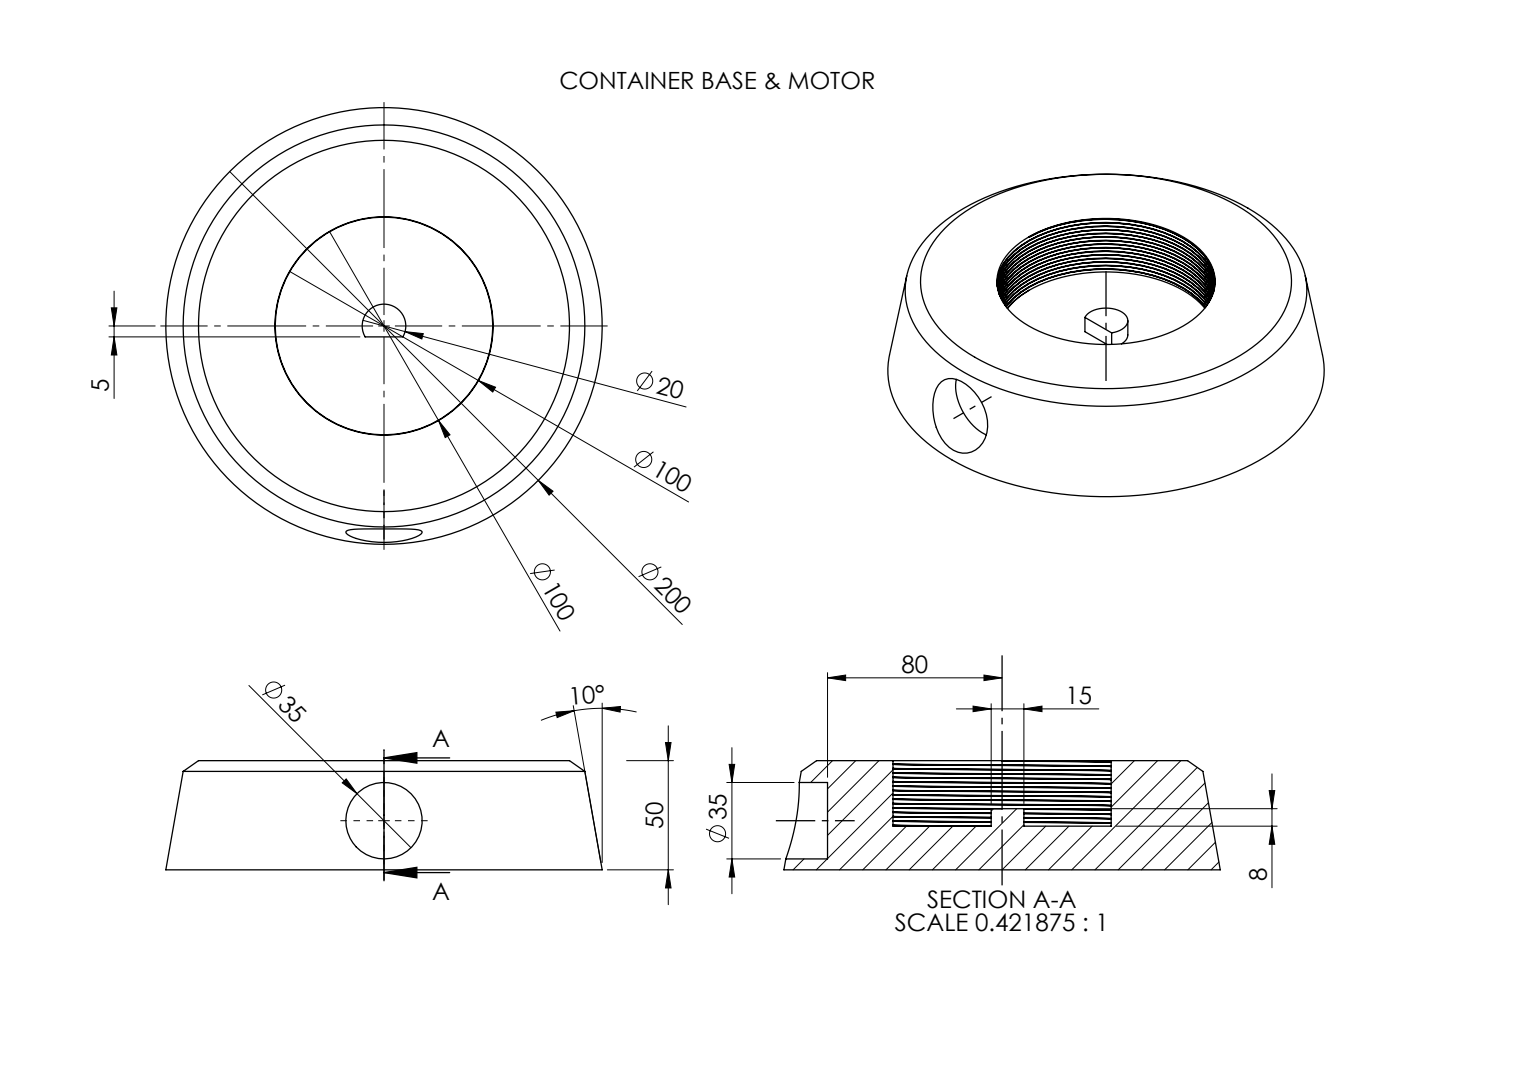
ISO-10303-21;
HEADER;
FILE_DESCRIPTION (('STEP AP214'),
    '1' );
FILE_NAME ('container base & motor.step',
    '2026-10-09T15:02:13',
    ( '' ),
    ( '' ),
    'SwSTEP 2.0',
    'SolidWorks 2026',
    '' );
FILE_SCHEMA (( 'AUTOMOTIVE_DESIGN' ));
ENDSEC;

DATA;
#6=DIRECTION ( 'NONE',  ( 0.000000000000000000, 0.000000000000000000, 1.000000000000000000 ) ) ;
#12=CARTESIAN_POINT ( 'NONE',  ( -15.40903463028480580, 24.25937500034139660, 47.42413220539094709 ) ) ;
#14=CARTESIAN_POINT ( 'NONE',  ( -49.86468353124999453, 37.82187500034139305, -16.20201782572375393 ) ) ;
#16=CARTESIAN_POINT ( 'NONE',  ( -3.219174618344376363E-15, 29.49999999999999645, -52.57311121191334990 ) ) ;
#17=CARTESIAN_POINT ( 'NONE',  ( 30.81806926056962936, 37.15937500034139873, -42.41743335407647209 ) ) ;
#19=CARTESIAN_POINT ( 'NONE',  ( 40.45084971874737079, 45.20000000000000284, -29.38926261462366440 ) ) ;
#27=CARTESIAN_POINT ( 'NONE',  ( -30.90169943749473447, 34.29999999999999005, 42.53254041760200721 ) ) ;
#31=CARTESIAN_POINT ( 'NONE',  ( 15.40903463028482356, 44.52187500034139589, 47.42413220539093999 ) ) ;
#32=CARTESIAN_POINT ( 'NONE',  ( -49.93234176562499727, 49.82031250051209526, 0.000000000000000000 ) ) ;
#34=CARTESIAN_POINT ( 'NONE',  ( -15.45084971874736368, 26.18125000068280173, 47.55282581475768211 ) ) ;
#36=CARTESIAN_POINT ( 'NONE',  ( -3.210462471511496205E-15, 31.42187500034139447, -52.43083105670540789 ) ) ;
#40=VERTEX_POINT ( 'NONE', #9811 ) ;
#45=CARTESIAN_POINT ( 'NONE',  ( -2.547328955960238000E-13, 24.28125000068279604, 49.99999999999999289 ) ) ;
#46=CARTESIAN_POINT ( 'NONE',  ( -3.210462471511496205E-15, 33.35937500034140157, -52.43083105670540789 ) ) ;
#48=CARTESIAN_POINT ( 'NONE',  ( 49.86468353125001585, 46.82187500034139305, 16.20201782572375038 ) ) ;
#63=CARTESIAN_POINT ( 'NONE',  ( 2.600676159226420495E-13, 33.28125000068279604, -49.99999999999999289 ) ) ;
#68=SURFACE_SIDE_STYLE ('',( #9066 ) ) ;
#69=CARTESIAN_POINT ( 'NONE',  ( -7.919222016226809657, 49.55125428154685352, -49.99999999999999289 ) ) ;
#70=CARTESIAN_POINT ( 'NONE',  ( -49.99999999999999289, 39.88125000068279746, 16.24598481164533226 ) ) ;
#73=EDGE_CURVE ( 'NONE', #16417, #15936, #15440, .T. ) ;
#74=CARTESIAN_POINT ( 'NONE',  ( 1.041190247313760726E-14, 50.00000000000000000, 85.01963570546854498 ) ) ;
#78=VECTOR ( 'NONE', #10957, 1000.000000000000000 ) ;
#82=CARTESIAN_POINT ( 'NONE',  ( 0.000000000000000000, 22.50000000000000000, 80.00000000000000000 ) ) ;
#83=CARTESIAN_POINT ( 'NONE',  ( -17.47289750917834539, 23.62647710751876318, 94.22769020256006911 ) ) ;
#89=CARTESIAN_POINT ( 'NONE',  ( 49.86468353125000164, 20.85937500034139802, -6.106662507704105588E-15 ) ) ;
#90=DIRECTION ( 'NONE',  ( -2.126576849575776229E-17, -0.9848077530122080203, -0.1736481776669307198 ) ) ;
#91=CARTESIAN_POINT ( 'NONE',  ( 30.81806926056962936, 27.22187500034139518, -42.41743335407646498 ) ) ;
#94=CARTESIAN_POINT ( 'NONE',  ( 30.90169943749474157, 29.30000000000000071, -42.53254041760200721 ) ) ;
#95=CARTESIAN_POINT ( 'NONE',  ( -49.86468353124999453, 35.95937500034139589, 16.20201782572377525 ) ) ;
#97=CARTESIAN_POINT ( 'NONE',  ( 49.99999999999999289, 41.10000000000000853, -16.24598481164532160 ) ) ;
#100=UNCERTAINTY_MEASURE_WITH_UNIT (LENGTH_MEASURE( 1.000000000000000082E-05 ), #13795, 'distance_accuracy_value', 'NONE');
#102=VERTEX_POINT ( 'NONE', #7719 ) ;
#108=CARTESIAN_POINT ( 'NONE',  ( -40.34137639590981195, 44.12187500034139731, 29.30972558990012189 ) ) ;
#109=CARTESIAN_POINT ( 'NONE',  ( -15.40903463028481646, 39.45937500034139589, -47.42413220539093999 ) ) ;
#113=CARTESIAN_POINT ( 'NONE',  ( -49.99999999999999289, 25.68125000068279462, -16.24598481164531449 ) ) ;
#114=CARTESIAN_POINT ( 'NONE',  ( 15.22000719008740077, 31.21383541804545914, 93.26445288283514401 ) ) ;
#116=CARTESIAN_POINT ( 'NONE',  ( 15.40903463028482356, 32.52187500034139589, 47.42413220539093999 ) ) ;
#122=CARTESIAN_POINT ( 'NONE',  ( -40.45084971874737789, 23.80000000000000071, -29.38926261462365730 ) ) ;
#124=CARTESIAN_POINT ( 'NONE',  ( 9.631387414534489405E-15, 34.35937500034139447, 52.43083105670540789 ) ) ;
#126=FACE_OUTER_BOUND ( 'NONE', #347, .T. ) ;
#128=CARTESIAN_POINT ( 'NONE',  ( 49.86468353125001585, 44.82187500034139305, 16.20201782572375038 ) ) ;
#132=DIRECTION ( 'NONE',  ( 0.000000000000000000, 0.000000000000000000, 1.000000000000000000 ) ) ;
#133=ORIENTED_EDGE ( 'NONE', *, *, #7031, .F. ) ;
#151=CIRCLE ( 'NONE', #2279, 50.00000000000000000 ) ;
#152=CARTESIAN_POINT ( 'NONE',  ( -30.90169943749473447, 32.08125000068280031, 42.53254041760200721 ) ) ;
#156=CARTESIAN_POINT ( 'NONE',  ( -30.90169943749474513, 49.70000000000000284, -42.53254041760200721 ) ) ;
#157=CARTESIAN_POINT ( 'NONE',  ( -40.45084971874737079, 41.98125000068279888, 29.38926261462367151 ) ) ;
#158=DIRECTION ( 'NONE',  ( -0.000000000000000000, 1.000000000000000000, -0.000000000000000000 ) ) ;
#159=EDGE_CURVE ( 'NONE', #15854, #13562, #284, .T. ) ;
#169=CARTESIAN_POINT ( 'NONE',  ( 49.99999999999999289, 42.88125000068279036, -16.24598481164532160 ) ) ;
#170=CARTESIAN_POINT ( 'NONE',  ( -1.240322475938754499E-13, 38.28125000068280315, 50.00000000000000000 ) ) ;
#173=CARTESIAN_POINT ( 'NONE',  ( 2.600676159226421000E-13, 31.49999999999999289, -49.99999999999999289 ) ) ;
#179=CARTESIAN_POINT ( 'NONE',  ( 15.40903463028482356, 24.45937500034139589, 47.42413220539093999 ) ) ;
#181=CARTESIAN_POINT ( 'NONE',  ( 49.86468353125000164, 28.92187500034139802, -6.106662507704105588E-15 ) ) ;
#183=CARTESIAN_POINT ( 'NONE',  ( 15.45084971874737789, 28.60000000000000142, 47.55282581475767500 ) ) ;
#184=CARTESIAN_POINT ( 'NONE',  ( 40.34137639590981905, 32.65937500034139873, 29.30972558990010768 ) ) ;
#192=( BOUNDED_CURVE ( )  B_SPLINE_CURVE ( 2, ( #6981, #12037, #4493, #8380, #732, #13454, #3955, #10196, #11517, #15248, #2623, #11683, #15338 ),
 .UNSPECIFIED., .F., .T. ) 
 B_SPLINE_CURVE_WITH_KNOTS ( ( 3, 2, 2, 2, 2, 2, 3 ),
 ( 0.4500000000000000111, 0.4533333333333333104, 0.4600000000000000200, 0.4666666666666666741, 0.4733333333333333282, 0.4799999999999999822, 0.4833333333333333370 ),
 .UNSPECIFIED. ) 
 CURVE ( )  GEOMETRIC_REPRESENTATION_ITEM ( )  RATIONAL_B_SPLINE_CURVE ( ( 0.9755282581475768211, 0.9755282581475770431, 1.000000000000000000, 0.9510565162951535312, 1.000000000000000000, 0.9510565162951535312, 1.000000000000000000, 0.9510565162951535312, 1.000000000000000000, 0.9510565162951535312, 1.000000000000000000, 0.9755282581475768211, 0.9755282581475768211 ) ) 
 REPRESENTATION_ITEM ( '' )  );
#196=CARTESIAN_POINT ( 'NONE',  ( 15.40903463028481113, 37.32187500034140015, -47.42413220539094709 ) ) ;
#197=CARTESIAN_POINT ( 'NONE',  ( 15.40903463028482356, 44.45937500034139589, 47.42413220539093999 ) ) ;
#198=DIRECTION ( 'NONE',  ( 0.8660254037844513642, 0.4999999999999780731, 0.000000000000000000 ) ) ;
#201=CARTESIAN_POINT ( 'NONE',  ( -15.45084971874736368, 20.18125000068279817, 47.55282581475768211 ) ) ;
#203=CARTESIAN_POINT ( 'NONE',  ( -49.86468353124999453, 28.02187500034139234, 16.20201782572377525 ) ) ;
#211=CARTESIAN_POINT ( 'NONE',  ( 49.99999999999999289, 48.88125000068280457, -16.24598481164532160 ) ) ;
#216=CARTESIAN_POINT ( 'NONE',  ( 49.86468353125000164, 30.85937500034139802, -6.106662507704105588E-15 ) ) ;
#217=CYLINDRICAL_SURFACE ( 'NONE', #11583, 50.00000000000000000 ) ;
#219=CARTESIAN_POINT ( 'NONE',  ( -49.86468353124999453, 47.82187500034140015, -16.20201782572375393 ) ) ;
#222=CARTESIAN_POINT ( 'NONE',  ( -40.34137639590981905, 47.72187500034139873, -29.30972558990011478 ) ) ;
#228=EDGE_LOOP ( 'NONE', ( #7013, #1311, #10553, #6194 ) ) ;
#232=CARTESIAN_POINT ( 'NONE',  ( -40.45084971874737789, 21.80000000000000071, -29.38926261462365730 ) ) ;
#234=CARTESIAN_POINT ( 'NONE',  ( -49.86468353125000164, 49.85937500034139447, 0.000000000000000000 ) ) ;
#237=CARTESIAN_POINT ( 'NONE',  ( -30.81806926056962226, 26.22187500034139518, 42.41743335407647919 ) ) ;
#239=CARTESIAN_POINT ( 'NONE',  ( -50.00000000000000000, 37.78125000068280315, 0.000000000000000000 ) ) ;
#248=DIRECTION ( 'NONE',  ( 0.000000000000000000, 0.000000000000000000, 1.000000000000000000 ) ) ;
#250=ORIENTED_EDGE ( 'NONE', *, *, #6640, .T. ) ;
#253=CARTESIAN_POINT ( 'NONE',  ( -13.94098003074309844, 33.14011566961073640, 93.12075586326798771 ) ) ;
#257=CARTESIAN_POINT ( 'NONE',  ( 40.34137639590981195, 21.05937500034139376, -29.30972558990011834 ) ) ;
#258=CARTESIAN_POINT ( 'NONE',  ( 6.123233995736766085E-15, 20.00000000000000355, -50.00000000000000000 ) ) ;
#259=CARTESIAN_POINT ( 'NONE',  ( 15.40903463028481113, 27.32187500034139660, -47.42413220539094709 ) ) ;
#261=CARTESIAN_POINT ( 'NONE',  ( 50.00000000000000711, 30.89999999999999503, 16.24598481164530739 ) ) ;
#262=CARTESIAN_POINT ( 'NONE',  ( 30.81806926056962936, 29.15937500034139518, -42.41743335407647209 ) ) ;
#275=CARTESIAN_POINT ( 'NONE',  ( -49.86468353124999453, 38.02187500034140299, 16.20201782572377525 ) ) ;
#276=CARTESIAN_POINT ( 'NONE',  ( -49.86468353125000164, 43.85937500034140157, 0.000000000000000000 ) ) ;
#279=CARTESIAN_POINT ( 'NONE',  ( -49.86468353124999453, 49.75937500034138594, -16.20201782572375393 ) ) ;
#280=CARTESIAN_POINT ( 'NONE',  ( 13.91912017332526830, 33.12251588586428852, 93.12580776402357685 ) ) ;
#282=CARTESIAN_POINT ( 'NONE',  ( 15.40903463028481113, 27.32187500034139660, -47.42413220539094709 ) ) ;
#284=( BOUNDED_CURVE ( )  B_SPLINE_CURVE ( 2, ( #4150, #13941, #12709, #1308, #6399, #11460, #5161, #10217, #15270, #3902, #8972, #5486, #15612 ),
 .UNSPECIFIED., .F., .T. ) 
 B_SPLINE_CURVE_WITH_KNOTS ( ( 3, 2, 2, 2, 2, 2, 3 ),
 ( 0.1166666666666666685, 0.1199999999999999956, 0.1266666666666666774, 0.1333333333333333315, 0.1400000000000000133, 0.1466666666666666674, 0.1499999999999999944 ),
 .UNSPECIFIED. ) 
 CURVE ( )  GEOMETRIC_REPRESENTATION_ITEM ( )  RATIONAL_B_SPLINE_CURVE ( ( 0.9755282581475768211, 0.9755282581475768211, 1.000000000000000000, 0.9510565162951535312, 1.000000000000000000, 0.9510565162951535312, 1.000000000000000000, 0.9510565162951535312, 1.000000000000000000, 0.9510565162951535312, 1.000000000000000000, 0.9755282581475768211, 0.9755282581475768211 ) ) 
 REPRESENTATION_ITEM ( '' )  );
#285=CARTESIAN_POINT ( 'NONE',  ( -30.90169943749474513, 27.70000000000000284, -42.53254041760200721 ) ) ;
#288=ORIENTED_EDGE ( 'NONE', *, *, #496, .T. ) ;
#293=CARTESIAN_POINT ( 'NONE',  ( -40.34137639590981195, 28.05937500034139731, 29.30972558990012189 ) ) ;
#294=EDGE_CURVE ( 'NONE', #4877, #10001, #5939, .T. ) ;
#297=CARTESIAN_POINT ( 'NONE',  ( 15.40903463028482356, 40.52187500034139589, 47.42413220539093999 ) ) ;
#300=CARTESIAN_POINT ( 'NONE',  ( 49.86468353125001585, 48.82187500034139305, 16.20201782572375038 ) ) ;
#308=CARTESIAN_POINT ( 'NONE',  ( -40.45084971874737789, 43.58125000068280031, -29.38926261462365730 ) ) ;
#311=CARTESIAN_POINT ( 'NONE',  ( 50.00000000000000711, 24.90000000000000213, 16.24598481164530739 ) ) ;
#312=CARTESIAN_POINT ( 'NONE',  ( 49.86468353125000164, 42.85937500034140157, -6.106662507704105588E-15 ) ) ;
#315=CARTESIAN_POINT ( 'NONE',  ( 49.86468353125000164, 20.92187500034139802, -6.106662507704105588E-15 ) ) ;
#317=DIRECTION ( 'NONE',  ( 0.000000000000000000, 0.000000000000000000, 1.000000000000000000 ) ) ;
#318=CARTESIAN_POINT ( 'NONE',  ( -15.45084971874736368, 42.18125000068279462, 47.55282581475768211 ) ) ;
#334=CARTESIAN_POINT ( 'NONE',  ( 50.00000000000000711, 22.89999999999999858, 16.24598481164530739 ) ) ;
#339=CARTESIAN_POINT ( 'NONE',  ( -48.15826639445383961, 20.00000000000001066, 12.93428853971354009 ) ) ;
#341=CARTESIAN_POINT ( 'NONE',  ( -30.81806926056962226, 26.22187500034139518, 42.41743335407647209 ) ) ;
#344=CARTESIAN_POINT ( 'NONE',  ( 30.81806926056962936, 35.15937500034139873, -42.41743335407647209 ) ) ;
#346=CARTESIAN_POINT ( 'NONE',  ( 40.45084971874737789, 38.80000000000000426, 29.38926261462365375 ) ) ;
#347=EDGE_LOOP ( 'NONE', ( #13905, #11587, #8273, #12260 ) ) ;
#352=DIRECTION ( 'NONE',  ( 0.000000000000000000, 1.000000000000000000, 0.000000000000000000 ) ) ;
#355=CARTESIAN_POINT ( 'NONE',  ( 30.81806926056962936, 33.22187500034139163, -42.41743335407647209 ) ) ;
#356=CARTESIAN_POINT ( 'NONE',  ( 9.631387414534489405E-15, 36.35937500034140157, 52.43083105670540789 ) ) ;
#359=CARTESIAN_POINT ( 'NONE',  ( 49.86468353125000164, 48.85937500034139447, -6.106662507704105588E-15 ) ) ;
#361=CARTESIAN_POINT ( 'NONE',  ( 49.86468353125001585, 30.82187500034139660, 16.20201782572375038 ) ) ;
#362=AXIS2_PLACEMENT_3D ( 'NONE', #15623, #11718, #317 ) ;
#366=ORIENTED_EDGE ( 'NONE', *, *, #16114, .F. ) ;
#369=CARTESIAN_POINT ( 'NONE',  ( -2.547328955960238000E-13, 30.28125000068279604, 49.99999999999999289 ) ) ;
#371=CARTESIAN_POINT ( 'NONE',  ( -40.34137639590981905, 27.65937500034139873, -29.30972558990011478 ) ) ;
#373=VECTOR ( 'NONE', #8711, 1000.000000000000000 ) ;
#374=CARTESIAN_POINT ( 'NONE',  ( 9.631387414534489405E-15, 40.42187500034138736, 52.43083105670540789 ) ) ;
#377=CARTESIAN_POINT ( 'NONE',  ( 15.40903463028481113, 47.32187500034140015, -47.42413220539094709 ) ) ;
#383=VERTEX_POINT ( 'NONE', #15129 ) ;
#384=VERTEX_POINT ( 'NONE', #2495 ) ;
#388=CARTESIAN_POINT ( 'NONE',  ( -8.660254037844387298, 28.00000000000000355, 5.000000000000000000 ) ) ;
#390=CARTESIAN_POINT ( 'NONE',  ( -49.99999999999999289, 26.10000000000000142, 16.24598481164533226 ) ) ;
#391=CARTESIAN_POINT ( 'NONE',  ( 49.86468353125001585, 42.75937500034138594, 16.20201782572375038 ) ) ;
#396=CARTESIAN_POINT ( 'NONE',  ( -40.45084971874737079, 39.98125000068279888, 29.38926261462367151 ) ) ;
#400=CARTESIAN_POINT ( 'NONE',  ( 7.919222016226807881, 46.33250428222964246, 50.00000000000000000 ) ) ;
#405=ORIENTED_EDGE ( 'NONE', *, *, #8129, .F. ) ;
#406=ADVANCED_FACE ( 'NONE', ( #16070 ), #6031, .F. ) ;
#408=CARTESIAN_POINT ( 'NONE',  ( 40.45084971874737079, 43.20000000000000284, -29.38926261462366440 ) ) ;
#410=VECTOR ( 'NONE', #1881, 1000.000000000000000 ) ;
#422=CARTESIAN_POINT ( 'NONE',  ( 1.235979693235591175E-19, 4.999999999999997335, 99.11836509645767990 ) ) ;
#423=CARTESIAN_POINT ( 'NONE',  ( -48.02615145421049903, 20.00000000000000355, 13.41652781627881375 ) ) ;
#424=CARTESIAN_POINT ( 'NONE',  ( -30.81806926056962226, 32.22187500034139163, 42.41743335407647209 ) ) ;
#425=CARTESIAN_POINT ( 'NONE',  ( -2.547328955960238000E-13, 22.49999999999999645, 49.99999999999999289 ) ) ;
#428=CARTESIAN_POINT ( 'NONE',  ( 9.631387414534489405E-15, 32.35937500034139447, 52.43083105670540789 ) ) ;
#430=VECTOR ( 'NONE', #7991, 1000.000000000000000 ) ;
#432=CARTESIAN_POINT ( 'NONE',  ( 49.99999999999999289, 39.10000000000000142, -16.24598481164532160 ) ) ;
#434=( BOUNDED_CURVE ( )  B_SPLINE_CURVE ( 2, ( #3419, #3668, #8482, #2153, #8725, #747, #10898 ),
 .UNSPECIFIED., .F., .F. ) 
 B_SPLINE_CURVE_WITH_KNOTS ( ( 3, 2, 2, 3 ),
 ( 0.9833333333333333925, 0.9866666666666666918, 0.9933333333333332904, 1.000000000000000000 ),
 .UNSPECIFIED. ) 
 CURVE ( )  GEOMETRIC_REPRESENTATION_ITEM ( )  RATIONAL_B_SPLINE_CURVE ( ( 0.9755282581475768211, 0.9755282581475771542, 1.000000000000000000, 0.9510565162951535312, 1.000000000000000000, 0.9510565162951535312, 1.000000000000000000 ) ) 
 REPRESENTATION_ITEM ( '' )  );
#444=CARTESIAN_POINT ( 'NONE',  ( -40.34137639590981905, 37.72187500034139873, -29.30972558990011478 ) ) ;
#445=CARTESIAN_POINT ( 'NONE',  ( -15.40903463028481646, 35.45937500034139589, -47.42413220539093999 ) ) ;
#448=CARTESIAN_POINT ( 'NONE',  ( -15.40903463028481646, 49.45937500034140299, -47.42413220539093999 ) ) ;
#450=CARTESIAN_POINT ( 'NONE',  ( -3.210462471511496205E-15, 25.42187500034139092, -52.43083105670540789 ) ) ;
#452=CARTESIAN_POINT ( 'NONE',  ( -40.45084971874737789, 27.58125000068280031, -29.38926261462365730 ) ) ;
#458=CARTESIAN_POINT ( 'NONE',  ( -40.45084971874737079, 33.98125000068279888, 29.38926261462367151 ) ) ;
#461=CARTESIAN_POINT ( 'NONE',  ( -49.86468353124999453, 27.95937500034139944, 16.20201782572377525 ) ) ;
#463=CARTESIAN_POINT ( 'NONE',  ( -49.86468353124999453, 41.82187500034140015, -16.20201782572375393 ) ) ;
#465=CARTESIAN_POINT ( 'NONE',  ( 30.81806926056964002, 46.62187500034140442, 42.41743335407647209 ) ) ;
#470=ORIENTED_EDGE ( 'NONE', *, *, #10226, .T. ) ;
#472=CARTESIAN_POINT ( 'NONE',  ( 0.000000000000000000, 22.50000000000000000, 80.00000000000000000 ) ) ;
#475=CARTESIAN_POINT ( 'NONE',  ( 9.657523855033129090E-15, 24.50000000000000355, 52.57311121191334990 ) ) ;
#476=CARTESIAN_POINT ( 'NONE',  ( -3.210462471511496205E-15, 47.35937500034138736, -52.43083105670540789 ) ) ;
#482=LINE ( 'NONE', #8144, #13108 ) ;
#483=CARTESIAN_POINT ( 'NONE',  ( -15.45084971874736368, 32.18125000068279462, 47.55282581475768211 ) ) ;
#496=EDGE_CURVE ( 'NONE', #9157, #8721, #11184, .T. ) ;
#498=CARTESIAN_POINT ( 'NONE',  ( 40.45084971874737079, 23.20000000000000284, -29.38926261462366440 ) ) ;
#501=CARTESIAN_POINT ( 'NONE',  ( -30.90169943749473447, 30.08125000068279675, 42.53254041760200721 ) ) ;
#503=ADVANCED_FACE ( 'NONE', ( #9598 ), #12925, .T. ) ;
#504=CARTESIAN_POINT ( 'NONE',  ( -47.65000835890729292, 20.00000000000000355, 14.69569212619059684 ) ) ;
#505=CARTESIAN_POINT ( 'NONE',  ( 30.81806926056962936, 23.22187500034139163, -42.41743335407646498 ) ) ;
#510=CARTESIAN_POINT ( 'NONE',  ( 40.34137639590981905, 34.65937500034139873, 29.30972558990010768 ) ) ;
#519=VECTOR ( 'NONE', #4561, 1000.000000000000000 ) ;
#522=CARTESIAN_POINT ( 'NONE',  ( -49.86468353125000164, 37.92187500034140157, 0.000000000000000000 ) ) ;
#523=CARTESIAN_POINT ( 'NONE',  ( -30.81806926056963292, 37.55937500034139020, -42.41743335407646498 ) ) ;
#526=CARTESIAN_POINT ( 'NONE',  ( 15.45084971874736723, 23.18125000068279817, -47.55282581475768211 ) ) ;
#528=( BOUNDED_CURVE ( )  B_SPLINE_CURVE ( 2, ( #2578, #6411, #11472, #156, #11398, #69, #5174 ),
 .UNSPECIFIED., .F., .F. ) 
 B_SPLINE_CURVE_WITH_KNOTS ( ( 3, 2, 2, 3 ),
 ( 0.000000000000000000, 0.006666666666666667095, 0.01333333333333333419, 0.01666666666666666990 ),
 .UNSPECIFIED. ) 
 CURVE ( )  GEOMETRIC_REPRESENTATION_ITEM ( )  RATIONAL_B_SPLINE_CURVE ( ( 1.000000000000000000, 0.9510565162951535312, 1.000000000000000000, 0.9510565162951535312, 1.000000000000000000, 0.9755282581475768211, 0.9755282581475768211 ) ) 
 REPRESENTATION_ITEM ( '' )  );
#530=CARTESIAN_POINT ( 'NONE',  ( 49.86468353125000164, 26.92187500034139802, -6.106662507704105588E-15 ) ) ;
#535=ORIENTED_EDGE ( 'NONE', *, *, #3544, .T. ) ;
#539=CARTESIAN_POINT ( 'NONE',  ( -40.34137639590981195, 26.05937500034139731, 29.30972558990012189 ) ) ;
#541=CARTESIAN_POINT ( 'NONE',  ( -30.81806926056963292, 39.62187500034139020, -42.41743335407646498 ) ) ;
#543=CARTESIAN_POINT ( 'NONE',  ( -3.210462471511496205E-15, 49.42187500034138736, -52.43083105670540789 ) ) ;
#547=PRODUCT_DEFINITION_SHAPE ( 'NONE', 'NONE',  #11888 ) ;
#551=LINE ( 'NONE', #10709, #923 ) ;
#552=DIRECTION ( 'NONE',  ( 0.000000000000000000, -1.000000000000000000, 0.000000000000000000 ) ) ;
#553=CARTESIAN_POINT ( 'NONE',  ( -40.45084971874737789, 25.80000000000000071, -29.38926261462365730 ) ) ;
#554=CARTESIAN_POINT ( 'NONE',  ( -40.34137639590981905, 45.65937500034139873, -29.30972558990011478 ) ) ;
#555=CARTESIAN_POINT ( 'NONE',  ( -30.81806926056963292, 47.55937500034139731, -42.41743335407646498 ) ) ;
#556=CARTESIAN_POINT ( 'NONE',  ( -2.547328955960238000E-13, 32.28125000068278894, 49.99999999999999289 ) ) ;
#560=CARTESIAN_POINT ( 'NONE',  ( 40.45084971874737789, 22.58125000068279675, 29.38926261462365375 ) ) ;
#564=EDGE_CURVE ( 'NONE', #10216, #11191, #8756, .T. ) ;
#567=EDGE_LOOP ( 'NONE', ( #8568, #5125, #571, #2717, #7157 ) ) ;
#568=CARTESIAN_POINT ( 'NONE',  ( 0.000000000000000000, 20.00000000000000355, 0.000000000000000000 ) ) ;
#571=ORIENTED_EDGE ( 'NONE', *, *, #12236, .F. ) ;
#572=LINE ( 'NONE', #1986, #430 ) ;
#578=CARTESIAN_POINT ( 'NONE',  ( 13.94233552421758837, 11.90832207049870206, 96.90308138387069903 ) ) ;
#580=CARTESIAN_POINT ( 'NONE',  ( -40.34137639590981195, 22.12187500034139731, 29.30972558990012189 ) ) ;
#583=CARTESIAN_POINT ( 'NONE',  ( 49.86468353125001585, 28.75937500034139305, 16.20201782572375038 ) ) ;
#591=CARTESIAN_POINT ( 'NONE',  ( 0.000000000000000000, 20.00000000000000355, 0.000000000000000000 ) ) ;
#595=CARTESIAN_POINT ( 'NONE',  ( -49.86468353125000164, 29.92187500034139802, 0.000000000000000000 ) ) ;
#596=CARTESIAN_POINT ( 'NONE',  ( -49.86468353125000164, 37.85937500034139447, 0.000000000000000000 ) ) ;
#601=CARTESIAN_POINT ( 'NONE',  ( -3.210462471511496205E-15, 47.35937500034138736, -52.43083105670540789 ) ) ;
#604=CARTESIAN_POINT ( 'NONE',  ( -15.40903463028481646, 23.52187500034139944, -47.42413220539093999 ) ) ;
#607=CARTESIAN_POINT ( 'NONE',  ( -15.45084971874736368, 28.18125000068279817, 47.55282581475768211 ) ) ;
#608=ORIENTED_EDGE ( 'NONE', *, *, #2441, .T. ) ;
#610=CIRCLE ( 'NONE', #11775, 50.00000000000000000 ) ;
#612=CARTESIAN_POINT ( 'NONE',  ( -5.823736356558309156E-14, 44.28125000068280315, 50.00000000000000000 ) ) ;
#615=CARTESIAN_POINT ( 'NONE',  ( 49.86468353125000164, 20.85937500034139802, -6.106662507704105588E-15 ) ) ;
#617=( BOUNDED_CURVE ( )  B_SPLINE_CURVE ( 2, ( #7741, #2667, #10000, #7663, #1411, #169, #5273, #15383, #8818, #9075, #12734, #16306, #7495 ),
 .UNSPECIFIED., .F., .F. ) 
 B_SPLINE_CURVE_WITH_KNOTS ( ( 3, 2, 2, 2, 2, 2, 3 ),
 ( 0.2166666666666666741, 0.2200000000000000011, 0.2266666666666666552, 0.2333333333333333370, 0.2399999999999999911, 0.2466666666666666730, 0.2500000000000000000 ),
 .UNSPECIFIED. ) 
 CURVE ( )  GEOMETRIC_REPRESENTATION_ITEM ( )  RATIONAL_B_SPLINE_CURVE ( ( 0.9755282581475768211, 0.9755282581475768211, 1.000000000000000000, 0.9510565162951535312, 1.000000000000000000, 0.9510565162951535312, 1.000000000000000000, 0.9510565162951535312, 1.000000000000000000, 0.9510565162951535312, 1.000000000000000000, 0.9755282581475768211, 0.9755282581475765991 ) ) 
 REPRESENTATION_ITEM ( '' )  );
#618=CARTESIAN_POINT ( 'NONE',  ( 50.00000000000000000, 39.00000000000000000, -6.123233995736766085E-15 ) ) ;
#620=CARTESIAN_POINT ( 'NONE',  ( 15.40903463028482356, 42.52187500034139589, 47.42413220539093999 ) ) ;
#627=CARTESIAN_POINT ( 'NONE',  ( -3.111920190527341144E-15, 45.50000000000000000, -50.00000000000000000 ) ) ;
#632=CARTESIAN_POINT ( 'NONE',  ( -50.00000000000000000, 20.00000000000000000, 0.000000000000000000 ) ) ;
#633=CARTESIAN_POINT ( 'NONE',  ( 15.40903463028481113, 43.25937500034139305, -47.42413220539094709 ) ) ;
#634=CARTESIAN_POINT ( 'NONE',  ( 40.34137639590981195, 47.05937500034140442, -29.30972558990011834 ) ) ;
#635=CARTESIAN_POINT ( 'NONE',  ( 7.919222016226809657, 25.44874571845315359, -50.00000000000000000 ) ) ;
#638=CARTESIAN_POINT ( 'NONE',  ( -15.45084971874736368, 46.40000000000000568, 47.55282581475768211 ) ) ;
#639=CARTESIAN_POINT ( 'NONE',  ( 15.45084971874737789, 20.38125000068279746, 47.55282581475767500 ) ) ;
#640=CARTESIAN_POINT ( 'NONE',  ( -17.50000000000000000, 22.50000000000000000, 80.00000000000000000 ) ) ;
#654=CYLINDRICAL_SURFACE ( 'NONE', #8851, 50.00000000000000000 ) ;
#658=CARTESIAN_POINT ( 'NONE',  ( -40.45084971874737079, 32.20000000000000284, 29.38926261462367151 ) ) ;
#659=ADVANCED_FACE ( 'NONE', ( #13818 ), #1344, .F. ) ;
#663=CARTESIAN_POINT ( 'NONE',  ( 49.86468353124999453, 23.02187500034139944, -16.20201782572376104 ) ) ;
#666=CARTESIAN_POINT ( 'NONE',  ( 40.34137639590981195, 29.05937500034139376, -29.30972558990011834 ) ) ;
#678=CARTESIAN_POINT ( 'NONE',  ( 49.86468353125001585, 26.82187500034138949, 16.20201782572375038 ) ) ;
#679=CARTESIAN_POINT ( 'NONE',  ( -49.86468353124999453, 33.95937500034139589, 16.20201782572377169 ) ) ;
#687=CARTESIAN_POINT ( 'NONE',  ( -49.86468353124999453, 45.75937500034140015, -16.20201782572375393 ) ) ;
#689=( BOUNDED_CURVE ( )  B_SPLINE_CURVE ( 2, ( #16294, #2487, #7565, #8893, #2576, #11470, #15284, #2732, #3913, #1400, #7810, #4068, #13209 ),
 .UNSPECIFIED., .F., .T. ) 
 B_SPLINE_CURVE_WITH_KNOTS ( ( 3, 2, 2, 2, 2, 2, 3 ),
 ( 0.8166666666666666519, 0.8199999999999999512, 0.8266666666666666607, 0.8333333333333333703, 0.8399999999999999689, 0.8466666666666666785, 0.8500000000000000888 ),
 .UNSPECIFIED. ) 
 CURVE ( )  GEOMETRIC_REPRESENTATION_ITEM ( )  RATIONAL_B_SPLINE_CURVE ( ( 0.9755282581475768211, 0.9755282581475768211, 1.000000000000000000, 0.9510565162951535312, 1.000000000000000000, 0.9510565162951535312, 1.000000000000000000, 0.9510565162951535312, 1.000000000000000000, 0.9510565162951535312, 1.000000000000000000, 0.9755282581475763770, 0.9755282581475768211 ) ) 
 REPRESENTATION_ITEM ( '' )  );
#690=CARTESIAN_POINT ( 'NONE',  ( 40.34137639590981905, 22.72187500034139518, 29.30972558990010768 ) ) ;
#695=EDGE_LOOP ( 'NONE', ( #7195, #10121, #1457 ) ) ;
#704=CARTESIAN_POINT ( 'NONE',  ( 9.631387414534489405E-15, 46.42187500034139447, 52.43083105670540789 ) ) ;
#708=CARTESIAN_POINT ( 'NONE',  ( 15.45084971874737789, 40.60000000000000142, 47.55282581475767500 ) ) ;
#712=CARTESIAN_POINT ( 'NONE',  ( -30.81806926056962226, 42.22187500034139163, 42.41743335407647919 ) ) ;
#720=FACE_OUTER_BOUND ( 'NONE', #12786, .T. ) ;
#725=CARTESIAN_POINT ( 'NONE',  ( 1.293669679204937499E-13, 37.50000000000000711, -50.00000000000000000 ) ) ;
#726=CARTESIAN_POINT ( 'NONE',  ( 49.86468353125000164, 36.85937500034139447, -6.106662507704105588E-15 ) ) ;
#727=CARTESIAN_POINT ( 'NONE',  ( -49.86468353124999453, 45.95937500034138878, 16.20201782572377169 ) ) ;
#732=CARTESIAN_POINT ( 'NONE',  ( -40.45084971874737079, 35.98125000068279888, 29.38926261462367151 ) ) ;
#735=DIRECTION ( 'NONE',  ( 0.000000000000000000, 0.000000000000000000, 1.000000000000000000 ) ) ;
#738=ORIENTED_EDGE ( 'NONE', *, *, #13518, .F. ) ;
#743=CARTESIAN_POINT ( 'NONE',  ( 15.45084971874736723, 29.40000000000000213, -47.55282581475768211 ) ) ;
#745=CARTESIAN_POINT ( 'NONE',  ( 1.293669679204937499E-13, 37.50000000000000711, -50.00000000000000000 ) ) ;
#747=CARTESIAN_POINT ( 'NONE',  ( -49.99999999999999289, 20.09999999999999787, 16.24598481164533226 ) ) ;
#749=DIRECTION ( 'NONE',  ( 0.000000000000000000, -0.000000000000000000, 1.000000000000000000 ) ) ;
#752=CARTESIAN_POINT ( 'NONE',  ( -43.39327851764683430, 20.00000000000000711, 25.00490296284258918 ) ) ;
#753=CARTESIAN_POINT ( 'NONE',  ( -15.40903463028480580, 20.32187500034139660, 47.42413220539094709 ) ) ;
#755=CARTESIAN_POINT ( 'NONE',  ( -15.40903463028481646, 23.45937500034139944, -47.42413220539093999 ) ) ;
#762=CARTESIAN_POINT ( 'NONE',  ( 40.45084971874737789, 48.80000000000000426, 29.38926261462365375 ) ) ;
#764=CARTESIAN_POINT ( 'NONE',  ( 50.00000000000000711, 48.68125000068279462, 16.24598481164530739 ) ) ;
#767=CARTESIAN_POINT ( 'NONE',  ( -49.86468353124999453, 29.82187500034139660, -16.20201782572375393 ) ) ;
#768=CARTESIAN_POINT ( 'NONE',  ( 30.81806926056964002, 32.55937500034139731, 42.41743335407646498 ) ) ;
#772=CARTESIAN_POINT ( 'NONE',  ( 9.631387414534489405E-15, 46.35937500034139447, 52.43083105670540789 ) ) ;
#774=CARTESIAN_POINT ( 'NONE',  ( 9.631387414534489405E-15, 22.42187500034139802, 52.43083105670540789 ) ) ;
#780=ORIENTED_EDGE ( 'NONE', *, *, #7914, .F. ) ;
#781=CARTESIAN_POINT ( 'NONE',  ( -7.919222016226688865, 33.33250428222964956, -50.00000000000003553 ) ) ;
#783=CARTESIAN_POINT ( 'NONE',  ( -49.86468353124999453, 19.95937500034138878, 16.20201782572377525 ) ) ;
#787=EDGE_CURVE ( 'NONE', #4002, #5069, #14947, .T. ) ;
#788=PRODUCT_CONTEXT ( 'NONE', #6541, 'mechanical' ) ;
#789=CARTESIAN_POINT ( 'NONE',  ( -40.45084971874737079, 31.98125000068280244, 29.38926261462367151 ) ) ;
#790=CARTESIAN_POINT ( 'NONE',  ( -50.00000000000000000, 36.00000000000000711, 0.000000000000000000 ) ) ;
#791=CARTESIAN_POINT ( 'NONE',  ( 15.40903463028481113, 43.32187500034139305, -47.42413220539094709 ) ) ;
#796=DIRECTION ( 'NONE',  ( -1.000000000000000000, 0.000000000000000000, -0.000000000000000000 ) ) ;
#803=CARTESIAN_POINT ( 'NONE',  ( -2.547328955960238000E-13, 22.28125000068279604, 49.99999999999999289 ) ) ;
#804=CARTESIAN_POINT ( 'NONE',  ( 49.99999999999999289, 36.88125000068279036, -16.24598481164532160 ) ) ;
#805=CARTESIAN_POINT ( 'NONE',  ( -30.81806926056962226, 38.15937500034138452, 42.41743335407647919 ) ) ;
#806=CARTESIAN_POINT ( 'NONE',  ( -40.34137639590981905, 45.65937500034139873, -29.30972558990011478 ) ) ;
#817=EDGE_LOOP ( 'NONE', ( #2895, #1858, #470, #5587, #7961 ) ) ;
#820=( BOUNDED_CURVE ( )  B_SPLINE_CURVE ( 2, ( #15392, #6687, #13234, #3087, #10333, #5524, #4346, #4266, #15642, #14383, #1832, #13070, #9332 ),
 .UNSPECIFIED., .F., .F. ) 
 B_SPLINE_CURVE_WITH_KNOTS ( ( 3, 2, 2, 2, 2, 2, 3 ),
 ( 0.3833333333333333592, 0.3866666666666666585, 0.3933333333333333126, 0.4000000000000000222, 0.4066666666666666763, 0.4133333333333333304, 0.4166666666666666852 ),
 .UNSPECIFIED. ) 
 CURVE ( )  GEOMETRIC_REPRESENTATION_ITEM ( )  RATIONAL_B_SPLINE_CURVE ( ( 0.9755282581475768211, 0.9755282581475770431, 1.000000000000000000, 0.9510565162951535312, 1.000000000000000000, 0.9510565162951535312, 1.000000000000000000, 0.9510565162951535312, 1.000000000000000000, 0.9510565162951535312, 1.000000000000000000, 0.9755282581475765991, 0.9755282581475768211 ) ) 
 REPRESENTATION_ITEM ( '' )  );
#822=CARTESIAN_POINT ( 'NONE',  ( -15.45084971874737256, 39.60000000000000142, -47.55282581475767500 ) ) ;
#823=CARTESIAN_POINT ( 'NONE',  ( 6.123233995736766085E-15, 20.00000000000000355, -50.00000000000000000 ) ) ;
#825=LINE ( 'NONE', #16289, #14432 ) ;
#829=CARTESIAN_POINT ( 'NONE',  ( -49.93234176562499727, 49.96093750017070079, 0.000000000000000000 ) ) ;
#831=CARTESIAN_POINT ( 'NONE',  ( -30.90169943749474513, 47.70000000000000284, -42.53254041760200721 ) ) ;
#834=CARTESIAN_POINT ( 'NONE',  ( -45.40153297753673201, 20.00000000000001776, 20.62078143446483480 ) ) ;
#835=CARTESIAN_POINT ( 'NONE',  ( 49.86468353125000164, 24.92187500034139802, -6.106662507704105588E-15 ) ) ;
#838=CARTESIAN_POINT ( 'NONE',  ( -49.86468353124999453, 27.95937500034139944, 16.20201782572377525 ) ) ;
#841=CARTESIAN_POINT ( 'NONE',  ( 30.90169943749475223, 44.69999999999999574, 42.53254041760199300 ) ) ;
#842=VERTEX_POINT ( 'NONE', #9257 ) ;
#849=CARTESIAN_POINT ( 'NONE',  ( -15.40903463028480580, 32.32187500034139305, 47.42413220539094709 ) ) ;
#850=CARTESIAN_POINT ( 'NONE',  ( 40.34137639590981905, 30.65937500034139518, 29.30972558990010768 ) ) ;
#854=CARTESIAN_POINT ( 'NONE',  ( 49.86468353125001585, 46.75937500034140015, 16.20201782572375038 ) ) ;
#857=CARTESIAN_POINT ( 'NONE',  ( 15.40903463028482356, 24.52187500034139589, 47.42413220539093999 ) ) ;
#864=CARTESIAN_POINT ( 'NONE',  ( -40.34137639590981905, 21.65937500034139518, -29.30972558990011478 ) ) ;
#868=CARTESIAN_POINT ( 'NONE',  ( -49.99999999999999289, 31.88125000068280102, 16.24598481164533226 ) ) ;
#869=CARTESIAN_POINT ( 'NONE',  ( 40.34137639590981195, 41.12187500034139731, -29.30972558990011834 ) ) ;
#876=ORIENTED_EDGE ( 'NONE', *, *, #11887, .F. ) ;
#880=CARTESIAN_POINT ( 'NONE',  ( -15.45084971874737256, 49.38125000068280457, -47.55282581475767500 ) ) ;
#882=CARTESIAN_POINT ( 'NONE',  ( -49.86468353124999453, 35.75937500034140015, -16.20201782572375393 ) ) ;
#883=CARTESIAN_POINT ( 'NONE',  ( -3.210462471511496205E-15, 49.35937500034138736, -52.43083105670540789 ) ) ;
#884=CARTESIAN_POINT ( 'NONE',  ( 50.00000000000000711, 24.89999999999999858, 16.24598481164530739 ) ) ;
#885=CIRCLE ( 'NONE', #362, 10.00000000000000000 ) ;
#886=CARTESIAN_POINT ( 'NONE',  ( -2.547328955960238000E-13, 30.49999999999999645, 49.99999999999999289 ) ) ;
#898=FACE_OUTER_BOUND ( 'NONE', #2362, .T. ) ;
#901=CARTESIAN_POINT ( 'NONE',  ( 2.978552182361884590E-14, 47.28125000068279604, -50.00000000000000000 ) ) ;
#903=CARTESIAN_POINT ( 'NONE',  ( -16.94192497067215797, 17.96950525308796287, 95.33822655640803134 ) ) ;
#904=CARTESIAN_POINT ( 'NONE',  ( 2.600676159226421000E-13, 21.28125000068279604, -49.99999999999999289 ) ) ;
#905=CARTESIAN_POINT ( 'NONE',  ( -2.445080149700054274E-14, 46.28125000068280315, 50.00000000000000000 ) ) ;
#906=CARTESIAN_POINT ( 'NONE',  ( 8.660254037844387298, 28.00000000000000355, 5.000000000000000000 ) ) ;
#910=CARTESIAN_POINT ( 'NONE',  ( -50.00000000000000000, 47.78125000068279604, 0.000000000000000000 ) ) ;
#913=CARTESIAN_POINT ( 'NONE',  ( -40.34137639590981195, 28.05937500034139731, 29.30972558990012189 ) ) ;
#923=VECTOR ( 'NONE', #11786, 1000.000000000000000 ) ;
#928=CARTESIAN_POINT ( 'NONE',  ( -49.86468353124999453, 27.82187500034139305, -16.20201782572375393 ) ) ;
#929=CARTESIAN_POINT ( 'NONE',  ( -30.81806926056962226, 32.15937500034139873, 42.41743335407647209 ) ) ;
#933=CARTESIAN_POINT ( 'NONE',  ( 49.86468353125000164, 44.85937500034140157, -6.106662507704105588E-15 ) ) ;
#936=CARTESIAN_POINT ( 'NONE',  ( -3.219174618344376363E-15, 49.50000000000000711, -52.57311121191334990 ) ) ;
#939=ORIENTED_EDGE ( 'NONE', *, *, #11943, .F. ) ;
#942=AXIS2_PLACEMENT_3D ( 'NONE', #9406, #9328, #14453 ) ;
#943=AXIS2_PLACEMENT_3D ( 'NONE', #6427, #11487, #8999 ) ;
#946=CARTESIAN_POINT ( 'NONE',  ( -49.86468353125000164, 19.85937500034139447, 0.000000000000000000 ) ) ;
#950=CARTESIAN_POINT ( 'NONE',  ( -30.90169943749474868, 31.48125000068279533, -42.53254041760200721 ) ) ;
#951=CARTESIAN_POINT ( 'NONE',  ( 49.86468353125001585, 40.82187500034140726, 16.20201782572375038 ) ) ;
#955=ORIENTED_EDGE ( 'NONE', *, *, #11085, .F. ) ;
#961=( BOUNDED_SURFACE ( )  B_SPLINE_SURFACE ( 1, 2, ( 
 ( #234, #12794, #13868, #2484, #5340, #1397, #10392, #3910, #11311, #9138, #15448, #12634, #5013, #4066, #6488, #1236, #15368, #11544, #13949, #14197, #3989, #9061, #12550, #3743, #6330, #476, #15528, #2818, #10640, #9468, #13207, #14520, #7891, #6826, #13121, #4243, #2979, #3143, #5647, #8049, #13045, #1571, #554, #9385, #12966, #13283, #5579, #15617, #11791, #10564, #8136, #10713, #1886, #9309, #11878, #9552, #6977, #10803, #8217, #15692, #5496, #12031, #15773, #15865, #4399, #14435, #633, #6663, #5728, #1728, #312, #391, #4487, #14283, #11956, #11713, #5412, #10470, #4158, #4320, #9230, #2906, #7973, #1647, #14362, #6744, #3058, #1811, #6903, #7307, #1963, #9801, #8463, #8373, #10879, #16021, #13605, #13686, #8294, #9879, #14930, #2210, #12366, #3560, #8613, #2303, #5893, #15941, #968, #11042, #6065, #7391, #13529, #16196, #13446, #13362, #14852, #805, #5810, #9714, #3397, #3222, #16111, #12455, #4824, #2131, #7056, #12120, #11134, #1048, #726, #6143, #7220, #12280, #4744, #2056, #4563, #11215, #16270, #9626, #3480, #882, #5976, #14766, #8535, #14678, #4901, #14599, #3306, #7144, #12203, #10956, #4649, #2633, #9041, #124, #7709, #13771, #6389, #12778, #5239, #1379, #15349, #1212, #10295, #46, #8706, #16352, #6469, #2383, #5150, #3806, #3728, #6221, #11377, #8960, #14096, #3650, #3966, #2710, #14014, #11526, #7790, #12859, #1464, #6308, #11291, #6558, #11452, #11618, #216, #8870, #9959, #8787, #7466, #10207, #12614, #1126, #5074, #15177, #15015, #15259, #12533, #4991, #13931, #10047, #15101, #13849, #2463, #7544, #16440, #2550, #7629, #3888, #10127, #12699, #1298, #1867, #293, #461, #8030, #13104, #371, #10544, #14178, #14418, #5563, #8110, #10624, #10697, #11858, #15428, #2962, #1552, #5319, #1709, #11938, #15678, #539, #10370, #9290, #15602, #6722, #5474, #5633, #13190, #4223, #15507, #4048, #3038, #4304, #9118, #15753, #6806, #1628, #14264, #13026, #9368, #1794, #4381, #11771, #14346, #12016, #9446, #13268, #14500, #6887, #7954, #3129, #8201, #6963, #2795, #7870, #12948, #6645, #11694, #5392, #10451, #4134, #9209, #2885, #9785, #864, #3459, #12263, #6045, #7200, #10779, #14742, #13344, #615, #8443, #7289, #11021, #12345, #5711, #4628, #10937, #2035, #783, #946 ),
 ( #13425, #9611, #8356, #5960, #8520, #11117, #7126, #9690, #7374, #4807, #8595, #16178, #3377, #3287, #9859, #14830, #13668, #13585, #16089, #2192, #4469, #14911, #5875, #14580, #14659, #3541, #12097, #2282, #15845, #9536, #3206, #8278, #13506, #1947, #7040, #704, #5792, #12184, #10859, #4724, #15925, #4547, #16002, #2113, #7612, #6290, #6204, #8688, #13832, #11438, #11512, #6128, #7693, #12763, #31, #5136, #1362, #6453, #108, #3712, #13754, #10191, #8854, #3868, #5215, #11359, #14000, #11275, #11197, #12686, #15085, #3629, #7523, #1190, #1030, #13912, #10275, #2618, #16424, #16250, #4885, #15244, #8942, #9941, #15331, #5060, #10111, #2531, #16333, #14995, #3950, #9024, #7450, #1283, #15162, #8770, #4973, #2446, #6372, #14079, #2694, #12596, #3789, #12437, #2367, #12517, #1107, #10032, #10434, #11922, #5545, #15732, #15663, #14328, #4285, #11599, #6871, #13008, #5302, #275, #522, #2777, #444, #5617, #14399, #10607, #196, #4207, #9349, #3022, #8093, #13168, #15490, #1777, #2945, #6533, #14161, #10680, #10351, #8012, #1611, #1535, #4031, #9184, #6789, #4363, #1445, #9428, #14476, #11833, #7770, #12842, #15413, #9101, #4115, #7850, #12930, #9273, #6624, #11677, #6704, #5379, #14248, #2867, #13086, #7935, #11754, #355, #5455, #10520, #1692, #15582, #9765, #13401, #1849, #8183, #849, #7185, #6945, #14812, #12165, #7110, #4609, #1927, #13249, #4699, #16158, #14564, #14722, #5857, #10921, #14641, #8339, #11999, #12246, #3353, #5941, #8427, #8505, #9672, #595, #767, #15818, #3111, #15983, #3443, #13489, #13570, #5690, #2097, #2013, #4531, #3269, #2174, #11004, #16066, #13325, #10758, #7270, #12326, #4452, #928, #6026, #11098, #4789, #9845, #9517, #3188, #8261, #7020, #12074, #678, #5777, #10843, #15907, #9594, #8576, #237, #11716, #9925, #10093, #1172, #6267, #10010, #3695, #7355, #7811, #15141, #1493, #3769, #4070, #5038, #13651, #12574, #11181, #14897, #11338, #5343, #8828, #10395, #3524, #2426, #8751, #16316, #15066, #15451, #6585, #13814, #8668, #2259, #12882, #13891, #12422, #9142, #16405, #11258, #7432, #6184, #2507, #11642, #14200, #4951, #7503, #5415, #2824, #6666, #7894, #12969, #1092, #1574, #315, #1013, #6110, #16235, #4869, #14979, #3608, #13737, #2350, #12499, #3225 ) ),
 .UNSPECIFIED., .F., .F., .F. ) 
 B_SPLINE_SURFACE_WITH_KNOTS ( ( 2, 2 ),
 ( 3, 2, 2, 2, 2, 2, 2, 2, 2, 2, 2, 2, 2, 2, 2, 2, 2, 2, 2, 2, 2, 2, 2, 2, 2, 2, 2, 2, 2, 2, 2, 2, 2, 2, 2, 2, 2, 2, 2, 2, 2, 2, 2, 2, 2, 2, 2, 2, 2, 2, 2, 2, 2, 2, 2, 2, 2, 2, 2, 2, 2, 2, 2, 2, 2, 2, 2, 2, 2, 2, 2, 2, 2, 2, 2, 2, 2, 2, 2, 2, 2, 2, 2, 2, 2, 2, 2, 2, 2, 2, 2, 2, 2, 2, 2, 2, 2, 2, 2, 2, 2, 2, 2, 2, 2, 2, 2, 2, 2, 2, 2, 2, 2, 2, 2, 2, 2, 2, 2, 2, 2, 2, 2, 2, 2, 2, 2, 2, 2, 2, 2, 2, 2, 2, 2, 2, 2, 2, 2, 2, 2, 2, 2, 2, 2, 2, 2, 2, 2, 2, 3 ),
 ( 0.000000000000000000, 1.000000000000000000 ),
 ( 0.000000000000000000, 0.006666666666666667095, 0.01333333333333333419, 0.02000000000000000042, 0.02666666666666666838, 0.03333333333333333287, 0.04000000000000000083, 0.04666666666666666879, 0.05333333333333333676, 0.05999999999999999778, 0.06666666666666666574, 0.07333333333333333370, 0.08000000000000000167, 0.08666666666666666963, 0.09333333333333333759, 0.1000000000000000056, 0.1066666666666666735, 0.1133333333333333276, 0.1199999999999999956, 0.1266666666666666774, 0.1333333333333333315, 0.1400000000000000133, 0.1466666666666666674, 0.1533333333333333215, 0.1600000000000000033, 0.1666666666666666574, 0.1733333333333333393, 0.1799999999999999933, 0.1866666666666666752, 0.1933333333333333293, 0.2000000000000000111, 0.2066666666666666652, 0.2133333333333333470, 0.2200000000000000011, 0.2266666666666666552, 0.2333333333333333370, 0.2399999999999999911, 0.2466666666666666730, 0.2533333333333333548, 0.2600000000000000089, 0.2666666666666666630, 0.2733333333333333171, 0.2800000000000000266, 0.2866666666666666807, 0.2933333333333333348, 0.2999999999999999889, 0.3066666666666666430, 0.3133333333333333526, 0.3200000000000000067, 0.3266666666666666607, 0.3333333333333333148, 0.3400000000000000244, 0.3466666666666666785, 0.3533333333333333326, 0.3599999999999999867, 0.3666666666666666408, 0.3733333333333333504, 0.3800000000000000044, 0.3866666666666666585, 0.3933333333333333126, 0.4000000000000000222, 0.4066666666666666763, 0.4133333333333333304, 0.4199999999999999845, 0.4266666666666666941, 0.4333333333333333481, 0.4400000000000000022, 0.4466666666666666563, 0.4533333333333333104, 0.4600000000000000200, 0.4666666666666666741, 0.4733333333333333282, 0.4799999999999999822, 0.4866666666666666918, 0.4933333333333333459, 0.5000000000000000000, 0.5066666666666667096, 0.5133333333333333082, 0.5200000000000000178, 0.5266666666666666163, 0.5333333333333333259, 0.5400000000000000355, 0.5466666666666666341, 0.5533333333333333437, 0.5600000000000000533, 0.5666666666666666519, 0.5733333333333333615, 0.5799999999999999600, 0.5866666666666666696, 0.5933333333333333792, 0.5999999999999999778, 0.6066666666666666874, 0.6133333333333332860, 0.6199999999999999956, 0.6266666666666667052, 0.6333333333333333037, 0.6400000000000000133, 0.6466666666666666119, 0.6533333333333333215, 0.6600000000000000311, 0.6666666666666666297, 0.6733333333333333393, 0.6800000000000000488, 0.6866666666666666474, 0.6933333333333333570, 0.6999999999999999556, 0.7066666666666666652, 0.7133333333333333748, 0.7199999999999999734, 0.7266666666666666829, 0.7333333333333332815, 0.7399999999999999911, 0.7466666666666667007, 0.7533333333333332993, 0.7600000000000000089, 0.7666666666666667185, 0.7733333333333333171, 0.7800000000000000266, 0.7866666666666666252, 0.7933333333333333348, 0.8000000000000000444, 0.8066666666666666430, 0.8133333333333333526, 0.8199999999999999512, 0.8266666666666666607, 0.8333333333333333703, 0.8399999999999999689, 0.8466666666666666785, 0.8533333333333333881, 0.8599999999999999867, 0.8666666666666666963, 0.8733333333333332948, 0.8800000000000000044, 0.8866666666666667140, 0.8933333333333333126, 0.9000000000000000222, 0.9066666666666666208, 0.9133333333333333304, 0.9200000000000000400, 0.9266666666666666385, 0.9333333333333333481, 0.9399999999999999467, 0.9466666666666666563, 0.9533333333333333659, 0.9599999999999999645, 0.9666666666666666741, 0.9733333333333333837, 0.9799999999999999822, 0.9866666666666666918, 0.9933333333333332904, 1.000000000000000000 ),
 .UNSPECIFIED. ) 
 GEOMETRIC_REPRESENTATION_ITEM ( )  RATIONAL_B_SPLINE_SURFACE ( (
 ( 1.000000000000000000, 0.9510565162951535312, 1.000000000000000000, 0.9510565162951535312, 1.000000000000000000, 0.9510565162951535312, 1.000000000000000000, 0.9510565162951535312, 1.000000000000000000, 0.9510565162951535312, 1.000000000000000000, 0.9510565162951535312, 1.000000000000000000, 0.9510565162951535312, 1.000000000000000000, 0.9510565162951535312, 1.000000000000000000, 0.9510565162951535312, 1.000000000000000000, 0.9510565162951535312, 1.000000000000000000, 0.9510565162951535312, 1.000000000000000000, 0.9510565162951535312, 1.000000000000000000, 0.9510565162951535312, 1.000000000000000000, 0.9510565162951535312, 1.000000000000000000, 0.9510565162951535312, 1.000000000000000000, 0.9510565162951535312, 1.000000000000000000, 0.9510565162951535312, 1.000000000000000000, 0.9510565162951535312, 1.000000000000000000, 0.9510565162951535312, 1.000000000000000000, 0.9510565162951535312, 1.000000000000000000, 0.9510565162951535312, 1.000000000000000000, 0.9510565162951535312, 1.000000000000000000, 0.9510565162951535312, 1.000000000000000000, 0.9510565162951535312, 1.000000000000000000, 0.9510565162951535312, 1.000000000000000000, 0.9510565162951535312, 1.000000000000000000, 0.9510565162951535312, 1.000000000000000000, 0.9510565162951535312, 1.000000000000000000, 0.9510565162951535312, 1.000000000000000000, 0.9510565162951535312, 1.000000000000000000, 0.9510565162951535312, 1.000000000000000000, 0.9510565162951535312, 1.000000000000000000, 0.9510565162951535312, 1.000000000000000000, 0.9510565162951535312, 1.000000000000000000, 0.9510565162951535312, 1.000000000000000000, 0.9510565162951535312, 1.000000000000000000, 0.9510565162951535312, 1.000000000000000000, 0.9510565162951535312, 1.000000000000000000, 0.9510565162951535312, 1.000000000000000000, 0.9510565162951535312, 1.000000000000000000, 0.9510565162951535312, 1.000000000000000000, 0.9510565162951535312, 1.000000000000000000, 0.9510565162951535312, 1.000000000000000000, 0.9510565162951535312, 1.000000000000000000, 0.9510565162951535312, 1.000000000000000000, 0.9510565162951535312, 1.000000000000000000, 0.9510565162951535312, 1.000000000000000000, 0.9510565162951535312, 1.000000000000000000, 0.9510565162951535312, 1.000000000000000000, 0.9510565162951535312, 1.000000000000000000, 0.9510565162951535312, 1.000000000000000000, 0.9510565162951535312, 1.000000000000000000, 0.9510565162951535312, 1.000000000000000000, 0.9510565162951535312, 1.000000000000000000, 0.9510565162951535312, 1.000000000000000000, 0.9510565162951535312, 1.000000000000000000, 0.9510565162951535312, 1.000000000000000000, 0.9510565162951535312, 1.000000000000000000, 0.9510565162951535312, 1.000000000000000000, 0.9510565162951535312, 1.000000000000000000, 0.9510565162951535312, 1.000000000000000000, 0.9510565162951535312, 1.000000000000000000, 0.9510565162951535312, 1.000000000000000000, 0.9510565162951535312, 1.000000000000000000, 0.9510565162951535312, 1.000000000000000000, 0.9510565162951535312, 1.000000000000000000, 0.9510565162951535312, 1.000000000000000000, 0.9510565162951535312, 1.000000000000000000, 0.9510565162951535312, 1.000000000000000000, 0.9510565162951535312, 1.000000000000000000, 0.9510565162951535312, 1.000000000000000000, 0.9510565162951535312, 1.000000000000000000, 0.9510565162951535312, 1.000000000000000000, 0.9510565162951535312, 1.000000000000000000, 0.9510565162951535312, 1.000000000000000000, 0.9510565162951535312, 1.000000000000000000, 0.9510565162951535312, 1.000000000000000000, 0.9510565162951535312, 1.000000000000000000, 0.9510565162951535312, 1.000000000000000000, 0.9510565162951535312, 1.000000000000000000, 0.9510565162951535312, 1.000000000000000000, 0.9510565162951535312, 1.000000000000000000, 0.9510565162951535312, 1.000000000000000000, 0.9510565162951535312, 1.000000000000000000, 0.9510565162951535312, 1.000000000000000000, 0.9510565162951535312, 1.000000000000000000, 0.9510565162951535312, 1.000000000000000000, 0.9510565162951535312, 1.000000000000000000, 0.9510565162951535312, 1.000000000000000000, 0.9510565162951535312, 1.000000000000000000, 0.9510565162951535312, 1.000000000000000000, 0.9510565162951535312, 1.000000000000000000, 0.9510565162951535312, 1.000000000000000000, 0.9510565162951535312, 1.000000000000000000, 0.9510565162951535312, 1.000000000000000000, 0.9510565162951535312, 1.000000000000000000, 0.9510565162951535312, 1.000000000000000000, 0.9510565162951535312, 1.000000000000000000, 0.9510565162951535312, 1.000000000000000000, 0.9510565162951535312, 1.000000000000000000, 0.9510565162951535312, 1.000000000000000000, 0.9510565162951535312, 1.000000000000000000, 0.9510565162951535312, 1.000000000000000000, 0.9510565162951535312, 1.000000000000000000, 0.9510565162951535312, 1.000000000000000000, 0.9510565162951535312, 1.000000000000000000, 0.9510565162951535312, 1.000000000000000000, 0.9510565162951535312, 1.000000000000000000, 0.9510565162951535312, 1.000000000000000000, 0.9510565162951535312, 1.000000000000000000, 0.9510565162951535312, 1.000000000000000000, 0.9510565162951535312, 1.000000000000000000, 0.9510565162951535312, 1.000000000000000000, 0.9510565162951535312, 1.000000000000000000, 0.9510565162951535312, 1.000000000000000000, 0.9510565162951535312, 1.000000000000000000, 0.9510565162951535312, 1.000000000000000000, 0.9510565162951535312, 1.000000000000000000, 0.9510565162951535312, 1.000000000000000000, 0.9510565162951535312, 1.000000000000000000, 0.9510565162951535312, 1.000000000000000000, 0.9510565162951535312, 1.000000000000000000, 0.9510565162951535312, 1.000000000000000000, 0.9510565162951535312, 1.000000000000000000, 0.9510565162951535312, 1.000000000000000000, 0.9510565162951535312, 1.000000000000000000, 0.9510565162951535312, 1.000000000000000000, 0.9510565162951535312, 1.000000000000000000, 0.9510565162951535312, 1.000000000000000000, 0.9510565162951535312, 1.000000000000000000, 0.9510565162951535312, 1.000000000000000000, 0.9510565162951535312, 1.000000000000000000, 0.9510565162951535312, 1.000000000000000000, 0.9510565162951535312, 1.000000000000000000, 0.9510565162951535312, 1.000000000000000000, 0.9510565162951535312, 1.000000000000000000, 0.9510565162951535312, 1.000000000000000000, 0.9510565162951535312, 1.000000000000000000, 0.9510565162951535312, 1.000000000000000000, 0.9510565162951535312, 1.000000000000000000, 0.9510565162951535312, 1.000000000000000000, 0.9510565162951535312, 1.000000000000000000, 0.9510565162951535312, 1.000000000000000000, 0.9510565162951535312, 1.000000000000000000, 0.9510565162951535312, 1.000000000000000000, 0.9510565162951535312, 1.000000000000000000, 0.9510565162951535312, 1.000000000000000000, 0.9510565162951535312, 1.000000000000000000, 0.9510565162951535312, 1.000000000000000000, 0.9510565162951535312, 1.000000000000000000),
 ( 1.000000000000000000, 0.9510565162951535312, 1.000000000000000000, 0.9510565162951535312, 1.000000000000000000, 0.9510565162951535312, 1.000000000000000000, 0.9510565162951535312, 1.000000000000000000, 0.9510565162951535312, 1.000000000000000000, 0.9510565162951535312, 1.000000000000000000, 0.9510565162951535312, 1.000000000000000000, 0.9510565162951535312, 1.000000000000000000, 0.9510565162951535312, 1.000000000000000000, 0.9510565162951535312, 1.000000000000000000, 0.9510565162951535312, 1.000000000000000000, 0.9510565162951535312, 1.000000000000000000, 0.9510565162951535312, 1.000000000000000000, 0.9510565162951535312, 1.000000000000000000, 0.9510565162951535312, 1.000000000000000000, 0.9510565162951535312, 1.000000000000000000, 0.9510565162951535312, 1.000000000000000000, 0.9510565162951535312, 1.000000000000000000, 0.9510565162951535312, 1.000000000000000000, 0.9510565162951535312, 1.000000000000000000, 0.9510565162951535312, 1.000000000000000000, 0.9510565162951535312, 1.000000000000000000, 0.9510565162951535312, 1.000000000000000000, 0.9510565162951535312, 1.000000000000000000, 0.9510565162951535312, 1.000000000000000000, 0.9510565162951535312, 1.000000000000000000, 0.9510565162951535312, 1.000000000000000000, 0.9510565162951535312, 1.000000000000000000, 0.9510565162951535312, 1.000000000000000000, 0.9510565162951535312, 1.000000000000000000, 0.9510565162951535312, 1.000000000000000000, 0.9510565162951535312, 1.000000000000000000, 0.9510565162951535312, 1.000000000000000000, 0.9510565162951535312, 1.000000000000000000, 0.9510565162951535312, 1.000000000000000000, 0.9510565162951535312, 1.000000000000000000, 0.9510565162951535312, 1.000000000000000000, 0.9510565162951535312, 1.000000000000000000, 0.9510565162951535312, 1.000000000000000000, 0.9510565162951535312, 1.000000000000000000, 0.9510565162951535312, 1.000000000000000000, 0.9510565162951535312, 1.000000000000000000, 0.9510565162951535312, 1.000000000000000000, 0.9510565162951535312, 1.000000000000000000, 0.9510565162951535312, 1.000000000000000000, 0.9510565162951535312, 1.000000000000000000, 0.9510565162951535312, 1.000000000000000000, 0.9510565162951535312, 1.000000000000000000, 0.9510565162951535312, 1.000000000000000000, 0.9510565162951535312, 1.000000000000000000, 0.9510565162951535312, 1.000000000000000000, 0.9510565162951535312, 1.000000000000000000, 0.9510565162951535312, 1.000000000000000000, 0.9510565162951535312, 1.000000000000000000, 0.9510565162951535312, 1.000000000000000000, 0.9510565162951535312, 1.000000000000000000, 0.9510565162951535312, 1.000000000000000000, 0.9510565162951535312, 1.000000000000000000, 0.9510565162951535312, 1.000000000000000000, 0.9510565162951535312, 1.000000000000000000, 0.9510565162951535312, 1.000000000000000000, 0.9510565162951535312, 1.000000000000000000, 0.9510565162951535312, 1.000000000000000000, 0.9510565162951535312, 1.000000000000000000, 0.9510565162951535312, 1.000000000000000000, 0.9510565162951535312, 1.000000000000000000, 0.9510565162951535312, 1.000000000000000000, 0.9510565162951535312, 1.000000000000000000, 0.9510565162951535312, 1.000000000000000000, 0.9510565162951535312, 1.000000000000000000, 0.9510565162951535312, 1.000000000000000000, 0.9510565162951535312, 1.000000000000000000, 0.9510565162951535312, 1.000000000000000000, 0.9510565162951535312, 1.000000000000000000, 0.9510565162951535312, 1.000000000000000000, 0.9510565162951535312, 1.000000000000000000, 0.9510565162951535312, 1.000000000000000000, 0.9510565162951535312, 1.000000000000000000, 0.9510565162951535312, 1.000000000000000000, 0.9510565162951535312, 1.000000000000000000, 0.9510565162951535312, 1.000000000000000000, 0.9510565162951535312, 1.000000000000000000, 0.9510565162951535312, 1.000000000000000000, 0.9510565162951535312, 1.000000000000000000, 0.9510565162951535312, 1.000000000000000000, 0.9510565162951535312, 1.000000000000000000, 0.9510565162951535312, 1.000000000000000000, 0.9510565162951535312, 1.000000000000000000, 0.9510565162951535312, 1.000000000000000000, 0.9510565162951535312, 1.000000000000000000, 0.9510565162951535312, 1.000000000000000000, 0.9510565162951535312, 1.000000000000000000, 0.9510565162951535312, 1.000000000000000000, 0.9510565162951535312, 1.000000000000000000, 0.9510565162951535312, 1.000000000000000000, 0.9510565162951535312, 1.000000000000000000, 0.9510565162951535312, 1.000000000000000000, 0.9510565162951535312, 1.000000000000000000, 0.9510565162951535312, 1.000000000000000000, 0.9510565162951535312, 1.000000000000000000, 0.9510565162951535312, 1.000000000000000000, 0.9510565162951535312, 1.000000000000000000, 0.9510565162951535312, 1.000000000000000000, 0.9510565162951535312, 1.000000000000000000, 0.9510565162951535312, 1.000000000000000000, 0.9510565162951535312, 1.000000000000000000, 0.9510565162951535312, 1.000000000000000000, 0.9510565162951535312, 1.000000000000000000, 0.9510565162951535312, 1.000000000000000000, 0.9510565162951535312, 1.000000000000000000, 0.9510565162951535312, 1.000000000000000000, 0.9510565162951535312, 1.000000000000000000, 0.9510565162951535312, 1.000000000000000000, 0.9510565162951535312, 1.000000000000000000, 0.9510565162951535312, 1.000000000000000000, 0.9510565162951535312, 1.000000000000000000, 0.9510565162951535312, 1.000000000000000000, 0.9510565162951535312, 1.000000000000000000, 0.9510565162951535312, 1.000000000000000000, 0.9510565162951535312, 1.000000000000000000, 0.9510565162951535312, 1.000000000000000000, 0.9510565162951535312, 1.000000000000000000, 0.9510565162951535312, 1.000000000000000000, 0.9510565162951535312, 1.000000000000000000, 0.9510565162951535312, 1.000000000000000000, 0.9510565162951535312, 1.000000000000000000, 0.9510565162951535312, 1.000000000000000000, 0.9510565162951535312, 1.000000000000000000, 0.9510565162951535312, 1.000000000000000000, 0.9510565162951535312, 1.000000000000000000, 0.9510565162951535312, 1.000000000000000000, 0.9510565162951535312, 1.000000000000000000, 0.9510565162951535312, 1.000000000000000000, 0.9510565162951535312, 1.000000000000000000, 0.9510565162951535312, 1.000000000000000000, 0.9510565162951535312, 1.000000000000000000, 0.9510565162951535312, 1.000000000000000000, 0.9510565162951535312, 1.000000000000000000, 0.9510565162951535312, 1.000000000000000000, 0.9510565162951535312, 1.000000000000000000, 0.9510565162951535312, 1.000000000000000000, 0.9510565162951535312, 1.000000000000000000, 0.9510565162951535312, 1.000000000000000000, 0.9510565162951535312, 1.000000000000000000, 0.9510565162951535312, 1.000000000000000000, 0.9510565162951535312, 1.000000000000000000, 0.9510565162951535312, 1.000000000000000000, 0.9510565162951535312, 1.000000000000000000, 0.9510565162951535312, 1.000000000000000000, 0.9510565162951535312, 1.000000000000000000) ) ) 
 REPRESENTATION_ITEM ( '' )  SURFACE ( )  );
#964=CARTESIAN_POINT ( 'NONE',  ( -49.99999999999999289, 39.88125000068280457, 16.24598481164533226 ) ) ;
#967=CARTESIAN_POINT ( 'NONE',  ( 7.919222016226875382, 37.22999571913595673, -49.99999999999997158 ) ) ;
#968=CARTESIAN_POINT ( 'NONE',  ( 40.34137639590981195, 39.05937500034140442, -29.30972558990011834 ) ) ;
#970=CARTESIAN_POINT ( 'NONE',  ( 49.86468353125000164, 44.85937500034140157, -6.106662507704105588E-15 ) ) ;
#973=CARTESIAN_POINT ( 'NONE',  ( -49.86468353124999453, 49.82187500034139305, -16.20201782572375393 ) ) ;
#975=CARTESIAN_POINT ( 'NONE',  ( 1.293669679204937499E-13, 41.50000000000000000, -50.00000000000000000 ) ) ;
#984=CARTESIAN_POINT ( 'NONE',  ( -1.240322475938754499E-13, 40.50000000000000000, 50.00000000000000000 ) ) ;
#988=CARTESIAN_POINT ( 'NONE',  ( -14.89909204896622263, 13.30277682295380615, 96.51165749809530325 ) ) ;
#990=CARTESIAN_POINT ( 'NONE',  ( 0.000000000000000000, 20.00000000000000355, 0.000000000000000000 ) ) ;
#995=CARTESIAN_POINT ( 'NONE',  ( 15.45084971874737789, 46.38125000068279746, 47.55282581475767500 ) ) ;
#998=CARTESIAN_POINT ( 'NONE',  ( -30.90169943749473447, 26.29999999999999716, 42.53254041760200721 ) ) ;
#1011=CARTESIAN_POINT ( 'NONE',  ( 50.00000000000000000, 35.00000000000000000, -6.123233995736766085E-15 ) ) ;
#1013=CARTESIAN_POINT ( 'NONE',  ( 49.86468353125001585, 20.82187500034140015, 16.20201782572375038 ) ) ;
#1014=CARTESIAN_POINT ( 'NONE',  ( 9.631387414534489405E-15, 32.35937500034139447, 52.43083105670540789 ) ) ;
#1015=CARTESIAN_POINT ( 'NONE',  ( -7.919222016226816763, 35.55125428154684641, -49.99999999999999289 ) ) ;
#1016=CARTESIAN_POINT ( 'NONE',  ( -49.86468353125000164, 35.92187500034140157, 0.000000000000000000 ) ) ;
#1017=CARTESIAN_POINT ( 'NONE',  ( 0.000000000000000000, 20.00000000000000355, 0.000000000000000000 ) ) ;
#1018=VECTOR ( 'NONE', #4511, 1000.000000000000000 ) ;
#1020=CARTESIAN_POINT ( 'NONE',  ( -40.34137639590981195, 38.05937500034139731, 29.30972558990012189 ) ) ;
#1022=CARTESIAN_POINT ( 'NONE',  ( 50.00000000000000000, 45.00000000000000711, -6.123233995736766085E-15 ) ) ;
#1029=CARTESIAN_POINT ( 'NONE',  ( -1.240322475938754499E-13, 40.28125000068280315, 50.00000000000000000 ) ) ;
#1030=CARTESIAN_POINT ( 'NONE',  ( 15.40903463028482356, 42.52187500034139589, 47.42413220539093999 ) ) ;
#1034=CARTESIAN_POINT ( 'NONE',  ( 15.45084971874736723, 37.18125000068280173, -47.55282581475768211 ) ) ;
#1035=CARTESIAN_POINT ( 'NONE',  ( -49.86468353125000164, 35.92187500034140157, 0.000000000000000000 ) ) ;
#1045=CARTESIAN_POINT ( 'NONE',  ( 30.90169943749473802, 27.29999999999999716, -42.53254041760200721 ) ) ;
#1046=CARTESIAN_POINT ( 'NONE',  ( -40.45084971874737789, 23.58125000068280031, -29.38926261462365730 ) ) ;
#1048=CARTESIAN_POINT ( 'NONE',  ( 49.86468353124999453, 36.95937500034139589, -16.20201782572376459 ) ) ;
#1050=CARTESIAN_POINT ( 'NONE',  ( -3.210462471511496205E-15, 45.35937500034139447, -52.43083105670540789 ) ) ;
#1055=CARTESIAN_POINT ( 'NONE',  ( 40.45084971874737789, 40.80000000000000426, 29.38926261462365375 ) ) ;
#1061=ORIENTED_EDGE ( 'NONE', *, *, #9175, .F. ) ;
#1067=CARTESIAN_POINT ( 'NONE',  ( 8.660254037844387298, 28.00000000000000355, 5.000000000000000000 ) ) ;
#1069=CARTESIAN_POINT ( 'NONE',  ( -14.27211209225524158, 12.35708747557853826, 96.77492152178915319 ) ) ;
#1074=PRESENTATION_STYLE_ASSIGNMENT (( #12482 ) ) ;
#1076=CARTESIAN_POINT ( 'NONE',  ( 30.90169943749474157, 47.08125000068280031, -42.53254041760200721 ) ) ;
#1080=CARTESIAN_POINT ( 'NONE',  ( -15.45084971874737256, 25.60000000000000142, -47.55282581475767500 ) ) ;
#1088=CARTESIAN_POINT ( 'NONE',  ( -7.919222016226934890, 20.22999571913595318, 49.99999999999996447 ) ) ;
#1089=DIRECTION ( 'NONE',  ( -0.000000000000000000, 1.000000000000000000, -0.000000000000000000 ) ) ;
#1092=CARTESIAN_POINT ( 'NONE',  ( 40.34137639590981195, 21.12187500034139376, -29.30972558990011834 ) ) ;
#1093=CARTESIAN_POINT ( 'NONE',  ( -40.34137639590981195, 30.05937500034139731, 29.30972558990012189 ) ) ;
#1095=CARTESIAN_POINT ( 'NONE',  ( 30.81806926056962936, 33.22187500034139163, -42.41743335407646498 ) ) ;
#1096=CARTESIAN_POINT ( 'NONE',  ( -15.45084971874736368, 40.40000000000000568, 47.55282581475768211 ) ) ;
#1097=CARTESIAN_POINT ( 'NONE',  ( 49.86468353125001585, 40.75937500034138594, 16.20201782572375038 ) ) ;
#1099=CARTESIAN_POINT ( 'NONE',  ( 49.99999999999999289, 43.10000000000000142, -16.24598481164532160 ) ) ;
#1107=CARTESIAN_POINT ( 'NONE',  ( 15.40903463028481113, 39.32187500034140015, -47.42413220539094709 ) ) ;
#1111=CARTESIAN_POINT ( 'NONE',  ( 49.99999999999999289, 30.88125000068279391, -16.24598481164532160 ) ) ;
#1113=CARTESIAN_POINT ( 'NONE',  ( -49.86468353125000164, 31.92187500034139447, 0.000000000000000000 ) ) ;
#1117=FACE_OUTER_BOUND ( 'NONE', #4619, .T. ) ;
#1124=CARTESIAN_POINT ( 'NONE',  ( -30.90169943749474513, 49.48125000068279178, -42.53254041760200721 ) ) ;
#1126=CARTESIAN_POINT ( 'NONE',  ( -30.81806926056962226, 30.15937500034139163, 42.41743335407647919 ) ) ;
#1128=CARTESIAN_POINT ( 'NONE',  ( 49.86468353124999453, 47.02187500034139589, -16.20201782572376104 ) ) ;
#1147=LINE ( 'NONE', #16290, #13270 ) ;
#1150=CARTESIAN_POINT ( 'NONE',  ( -2.547328955960238000E-13, 32.28125000068278894, 49.99999999999999289 ) ) ;
#1153=CARTESIAN_POINT ( 'NONE',  ( -30.90169943749473802, 46.08125000068278609, 42.53254041760200721 ) ) ;
#1157=CARTESIAN_POINT ( 'NONE',  ( -30.81806926056962226, 22.15937500034139873, 42.41743335407647919 ) ) ;
#1165=EDGE_CURVE ( 'NONE', #5069, #10216, #1357, .T. ) ;
#1170=AXIS2_PLACEMENT_3D ( 'NONE', #2365, #12760, #7448 ) ;
#1172=CARTESIAN_POINT ( 'NONE',  ( -49.86468353124999453, 25.82187500034139305, -16.20201782572375393 ) ) ;
#1173=CARTESIAN_POINT ( 'NONE',  ( -40.34137639590981905, 21.65937500034139518, -29.30972558990011478 ) ) ;
#1175=CARTESIAN_POINT ( 'NONE',  ( -15.40903463028480580, 34.32187500034139305, 47.42413220539094709 ) ) ;
#1177=CARTESIAN_POINT ( 'NONE',  ( 49.99999999999999289, 35.10000000000000853, -16.24598481164532160 ) ) ;
#1178=CARTESIAN_POINT ( 'NONE',  ( 49.86468353125000164, 38.85937500034139447, -6.106662507704105588E-15 ) ) ;
#1180=CARTESIAN_POINT ( 'NONE',  ( 50.00000000000000000, 43.00000000000000000, -6.123233995736766085E-15 ) ) ;
#1185=ORIENTED_EDGE ( 'NONE', *, *, #11085, .T. ) ;
#1187=CARTESIAN_POINT ( 'NONE',  ( -49.99999999999999289, 33.89999999999999147, -16.24598481164531449 ) ) ;
#1190=CARTESIAN_POINT ( 'NONE',  ( 30.81806926056964002, 42.62187500034139731, 42.41743335407647209 ) ) ;
#1194=CARTESIAN_POINT ( 'NONE',  ( 9.657523855033129090E-15, 30.28125000068279604, 52.57311121191334990 ) ) ;
#1196=CARTESIAN_POINT ( 'NONE',  ( -30.81806926056963292, 35.62187500034140442, -42.41743335407647209 ) ) ;
#1205=EDGE_CURVE ( 'NONE', #13562, #9978, #13349, .T. ) ;
#1211=CARTESIAN_POINT ( 'NONE',  ( -48.35726954556750457, 20.00000000000000355, 12.16803787670978387 ) ) ;
#1212=CARTESIAN_POINT ( 'NONE',  ( -30.81806926056963292, 33.55937500034138310, -42.41743335407647209 ) ) ;
#1215=CARTESIAN_POINT ( 'NONE',  ( 30.81806926056964002, 46.62187500034139731, 42.41743335407646498 ) ) ;
#1230=AXIS2_PLACEMENT_3D ( 'NONE', #3697, #5194, #11341 ) ;
#1236=CARTESIAN_POINT ( 'NONE',  ( 9.631387414534489405E-15, 48.35937500034140157, 52.43083105670540789 ) ) ;
#1241=CARTESIAN_POINT ( 'NONE',  ( 40.45084971874737079, 44.98125000068279888, -29.38926261462366440 ) ) ;
#1257=CARTESIAN_POINT ( 'NONE',  ( -15.72858266790894177, 30.19372578669147344, 93.36074974597489984 ) ) ;
#1263=CARTESIAN_POINT ( 'NONE',  ( 30.81806926056962936, 25.15937500034139518, -42.41743335407646498 ) ) ;
#1265=CARTESIAN_POINT ( 'NONE',  ( 49.86468353125000164, 36.92187500034140157, -6.106662507704105588E-15 ) ) ;
#1267=CARTESIAN_POINT ( 'NONE',  ( -49.99999999999999289, 33.90000000000000568, -16.24598481164531449 ) ) ;
#1268=CARTESIAN_POINT ( 'NONE',  ( -15.40903463028481646, 39.45937500034139589, -47.42413220539093999 ) ) ;
#1270=CARTESIAN_POINT ( 'NONE',  ( -50.00000000000000000, 46.00000000000000000, 0.000000000000000000 ) ) ;
#1272=ORIENTED_EDGE ( 'NONE', *, *, #8288, .T. ) ;
#1273=ORIENTED_EDGE ( 'NONE', *, *, #3682, .T. ) ;
#1283=CARTESIAN_POINT ( 'NONE',  ( 30.81806926056964002, 40.62187500034139731, 42.41743335407647209 ) ) ;
#1286=CARTESIAN_POINT ( 'NONE',  ( -15.45084971874736368, 30.18125000068280173, 47.55282581475768211 ) ) ;
#1287=CARTESIAN_POINT ( 'NONE',  ( 15.75363786119666720, 30.20531192536913423, 93.35498375726734821 ) ) ;
#1288=CARTESIAN_POINT ( 'NONE',  ( -3.210462471511496205E-15, 37.42187500034140157, -52.43083105670540789 ) ) ;
#1289=CARTESIAN_POINT ( 'NONE',  ( 50.00000000000000711, 38.89999999999999858, 16.24598481164530739 ) ) ;
#1290=CARTESIAN_POINT ( 'NONE',  ( -49.99999999999999289, 27.89999999999999858, -16.24598481164531449 ) ) ;
#1292=ORIENTED_EDGE ( 'NONE', *, *, #6562, .F. ) ;
#1295=EDGE_CURVE ( 'NONE', #15320, #4877, #6671, .T. ) ;
#1298=CARTESIAN_POINT ( 'NONE',  ( -15.40903463028480580, 28.25937500034139660, 47.42413220539094709 ) ) ;
#1299=CARTESIAN_POINT ( 'NONE',  ( 0.000000000000000000, 50.00000000000000000, 0.000000000000000000 ) ) ;
#1300=CARTESIAN_POINT ( 'NONE',  ( 30.81806926056962936, 43.22187500034139873, -42.41743335407646498 ) ) ;
#1302=DIRECTION ( 'NONE',  ( -0.000000000000000000, -1.000000000000000000, -0.000000000000000000 ) ) ;
#1308=CARTESIAN_POINT ( 'NONE',  ( -30.90169943749473447, 46.08125000068279320, 42.53254041760200721 ) ) ;
#1311=ORIENTED_EDGE ( 'NONE', *, *, #8778, .T. ) ;
#1313=CARTESIAN_POINT ( 'NONE',  ( -49.86468353125000164, 49.85937500034139447, 0.000000000000000000 ) ) ;
#1314=CARTESIAN_POINT ( 'NONE',  ( -2.547328955960238000E-13, 24.28125000068279604, 49.99999999999999289 ) ) ;
#1316=CARTESIAN_POINT ( 'NONE',  ( 50.00000000000000711, 32.68125000068279462, 16.24598481164530739 ) ) ;
#1320=FACE_OUTER_BOUND ( 'NONE', #15807, .T. ) ;
#1321=CARTESIAN_POINT ( 'NONE',  ( 40.45084971874737789, 42.58125000068280031, 29.38926261462365375 ) ) ;
#1325=CARTESIAN_POINT ( 'NONE',  ( 30.81806926056964002, 20.55937500034139376, 42.41743335407647209 ) ) ;
#1337=CARTESIAN_POINT ( 'NONE',  ( -17.50000000000000000, 23.06298493376378289, 94.32371117417838491 ) ) ;
#1341=CARTESIAN_POINT ( 'NONE',  ( -30.81806926056962226, 24.15937500034140228, 42.41743335407647209 ) ) ;
#1342=LINE ( 'NONE', #2757, #2302 ) ;
#1343=CARTESIAN_POINT ( 'NONE',  ( -49.86468353124999453, 33.82187500034138594, -16.20201782572375393 ) ) ;
#1344=CYLINDRICAL_SURFACE ( 'NONE', #8409, 50.00000000000000000 ) ;
#1345=CARTESIAN_POINT ( 'NONE',  ( -30.90169943749473802, 30.29999999999999716, 42.53254041760200721 ) ) ;
#1346=CARTESIAN_POINT ( 'NONE',  ( -15.40903463028481646, 37.45937500034139589, -47.42413220539093999 ) ) ;
#1348=CARTESIAN_POINT ( 'NONE',  ( 40.45084971874737789, 42.80000000000000426, 29.38926261462365375 ) ) ;
#1357=( BOUNDED_CURVE ( )  B_SPLINE_CURVE ( 2, ( #5176, #13798, #15047, #7569, #5020, #11320, #12645, #10232, #16298, #15291, #16386, #9909, #5097 ),
 .UNSPECIFIED., .F., .T. ) 
 B_SPLINE_CURVE_WITH_KNOTS ( ( 3, 2, 2, 2, 2, 2, 3 ),
 ( 0.9500000000000000666, 0.9533333333333333659, 0.9599999999999999645, 0.9666666666666666741, 0.9733333333333333837, 0.9799999999999999822, 0.9833333333333333925 ),
 .UNSPECIFIED. ) 
 CURVE ( )  GEOMETRIC_REPRESENTATION_ITEM ( )  RATIONAL_B_SPLINE_CURVE ( ( 0.9755282581475768211, 0.9755282581475771542, 1.000000000000000000, 0.9510565162951535312, 1.000000000000000000, 0.9510565162951535312, 1.000000000000000000, 0.9510565162951535312, 1.000000000000000000, 0.9510565162951535312, 1.000000000000000000, 0.9755282581475763770, 0.9755282581475768211 ) ) 
 REPRESENTATION_ITEM ( '' )  );
#1362=CARTESIAN_POINT ( 'NONE',  ( -15.40903463028480580, 44.32187500034140015, 47.42413220539094709 ) ) ;
#1363=CARTESIAN_POINT ( 'NONE',  ( -15.40903463028481646, 45.45937500034139589, -47.42413220539093999 ) ) ;
#1366=CARTESIAN_POINT ( 'NONE',  ( -49.99999999999999289, 29.88125000068279391, 16.24598481164533226 ) ) ;
#1367=CARTESIAN_POINT ( 'NONE',  ( 10.69265510062280100, 36.36533908517922242, 92.97600696701006484 ) ) ;
#1368=CARTESIAN_POINT ( 'NONE',  ( -49.86468353124999453, 32.02187500034139589, 16.20201782572377525 ) ) ;
#1371=EDGE_CURVE ( 'NONE', #15116, #12470, #2527, .T. ) ;
#1373=ORIENTED_EDGE ( 'NONE', *, *, #5410, .T. ) ;
#1377=CARTESIAN_POINT ( 'NONE',  ( -49.99999999999999289, 24.10000000000000142, 16.24598481164533226 ) ) ;
#1378=DIRECTION ( 'NONE',  ( 0.000000000000000000, 0.000000000000000000, 1.000000000000000000 ) ) ;
#1379=CARTESIAN_POINT ( 'NONE',  ( -49.86468353124999453, 33.75937500034140015, -16.20201782572375393 ) ) ;
#1381=CARTESIAN_POINT ( 'NONE',  ( 15.40903463028481113, 49.32187500034139305, -47.42413220539094709 ) ) ;
#1391=ORIENTED_EDGE ( 'NONE', *, *, #564, .T. ) ;
#1397=CARTESIAN_POINT ( 'NONE',  ( -3.210462471511496205E-15, 49.35937500034138736, -52.43083105670540789 ) ) ;
#1400=CARTESIAN_POINT ( 'NONE',  ( 30.90169943749475223, 24.48125000068279888, 42.53254041760199300 ) ) ;
#1403=CARTESIAN_POINT ( 'NONE',  ( -3.219174618344376363E-15, 43.28125000068280315, -52.57311121191334990 ) ) ;
#1411=CARTESIAN_POINT ( 'NONE',  ( 40.45084971874737079, 42.98125000068279888, -29.38926261462366440 ) ) ;
#1414=EDGE_CURVE ( 'NONE', #4999, #9634, #11090, .T. ) ;
#1416=CARTESIAN_POINT ( 'NONE',  ( -2.547328955960238000E-13, 32.50000000000000000, 49.99999999999999289 ) ) ;
#1421=CARTESIAN_POINT ( 'NONE',  ( -15.40903463028480580, 22.25937500034139660, 47.42413220539094709 ) ) ;
#1423=CARTESIAN_POINT ( 'NONE',  ( 30.81806926056962936, 31.22187500034139518, -42.41743335407646498 ) ) ;
#1424=EDGE_CURVE ( 'NONE', #4716, #8721, #4447, .T. ) ;
#1427=EDGE_CURVE ( 'NONE', #5069, #10576, #4749, .T. ) ;
#1428=CARTESIAN_POINT ( 'NONE',  ( 40.45084971874737079, 29.19999999999999929, -29.38926261462366440 ) ) ;
#1429=CARTESIAN_POINT ( 'NONE',  ( -49.86468353124999453, 31.95937500034139944, 16.20201782572377525 ) ) ;
#1431=CARTESIAN_POINT ( 'NONE',  ( -3.219174618344376363E-15, 41.49999999999999289, -52.57311121191334990 ) ) ;
#1437=EDGE_LOOP ( 'NONE', ( #8797, #14710, #1373, #13540 ) ) ;
#1438=ORIENTED_EDGE ( 'NONE', *, *, #16032, .F. ) ;
#1439=CARTESIAN_POINT ( 'NONE',  ( 0.000000000000000000, 0.000000000000000000, 100.0000000000000000 ) ) ;
#1441=AXIS2_PLACEMENT_3D ( 'NONE', #10549, #2890, #6473 ) ;
#1442=DIRECTION ( 'NONE',  ( -0.000000000000000000, 1.000000000000000000, -0.000000000000000000 ) ) ;
#1445=CARTESIAN_POINT ( 'NONE',  ( 15.40903463028481113, 35.32187500034139305, -47.42413220539094709 ) ) ;
#1446=CARTESIAN_POINT ( 'NONE',  ( 49.86468353125000164, 40.85937500034139447, -6.106662507704105588E-15 ) ) ;
#1449=CARTESIAN_POINT ( 'NONE',  ( 30.90169943749474157, 25.08125000068279675, -42.53254041760200721 ) ) ;
#1450=CARTESIAN_POINT ( 'NONE',  ( 3.979171442067388931, 39.55125785365773083, 92.94260441222228053 ) ) ;
#1452=CARTESIAN_POINT ( 'NONE',  ( -40.34137639590981195, 30.12187500034139731, 29.30972558990012189 ) ) ;
#1457=ORIENTED_EDGE ( 'NONE', *, *, #8755, .F. ) ;
#1462=CARTESIAN_POINT ( 'NONE',  ( -2.547328955960238000E-13, 24.49999999999999289, 49.99999999999999289 ) ) ;
#1464=CARTESIAN_POINT ( 'NONE',  ( -15.40903463028481646, 31.45937500034139944, -47.42413220539093999 ) ) ;
#1467=CARTESIAN_POINT ( 'NONE',  ( 30.81806926056962936, 47.22187500034139873, -42.41743335407646498 ) ) ;
#1471=CARTESIAN_POINT ( 'NONE',  ( 8.660254037844387298, 20.00000000000000355, 5.000000000000000000 ) ) ;
#1480=( GEOMETRIC_REPRESENTATION_CONTEXT ( 3 ) GLOBAL_UNCERTAINTY_ASSIGNED_CONTEXT ( ( #6443 ) ) GLOBAL_UNIT_ASSIGNED_CONTEXT ( ( #5094, #4932, #3993 ) ) REPRESENTATION_CONTEXT ( 'NONE', 'WORKASPACE' ) );
#1484=CARTESIAN_POINT ( 'NONE',  ( -49.99999999999999289, 22.09999999999999787, 16.24598481164533226 ) ) ;
#1493=CARTESIAN_POINT ( 'NONE',  ( 40.34137639590981195, 25.12187500034139376, -29.30972558990011834 ) ) ;
#1496=CARTESIAN_POINT ( 'NONE',  ( -40.45084971874737789, 39.58125000068280031, -29.38926261462365730 ) ) ;
#1498=CARTESIAN_POINT ( 'NONE',  ( 7.919222016226827421, 47.22999571913595673, -50.00000000000000000 ) ) ;
#1503=VECTOR ( 'NONE', #5732, 1000.000000000000227 ) ;
#1504=AXIS2_PLACEMENT_3D ( 'NONE', #8311, #13377, #1981 ) ;
#1506=DIRECTION ( 'NONE',  ( -0.000000000000000000, 1.000000000000000000, -0.000000000000000000 ) ) ;
#1508=ORIENTED_EDGE ( 'NONE', *, *, #2739, .T. ) ;
#1509=DIRECTION ( 'NONE',  ( 1.000000000000000000, 0.000000000000000000, -0.000000000000000000 ) ) ;
#1510=CARTESIAN_POINT ( 'NONE',  ( -15.18866191491423479, 31.21127306749596642, 93.26832743753136867 ) ) ;
#1514=CARTESIAN_POINT ( 'NONE',  ( -49.99999999999999289, 29.68125000068279817, -16.24598481164531449 ) ) ;
#1516=CARTESIAN_POINT ( 'NONE',  ( -30.81806926056963292, 21.55937500034140086, -42.41743335407646498 ) ) ;
#1517=CARTESIAN_POINT ( 'NONE',  ( -47.84248829804688086, 20.00000000000000355, 14.05740927763701187 ) ) ;
#1518=CARTESIAN_POINT ( 'NONE',  ( -49.86468353124999453, 27.82187500034139305, -16.20201782572375393 ) ) ;
#1521=CARTESIAN_POINT ( 'NONE',  ( 30.90169943749474157, 33.30000000000000426, -42.53254041760200721 ) ) ;
#1522=CARTESIAN_POINT ( 'NONE',  ( 15.40903463028481113, 29.25937500034139660, -47.42413220539094709 ) ) ;
#1535=CARTESIAN_POINT ( 'NONE',  ( -49.86468353124999453, 35.82187500034139305, -16.20201782572375393 ) ) ;
#1536=CARTESIAN_POINT ( 'NONE',  ( -15.40903463028480580, 44.25937500034140015, 47.42413220539094709 ) ) ;
#1540=CARTESIAN_POINT ( 'NONE',  ( 50.00000000000000711, 22.68125000068279462, 16.24598481164530739 ) ) ;
#1542=EDGE_CURVE ( 'NONE', #9634, #1788, #14255, .T. ) ;
#1543=CARTESIAN_POINT ( 'NONE',  ( -40.34137639590981195, 28.12187500034139731, 29.30972558990012189 ) ) ;
#1549=EDGE_CURVE ( 'NONE', #5607, #12984, #192, .T. ) ;
#1552=CARTESIAN_POINT ( 'NONE',  ( 30.81806926056964002, 26.55937500034139376, 42.41743335407647209 ) ) ;
#1553=CARTESIAN_POINT ( 'NONE',  ( 0.000000000000000000, 20.00000000000000355, 50.00000000000000000 ) ) ;
#1554=CARTESIAN_POINT ( 'NONE',  ( 40.34137639590981195, 39.12187500034139731, -29.30972558990011834 ) ) ;
#1557=CARTESIAN_POINT ( 'NONE',  ( 49.86468353125000164, 44.92187500034140157, -6.106662507704105588E-15 ) ) ;
#1559=ORIENTED_EDGE ( 'NONE', *, *, #4297, .F. ) ;
#1565=EDGE_CURVE ( 'NONE', #3318, #383, #2418, .T. ) ;
#1566=CARTESIAN_POINT ( 'NONE',  ( -49.99999999999999289, 43.68125000068280173, -16.24598481164531449 ) ) ;
#1569=CARTESIAN_POINT ( 'NONE',  ( -30.90169943749474868, 27.70000000000000284, -42.53254041760200721 ) ) ;
#1571=CARTESIAN_POINT ( 'NONE',  ( -49.86468353124999453, 45.75937500034140015, -16.20201782572375393 ) ) ;
#1574=CARTESIAN_POINT ( 'NONE',  ( 49.86468353124999453, 21.02187500034139589, -16.20201782572376459 ) ) ;
#1577=CARTESIAN_POINT ( 'NONE',  ( 40.45084971874737079, 42.98125000068279888, -29.38926261462366440 ) ) ;
#1578=CARTESIAN_POINT ( 'NONE',  ( -7.919222016226822092, 46.44874571845315359, 50.00000000000000000 ) ) ;
#1590=CARTESIAN_POINT ( 'NONE',  ( -13.21908673885165086, 34.02500059410989763, 93.06976900205165748 ) ) ;
#1594=CARTESIAN_POINT ( 'NONE',  ( 17.47157445415547983, 21.34957311187938700, 94.63625203854948609 ) ) ;
#1595=CARTESIAN_POINT ( 'NONE',  ( -46.68017951973648394, 20.00000000000001066, 17.53418100958496595 ) ) ;
#1596=CARTESIAN_POINT ( 'NONE',  ( -3.210462471511496205E-15, 29.42187500034139447, -52.43083105670540789 ) ) ;
#1597=CARTESIAN_POINT ( 'NONE',  ( -49.99999999999999289, 21.90000000000000213, -16.24598481164531449 ) ) ;
#1599=CARTESIAN_POINT ( 'NONE',  ( 49.86468353125000164, 32.85937500034139447, -6.106662507704105588E-15 ) ) ;
#1608=DIRECTION ( 'NONE',  ( 0.000000000000000000, 0.000000000000000000, 1.000000000000000000 ) ) ;
#1611=CARTESIAN_POINT ( 'NONE',  ( -49.86468353125000164, 35.92187500034140157, 0.000000000000000000 ) ) ;
#1612=CARTESIAN_POINT ( 'NONE',  ( -49.86468353124999453, 37.95937500034139589, 16.20201782572377169 ) ) ;
#1616=CARTESIAN_POINT ( 'NONE',  ( -30.81806926056963292, 49.55937500034139731, -42.41743335407647209 ) ) ;
#1618=CARTESIAN_POINT ( 'NONE',  ( 49.86468353124999453, 31.02187500034139234, -16.20201782572376459 ) ) ;
#1623=CARTESIAN_POINT ( 'NONE',  ( 0.000000000000000000, 20.00000000000000355, 0.000000000000000000 ) ) ;
#1628=CARTESIAN_POINT ( 'NONE',  ( 15.40903463028482356, 24.45937500034139589, 47.42413220539093999 ) ) ;
#1630=CARTESIAN_POINT ( 'NONE',  ( -49.86468353125000164, 41.92187500034139447, 0.000000000000000000 ) ) ;
#1634=CARTESIAN_POINT ( 'NONE',  ( 15.40903463028481113, 45.32187500034140015, -47.42413220539094709 ) ) ;
#1637=EDGE_CURVE ( 'NONE', #8883, #15854, #7499, .T. ) ;
#1643=CARTESIAN_POINT ( 'NONE',  ( -5.823736356558307894E-14, 44.28125000068280315, 50.00000000000000000 ) ) ;
#1646=CARTESIAN_POINT ( 'NONE',  ( 50.00000000000000000, 23.00000000000000355, -6.123233995736766085E-15 ) ) ;
#1647=CARTESIAN_POINT ( 'NONE',  ( -30.81806926056963292, 41.55937500034139731, -42.41743335407647209 ) ) ;
#1648=CARTESIAN_POINT ( 'NONE',  ( -50.00000000000000000, 25.78125000068279959, 0.000000000000000000 ) ) ;
#1653=CARTESIAN_POINT ( 'NONE',  ( 15.45084971874736723, 43.18125000068280173, -47.55282581475768211 ) ) ;
#1663=DIRECTION ( 'NONE',  ( 0.000000000000000000, 1.000000000000000000, 0.000000000000000000 ) ) ;
#1673=CARTESIAN_POINT ( 'NONE',  ( 15.45084971874736723, 47.40000000000000568, -47.55282581475768211 ) ) ;
#1675=CARTESIAN_POINT ( 'NONE',  ( -30.81806926056963292, 31.62187500034140086, -42.41743335407646498 ) ) ;
#1678=CARTESIAN_POINT ( 'NONE',  ( -40.34137639590981905, 29.65937500034139518, -29.30972558990011478 ) ) ;
#1680=CARTESIAN_POINT ( 'NONE',  ( 7.919222016226758143, 38.55125428154684641, 50.00000000000000711 ) ) ;
#1682=EDGE_CURVE ( 'NONE', #10619, #5249, #15486, .T. ) ;
#1692=CARTESIAN_POINT ( 'NONE',  ( 49.86468353125000164, 32.92187500034139447, -6.106662507704105588E-15 ) ) ;
#1693=CARTESIAN_POINT ( 'NONE',  ( -15.40903463028480580, 36.25937500034140015, 47.42413220539094709 ) ) ;
#1694=CARTESIAN_POINT ( 'NONE',  ( -3.111920190527341144E-15, 25.50000000000000355, -50.00000000000000000 ) ) ;
#1696=CARTESIAN_POINT ( 'NONE',  ( 49.99999999999999289, 22.88125000068280102, -16.24598481164532160 ) ) ;
#1698=( BOUNDED_CURVE ( )  B_SPLINE_CURVE ( 2, ( #7324, #12395, #4842, #4667, #14870, #8635, #5996, #13547, #12299, #13623, #16135, #10975, #901 ),
 .UNSPECIFIED., .F., .F. ) 
 B_SPLINE_CURVE_WITH_KNOTS ( ( 3, 2, 2, 2, 2, 2, 3 ),
 ( 0.05000000000000000278, 0.05333333333333333676, 0.05999999999999999778, 0.06666666666666666574, 0.07333333333333333370, 0.08000000000000000167, 0.08333333333333334259 ),
 .UNSPECIFIED. ) 
 CURVE ( )  GEOMETRIC_REPRESENTATION_ITEM ( )  RATIONAL_B_SPLINE_CURVE ( ( 0.9755282581475768211, 0.9755282581475768211, 1.000000000000000000, 0.9510565162951535312, 1.000000000000000000, 0.9510565162951535312, 1.000000000000000000, 0.9510565162951535312, 1.000000000000000000, 0.9510565162951535312, 1.000000000000000000, 0.9755282581475767101, 0.9755282581475768211 ) ) 
 REPRESENTATION_ITEM ( '' )  );
#1699=CARTESIAN_POINT ( 'NONE',  ( -49.86468353125000164, 25.92187500034139802, 0.000000000000000000 ) ) ;
#1701=CARTESIAN_POINT ( 'NONE',  ( -7.919222016226816763, 27.33250428222964246, -49.99999999999999289 ) ) ;
#1709=CARTESIAN_POINT ( 'NONE',  ( 9.631387414534489405E-15, 26.35937500034140157, 52.43083105670540789 ) ) ;
#1712=CARTESIAN_POINT ( 'NONE',  ( 49.86468353125000164, 38.92187500034139447, -6.106662507704105588E-15 ) ) ;
#1714=CARTESIAN_POINT ( 'NONE',  ( -40.34137639590981195, 44.12187500034139731, 29.30972558990012189 ) ) ;
#1719=ORIENTED_EDGE ( 'NONE', *, *, #3682, .F. ) ;
#1724=FACE_OUTER_BOUND ( 'NONE', #8544, .T. ) ;
#1727=CARTESIAN_POINT ( 'NONE',  ( -15.45084971874737256, 25.60000000000000142, -47.55282581475767500 ) ) ;
#1728=CARTESIAN_POINT ( 'NONE',  ( 49.86468353124999453, 42.95937500034139589, -16.20201782572376459 ) ) ;
#1729=CARTESIAN_POINT ( 'NONE',  ( -40.45084971874737789, 31.58125000068280031, -29.38926261462365730 ) ) ;
#1730=DIRECTION ( 'NONE',  ( 0.000000000000000000, 0.000000000000000000, 1.000000000000000000 ) ) ;
#1732=EDGE_CURVE ( 'NONE', #10576, #11191, #4881, .T. ) ;
#1734=CARTESIAN_POINT ( 'NONE',  ( 30.90169943749475578, 36.48125000068279888, 42.53254041760200010 ) ) ;
#1740=EDGE_CURVE ( 'NONE', #2027, #9264, #14507, .T. ) ;
#1742=ORIENTED_EDGE ( 'NONE', *, *, #14552, .F. ) ;
#1753=CARTESIAN_POINT ( 'NONE',  ( -3.111920190527341144E-15, 27.50000000000000000, -50.00000000000000000 ) ) ;
#1756=CARTESIAN_POINT ( 'NONE',  ( 0.5792196722693350175, 4.999999999999996447, 99.11836509645773674 ) ) ;
#1761=CARTESIAN_POINT ( 'NONE',  ( 49.86468353124999453, 34.95937500034138878, -16.20201782572376459 ) ) ;
#1777=CARTESIAN_POINT ( 'NONE',  ( 30.81806926056964002, 36.62187500034139731, 42.41743335407647209 ) ) ;
#1778=CARTESIAN_POINT ( 'NONE',  ( -30.81806926056962226, 38.15937500034139163, 42.41743335407647209 ) ) ;
#1781=EDGE_CURVE ( 'NONE', #842, #15320, #11663, .T. ) ;
#1782=CARTESIAN_POINT ( 'NONE',  ( -49.99999999999999289, 23.88125000068279746, 16.24598481164533226 ) ) ;
#1784=CARTESIAN_POINT ( 'NONE',  ( 40.34137639590981905, 24.72187500034139873, 29.30972558990010768 ) ) ;
#1788=VERTEX_POINT ( 'NONE', #12128 ) ;
#1794=CARTESIAN_POINT ( 'NONE',  ( -40.34137639590981195, 24.05937500034139731, 29.30972558990012189 ) ) ;
#1796=( BOUNDED_CURVE ( )  B_SPLINE_CURVE ( 2, ( #14890, #4862, #13730, #11174, #7424, #9759, #2343, #8571, #762, #8418, #16229, #10915, #13642 ),
 .UNSPECIFIED., .F., .F. ) 
 B_SPLINE_CURVE_WITH_KNOTS ( ( 3, 2, 2, 2, 2, 2, 3 ),
 ( 0.01666666666666666990, 0.02000000000000000042, 0.02666666666666666838, 0.03333333333333333287, 0.04000000000000000083, 0.04666666666666667573, 0.05000000000000000278 ),
 .UNSPECIFIED. ) 
 CURVE ( )  GEOMETRIC_REPRESENTATION_ITEM ( )  RATIONAL_B_SPLINE_CURVE ( ( 0.9755282581475768211, 0.9755282581475768211, 1.000000000000000000, 0.9510565162951535312, 1.000000000000000000, 0.9510565162951535312, 1.000000000000000000, 0.9510565162951535312, 1.000000000000000000, 0.9510565162951535312, 1.000000000000000000, 0.9755282581475768211, 0.9755282581475768211 ) ) 
 REPRESENTATION_ITEM ( '' )  );
#1797=CARTESIAN_POINT ( 'NONE',  ( -49.86468353124999453, 39.82187500034140015, -16.20201782572375393 ) ) ;
#1800=CARTESIAN_POINT ( 'NONE',  ( -15.40903463028481646, 45.52187500034139589, -47.42413220539093999 ) ) ;
#1808=CARTESIAN_POINT ( 'NONE',  ( 49.99999999999999289, 38.88125000068279036, -16.24598481164532160 ) ) ;
#1810=CARTESIAN_POINT ( 'NONE',  ( -50.00000000000000000, 28.00000000000000000, 0.000000000000000000 ) ) ;
#1811=CARTESIAN_POINT ( 'NONE',  ( 30.81806926056962936, 41.15937500034139873, -42.41743335407647209 ) ) ;
#1816=CARTESIAN_POINT ( 'NONE',  ( -40.45084971874737079, 33.98125000068279888, 29.38926261462367151 ) ) ;
#1817=CARTESIAN_POINT ( 'NONE',  ( 1.293669679204937499E-13, 37.50000000000000711, -50.00000000000000000 ) ) ;
#1821=ORIENTED_EDGE ( 'NONE', *, *, #7453, .T. ) ;
#1823=CARTESIAN_POINT ( 'NONE',  ( 7.919222016226854954, 42.55125428154684641, 49.99999999999998579 ) ) ;
#1829=FACE_OUTER_BOUND ( 'NONE', #13462, .T. ) ;
#1832=CARTESIAN_POINT ( 'NONE',  ( -15.45084971874737256, 37.38125000068279746, -47.55282581475767500 ) ) ;
#1833=CARTESIAN_POINT ( 'NONE',  ( 50.00000000000000000, 47.00000000000000000, -6.123233995736766085E-15 ) ) ;
#1834=CARTESIAN_POINT ( 'NONE',  ( -46.96694430692108568, 19.99999999999999645, 16.75173377947249165 ) ) ;
#1835=CARTESIAN_POINT ( 'NONE',  ( 15.40903463028481113, 23.32187500034139660, -47.42413220539094709 ) ) ;
#1838=CARTESIAN_POINT ( 'NONE',  ( 30.81806926056964002, 26.55937500034139376, 42.41743335407647209 ) ) ;
#1849=CARTESIAN_POINT ( 'NONE',  ( 15.40903463028482356, 32.52187500034139589, 47.42413220539093999 ) ) ;
#1850=CARTESIAN_POINT ( 'NONE',  ( -3.210462471511496205E-15, 35.35937500034140157, -52.43083105670540789 ) ) ;
#1854=CARTESIAN_POINT ( 'NONE',  ( 30.90169943749475578, 20.48125000068279178, 42.53254041760200010 ) ) ;
#1856=CARTESIAN_POINT ( 'NONE',  ( 40.45084971874737079, 49.20000000000000284, -29.38926261462366440 ) ) ;
#1858=ORIENTED_EDGE ( 'NONE', *, *, #1565, .T. ) ;
#1867=CARTESIAN_POINT ( 'NONE',  ( -30.81806926056962226, 28.15937500034139518, 42.41743335407647919 ) ) ;
#1870=CARTESIAN_POINT ( 'NONE',  ( 40.45084971874737789, 34.80000000000000426, 29.38926261462365375 ) ) ;
#1872=CARTESIAN_POINT ( 'NONE',  ( -15.40903463028481646, 43.52187500034139589, -47.42413220539093999 ) ) ;
#1877=PRODUCT ( 'container base & motor', 'container base & motor', '', ( #788 ) ) ;
#1881=DIRECTION ( 'NONE',  ( -0.000000000000000000, 1.000000000000000000, -0.000000000000000000 ) ) ;
#1884=LINE ( 'NONE', #10638, #2647 ) ;
#1885=CARTESIAN_POINT ( 'NONE',  ( 30.90169943749475578, 20.69999999999999574, 42.53254041760200010 ) ) ;
#1886=CARTESIAN_POINT ( 'NONE',  ( 40.34137639590981905, 44.65937500034139163, 29.30972558990010768 ) ) ;
#1895=ORIENTED_EDGE ( 'NONE', *, *, #7141, .F. ) ;
#1896=ORIENTED_EDGE ( 'NONE', *, *, #13712, .F. ) ;
#1904=CARTESIAN_POINT ( 'NONE',  ( 15.45084971874736723, 23.40000000000000213, -47.55282581475768211 ) ) ;
#1907=CARTESIAN_POINT ( 'NONE',  ( -15.45084971874736368, 32.39999999999999858, 47.55282581475768211 ) ) ;
#1908=CARTESIAN_POINT ( 'NONE',  ( 8.850089126414076190, 7.391638089289761737, 98.30041665922365723 ) ) ;
#1909=CARTESIAN_POINT ( 'NONE',  ( -45.47188453826096577, 20.00000000000001066, 20.46517872429623353 ) ) ;
#1910=CARTESIAN_POINT ( 'NONE',  ( 9.631387414534489405E-15, 22.42187500034139802, 52.43083105670540789 ) ) ;
#1913=CARTESIAN_POINT ( 'NONE',  ( 15.40903463028481113, 27.25937500034139660, -47.42413220539094709 ) ) ;
#1920=ORIENTED_EDGE ( 'NONE', *, *, #7912, .T. ) ;
#1925=ADVANCED_FACE ( 'NONE', ( #2470 ), #2388, .F. ) ;
#1927=CARTESIAN_POINT ( 'NONE',  ( -30.81806926056963292, 31.62187500034139731, -42.41743335407647209 ) ) ;
#1928=CARTESIAN_POINT ( 'NONE',  ( 49.86468353125000164, 36.85937500034139447, -6.106662507704105588E-15 ) ) ;
#1934=CARTESIAN_POINT ( 'NONE',  ( -49.86468353124999453, 43.75937500034140015, -16.20201782572375393 ) ) ;
#1936=CARTESIAN_POINT ( 'NONE',  ( -49.86468353124999453, 24.02187500034139589, 16.20201782572377525 ) ) ;
#1947=CARTESIAN_POINT ( 'NONE',  ( 30.81806926056964002, 46.62187500034140442, 42.41743335407647209 ) ) ;
#1949=CARTESIAN_POINT ( 'NONE',  ( 49.99999999999999289, 37.10000000000000142, -16.24598481164532160 ) ) ;
#1951=CARTESIAN_POINT ( 'NONE',  ( 30.81806926056964002, 40.62187500034139731, 42.41743335407647209 ) ) ;
#1953=ORIENTED_EDGE ( 'NONE', *, *, #1542, .T. ) ;
#1956=ORIENTED_EDGE ( 'NONE', *, *, #8034, .T. ) ;
#1957=EDGE_LOOP ( 'NONE', ( #12978, #13764, #4666, #14845 ) ) ;
#1958=CARTESIAN_POINT ( 'NONE',  ( 2.600676159226421000E-13, 23.50000000000000000, -49.99999999999999289 ) ) ;
#1962=DIRECTION ( 'NONE',  ( -0.000000000000000000, 1.000000000000000000, -0.000000000000000000 ) ) ;
#1963=CARTESIAN_POINT ( 'NONE',  ( 49.86468353125000164, 40.85937500034139447, -6.106662507704105588E-15 ) ) ;
#1974=COLOUR_RGB ( '', 0.08235294, 0.09019608, 0.10196078) ;
#1981=DIRECTION ( 'NONE',  ( 0.000000000000000000, 0.000000000000000000, 1.000000000000000000 ) ) ;
#1982=PRESENTATION_STYLE_ASSIGNMENT (( #14868 ) ) ;
#1984=CARTESIAN_POINT ( 'NONE',  ( 0.000000000000000000, 20.00000000000000355, 0.000000000000000000 ) ) ;
#1986=CARTESIAN_POINT ( 'NONE',  ( -17.50000000000000000, 22.50000000000000000, 102.0000000000000142 ) ) ;
#1988=FACE_OUTER_BOUND ( 'NONE', #11505, .T. ) ;
#1994=B_SPLINE_CURVE_WITH_KNOTS ( 'NONE', 3,
 ( #13386, #752, #5839, #10905 ),
 .UNSPECIFIED., .F., .F.,
 ( 4, 4 ),
 ( 0.000000000000000000, 0.01241723871866209916 ),
 .UNSPECIFIED. ) ;
#1995=CARTESIAN_POINT ( 'NONE',  ( -3.210462471511496205E-15, 21.42187500034139802, -52.43083105670540789 ) ) ;
#1998=CARTESIAN_POINT ( 'NONE',  ( 40.34137639590981195, 23.05937500034139731, -29.30972558990011834 ) ) ;
#2003=CARTESIAN_POINT ( 'NONE',  ( 15.45084971874736723, 45.40000000000000568, -47.55282581475768211 ) ) ;
#2004=ORIENTED_EDGE ( 'NONE', *, *, #16114, .T. ) ;
#2006=FACE_OUTER_BOUND ( 'NONE', #5801, .T. ) ;
#2009=ADVANCED_FACE ( 'NONE', ( #15434 ), #3605, .F. ) ;
#2010=DIRECTION ( 'NONE',  ( 0.000000000000000000, 0.000000000000000000, 1.000000000000000000 ) ) ;
#2013=CARTESIAN_POINT ( 'NONE',  ( 49.86468353125000164, 28.92187500034139802, -6.106662507704105588E-15 ) ) ;
#2014=CARTESIAN_POINT ( 'NONE',  ( 49.86468353124999453, 28.95937500034139589, -16.20201782572376104 ) ) ;
#2021=CARTESIAN_POINT ( 'NONE',  ( -15.40903463028480580, 48.25937500034140015, 47.42413220539094709 ) ) ;
#2023=CARTESIAN_POINT ( 'NONE',  ( 15.40903463028482356, 20.52187500034139589, 47.42413220539093999 ) ) ;
#2027=VERTEX_POINT ( 'NONE', #725 ) ;
#2032=( BOUNDED_CURVE ( )  B_SPLINE_CURVE ( 2, ( #4354, #15570, #6864, #15480, #15169, #432, #7922, #1289, #346, #10507, #10118, #1680, #14463 ),
 .UNSPECIFIED., .F., .F. ) 
 B_SPLINE_CURVE_WITH_KNOTS ( ( 3, 2, 2, 2, 2, 2, 3 ),
 ( 0.3500000000000000333, 0.3533333333333333326, 0.3599999999999999867, 0.3666666666666666408, 0.3733333333333333504, 0.3800000000000000044, 0.3833333333333333592 ),
 .UNSPECIFIED. ) 
 CURVE ( )  GEOMETRIC_REPRESENTATION_ITEM ( )  RATIONAL_B_SPLINE_CURVE ( ( 0.9755282581475768211, 0.9755282581475770431, 1.000000000000000000, 0.9510565162951535312, 1.000000000000000000, 0.9510565162951535312, 1.000000000000000000, 0.9510565162951535312, 1.000000000000000000, 0.9510565162951535312, 1.000000000000000000, 0.9755282581475765991, 0.9755282581475768211 ) ) 
 REPRESENTATION_ITEM ( '' )  );
#2033=CARTESIAN_POINT ( 'NONE',  ( 7.919222016226758143, 40.33250428222964246, 50.00000000000000711 ) ) ;
#2035=CARTESIAN_POINT ( 'NONE',  ( -40.34137639590981195, 20.05937500034139731, 29.30972558990012189 ) ) ;
#2036=CARTESIAN_POINT ( 'NONE',  ( 0.000000000000000000, 20.00000000000000355, 50.00000000000000000 ) ) ;
#2037=EDGE_CURVE ( 'NONE', #16127, #5607, #11137, .T. ) ;
#2040=CARTESIAN_POINT ( 'NONE',  ( 50.00000000000000000, 37.00000000000000711, -6.123233995736766085E-15 ) ) ;
#2042=CARTESIAN_POINT ( 'NONE',  ( -49.86468353124999453, 38.02187500034140299, 16.20201782572377525 ) ) ;
#2043=LINE ( 'NONE', #7132, #15998 ) ;
#2055=CARTESIAN_POINT ( 'NONE',  ( 15.45084971874736723, 37.18125000068280173, -47.55282581475768211 ) ) ;
#2056=CARTESIAN_POINT ( 'NONE',  ( 9.631387414534489405E-15, 36.35937500034140157, 52.43083105670540789 ) ) ;
#2057=CARTESIAN_POINT ( 'NONE',  ( 15.40903463028482356, 46.45937500034139589, 47.42413220539093999 ) ) ;
#2061=DIRECTION ( 'NONE',  ( 0.000000000000000000, 0.000000000000000000, 1.000000000000000000 ) ) ;
#2072=( NAMED_UNIT ( * ) SI_UNIT ( $, .STERADIAN. ) SOLID_ANGLE_UNIT ( ) );
#2074=CARTESIAN_POINT ( 'NONE',  ( 0.000000000000000000, 0.000000000000000000, 0.000000000000000000 ) ) ;
#2080=CARTESIAN_POINT ( 'NONE',  ( -15.45084971874737256, 31.60000000000000142, -47.55282581475767500 ) ) ;
#2081=CARTESIAN_POINT ( 'NONE',  ( -46.06840506420015657, 20.00000000000000355, 19.08445694769762113 ) ) ;
#2082=CARTESIAN_POINT ( 'NONE',  ( 30.81806926056962936, 25.22187500034139873, -42.41743335407646498 ) ) ;
#2085=CARTESIAN_POINT ( 'NONE',  ( 49.86468353124999453, 26.95937500034139944, -16.20201782572376459 ) ) ;
#2094=CARTESIAN_POINT ( 'NONE',  ( -2.547328955960238000E-13, 34.50000000000000000, 49.99999999999999289 ) ) ;
#2097=CARTESIAN_POINT ( 'NONE',  ( 49.86468353124999453, 29.02187500034139234, -16.20201782572376459 ) ) ;
#2098=CARTESIAN_POINT ( 'NONE',  ( -3.210462471511496205E-15, 29.35937500034139802, -52.43083105670540789 ) ) ;
#2099=CARTESIAN_POINT ( 'NONE',  ( -49.99999999999999289, 35.89999999999999858, -16.24598481164531449 ) ) ;
#2102=CARTESIAN_POINT ( 'NONE',  ( -40.34137639590981905, 47.65937500034139873, -29.30972558990011478 ) ) ;
#2104=CARTESIAN_POINT ( 'NONE',  ( -40.34137639590981195, 20.12187500034139731, 29.30972558990012189 ) ) ;
#2113=CARTESIAN_POINT ( 'NONE',  ( -30.81806926056963292, 45.62187500034139020, -42.41743335407647209 ) ) ;
#2116=CARTESIAN_POINT ( 'NONE',  ( -30.90169943749474868, 33.48125000068279888, -42.53254041760200721 ) ) ;
#2117=CARTESIAN_POINT ( 'NONE',  ( -49.86468353125000164, 41.92187500034139447, 0.000000000000000000 ) ) ;
#2130=CARTESIAN_POINT ( 'NONE',  ( 30.90169943749473802, 37.08125000068280031, -42.53254041760200721 ) ) ;
#2131=CARTESIAN_POINT ( 'NONE',  ( -3.210462471511496205E-15, 37.35937500034139447, -52.43083105670540789 ) ) ;
#2132=CARTESIAN_POINT ( 'NONE',  ( -49.86468353124999453, 47.95937500034138878, 16.20201782572377169 ) ) ;
#2133=CARTESIAN_POINT ( 'NONE',  ( 7.919222016226693306, 24.55125428154684286, 50.00000000000003553 ) ) ;
#2134=ADVANCED_FACE ( 'NONE', ( #14764 ), #13445, .F. ) ;
#2138=DIRECTION ( 'NONE',  ( -0.000000000000000000, 1.000000000000000000, -0.000000000000000000 ) ) ;
#2148=CARTESIAN_POINT ( 'NONE',  ( -30.90169943749473447, 40.30000000000000426, 42.53254041760200721 ) ) ;
#2149=CARTESIAN_POINT ( 'NONE',  ( 2.978552182361884590E-14, 47.28125000068279604, -50.00000000000000000 ) ) ;
#2153=CARTESIAN_POINT ( 'NONE',  ( -30.90169943749473447, 20.30000000000000071, 42.53254041760200721 ) ) ;
#2155=DIRECTION ( 'NONE',  ( 0.000000000000000000, 0.000000000000000000, 1.000000000000000000 ) ) ;
#2158=CARTESIAN_POINT ( 'NONE',  ( 0.000000000000000000, 0.000000000000000000, 0.000000000000000000 ) ) ;
#2159=CARTESIAN_POINT ( 'NONE',  ( -45.18727525474225359, 20.00000000000001066, 21.08615623785947690 ) ) ;
#2160=CARTESIAN_POINT ( 'NONE',  ( -49.99999999999999289, 47.68125000068280173, -16.24598481164531449 ) ) ;
#2163=CARTESIAN_POINT ( 'NONE',  ( 30.81806926056962936, 27.15937500034139163, -42.41743335407647209 ) ) ;
#2174=CARTESIAN_POINT ( 'NONE',  ( 30.81806926056964002, 28.62187500034140086, 42.41743335407647209 ) ) ;
#2175=CARTESIAN_POINT ( 'NONE',  ( -49.86468353125000164, 27.85937500034139447, 0.000000000000000000 ) ) ;
#2176=CARTESIAN_POINT ( 'NONE',  ( -1.240322475938754499E-13, 36.50000000000000711, 50.00000000000000000 ) ) ;
#2179=CARTESIAN_POINT ( 'NONE',  ( 40.34137639590981905, 46.65937500034139873, 29.30972558990010768 ) ) ;
#2182=CARTESIAN_POINT ( 'NONE',  ( 15.40903463028482356, 22.52187500034139589, 47.42413220539093999 ) ) ;
#2192=CARTESIAN_POINT ( 'NONE',  ( -49.86468353124999453, 48.02187500034139589, 16.20201782572377525 ) ) ;
#2196=CARTESIAN_POINT ( 'NONE',  ( 15.45084971874736723, 35.18125000068280173, -47.55282581475768211 ) ) ;
#2197=CARTESIAN_POINT ( 'NONE',  ( 49.86468353124999453, 39.02187500034138878, -16.20201782572376459 ) ) ;
#2204=ORIENTED_EDGE ( 'NONE', *, *, #5294, .T. ) ;
#2206=CARTESIAN_POINT ( 'NONE',  ( -30.90169943749473447, 40.08125000068279320, 42.53254041760200721 ) ) ;
#2208=FACE_BOUND ( 'NONE', #695, .T. ) ;
#2210=CARTESIAN_POINT ( 'NONE',  ( -49.86468353124999453, 39.75937500034139305, -16.20201782572375393 ) ) ;
#2211=CARTESIAN_POINT ( 'NONE',  ( -49.86468353124999453, 47.75937500034139305, -16.20201782572375393 ) ) ;
#2213=AXIS2_PLACEMENT_3D ( 'NONE', #13775, #1302, #15180 ) ;
#2216=EDGE_CURVE ( 'NONE', #9078, #10576, #10369, .T. ) ;
#2220=( BOUNDED_CURVE ( )  B_SPLINE_CURVE ( 2, ( #15889, #7001, #5757, #3332, #4512, #8242, #10826, #2239, #14876, #831, #14623, #12056, #6003 ),
 .UNSPECIFIED., .F., .T. ) 
 B_SPLINE_CURVE_WITH_KNOTS ( ( 3, 2, 2, 2, 2, 2, 3 ),
 ( 0.05000000000000000278, 0.05333333333333333676, 0.05999999999999999778, 0.06666666666666666574, 0.07333333333333333370, 0.08000000000000000167, 0.08333333333333334259 ),
 .UNSPECIFIED. ) 
 CURVE ( )  GEOMETRIC_REPRESENTATION_ITEM ( )  RATIONAL_B_SPLINE_CURVE ( ( 0.9755282581475768211, 0.9755282581475768211, 1.000000000000000000, 0.9510565162951535312, 1.000000000000000000, 0.9510565162951535312, 1.000000000000000000, 0.9510565162951535312, 1.000000000000000000, 0.9510565162951535312, 1.000000000000000000, 0.9755282581475767101, 0.9755282581475768211 ) ) 
 REPRESENTATION_ITEM ( '' )  );
#2222=EDGE_LOOP ( 'NONE', ( #11670, #9442, #4893 ) ) ;
#2226=EDGE_CURVE ( 'NONE', #4835, #13275, #13753, .T. ) ;
#2234=ADVANCED_FACE ( 'NONE', ( #9878 ), #7627, .F. ) ;
#2235=CARTESIAN_POINT ( 'NONE',  ( -13.93607900078482054, 11.90003901379968632, 96.90546041726973669 ) ) ;
#2239=CARTESIAN_POINT ( 'NONE',  ( -49.99999999999999289, 47.89999999999999858, -16.24598481164531449 ) ) ;
#2240=CARTESIAN_POINT ( 'NONE',  ( 15.45084971874737789, 46.60000000000000142, 47.55282581475767500 ) ) ;
#2242=CARTESIAN_POINT ( 'NONE',  ( -49.99999999999999289, 43.88125000068279746, 16.24598481164533226 ) ) ;
#2259=CARTESIAN_POINT ( 'NONE',  ( 49.86468353124999453, 23.02187500034139944, -16.20201782572376459 ) ) ;
#2260=CARTESIAN_POINT ( 'NONE',  ( -15.40903463028480580, 30.25937500034140015, 47.42413220539094709 ) ) ;
#2261=DIRECTION ( 'NONE',  ( -1.000000000000000000, 0.000000000000000000, 0.000000000000000000 ) ) ;
#2262=CARTESIAN_POINT ( 'NONE',  ( 40.34137639590981905, 36.72187500034139163, 29.30972558990010768 ) ) ;
#2265=CARTESIAN_POINT ( 'NONE',  ( 49.86468353125001585, 36.75937500034138594, 16.20201782572375038 ) ) ;
#2268=CARTESIAN_POINT ( 'NONE',  ( -30.90169943749474868, 45.70000000000000995, -42.53254041760200721 ) ) ;
#2270=MECHANICAL_DESIGN_GEOMETRIC_PRESENTATION_REPRESENTATION('',(#7583),#14469);
#2279=AXIS2_PLACEMENT_3D ( 'NONE', #1623, #4606, #2010 ) ;
#2281=CARTESIAN_POINT ( 'NONE',  ( 7.919222016226875382, 41.22999571913594963, -49.99999999999997158 ) ) ;
#2282=CARTESIAN_POINT ( 'NONE',  ( 30.81806926056962936, 47.22187500034139873, -42.41743335407647209 ) ) ;
#2285=CARTESIAN_POINT ( 'NONE',  ( -15.45084971874737256, 35.38125000068279746, -47.55282581475767500 ) ) ;
#2286=CARTESIAN_POINT ( 'NONE',  ( 49.86468353125001585, 36.82187500034140015, 16.20201782572375038 ) ) ;
#2298=CARTESIAN_POINT ( 'NONE',  ( -50.00000000000000000, 21.78125000068279959, 0.000000000000000000 ) ) ;
#2299=CARTESIAN_POINT ( 'NONE',  ( -49.99999999999999289, 23.88125000068279746, 16.24598481164533226 ) ) ;
#2300=AXIS2_PLACEMENT_3D ( 'NONE', #9631, #13368, #2061 ) ;
#2302=VECTOR ( 'NONE', #90, 1000.000000000000000 ) ;
#2303=CARTESIAN_POINT ( 'NONE',  ( -3.210462471511496205E-15, 39.35937500034138736, -52.43083105670540789 ) ) ;
#2304=CARTESIAN_POINT ( 'NONE',  ( -49.86468353124999453, 41.95937500034139589, 16.20201782572377169 ) ) ;
#2311=CARTESIAN_POINT ( 'NONE',  ( -50.00000000000000000, 42.00000000000000000, 0.000000000000000000 ) ) ;
#2317=ORIENTED_EDGE ( 'NONE', *, *, #6640, .F. ) ;
#2320=SURFACE_STYLE_FILL_AREA ( #4840 ) ;
#2321=VERTEX_POINT ( 'NONE', #1211 ) ;
#2324=CARTESIAN_POINT ( 'NONE',  ( -15.19004016089065701, 13.79141621452552258, 96.37893023295546868 ) ) ;
#2333=CARTESIAN_POINT ( 'NONE',  ( 50.00000000000000000, 48.78125000068279604, -6.123233995736766085E-15 ) ) ;
#2334=( BOUNDED_CURVE ( )  B_SPLINE_CURVE ( 2, ( #14307, #11815, #6926, #501, #2755, #10415, #14220, #1514, #9164, #4092, #2845, #11980, #14457 ),
 .UNSPECIFIED., .F., .T. ) 
 B_SPLINE_CURVE_WITH_KNOTS ( ( 3, 2, 2, 2, 2, 2, 3 ),
 ( 0.6500000000000000222, 0.6533333333333333215, 0.6600000000000000311, 0.6666666666666666297, 0.6733333333333333393, 0.6800000000000000488, 0.6833333333333333481 ),
 .UNSPECIFIED. ) 
 CURVE ( )  GEOMETRIC_REPRESENTATION_ITEM ( )  RATIONAL_B_SPLINE_CURVE ( ( 0.9755282581475768211, 0.9755282581475771542, 1.000000000000000000, 0.9510565162951535312, 1.000000000000000000, 0.9510565162951535312, 1.000000000000000000, 0.9510565162951535312, 1.000000000000000000, 0.9510565162951535312, 1.000000000000000000, 0.9755282581475768211, 0.9755282581475768211 ) ) 
 REPRESENTATION_ITEM ( '' )  );
#2337=CARTESIAN_POINT ( 'NONE',  ( -49.86468353124999453, 19.95937500034138878, 16.20201782572377525 ) ) ;
#2342=ORIENTED_EDGE ( 'NONE', *, *, #15755, .T. ) ;
#2343=CARTESIAN_POINT ( 'NONE',  ( 50.00000000000000000, 49.00000000000000000, -6.123233995736766085E-15 ) ) ;
#2350=CARTESIAN_POINT ( 'NONE',  ( -40.34137639590981195, 20.12187500034139731, 29.30972558990012189 ) ) ;
#2351=CARTESIAN_POINT ( 'NONE',  ( -49.86468353125000164, 31.85937500034139447, 0.000000000000000000 ) ) ;
#2353=CARTESIAN_POINT ( 'NONE',  ( 9.631387414534489405E-15, 36.42187500034139447, 52.43083105670540789 ) ) ;
#2355=CARTESIAN_POINT ( 'NONE',  ( 9.657523855033129090E-15, 36.50000000000000711, 52.57311121191334990 ) ) ;
#2356=CARTESIAN_POINT ( 'NONE',  ( -49.86468353124999453, 39.95937500034139589, 16.20201782572377525 ) ) ;
#2359=CARTESIAN_POINT ( 'NONE',  ( -15.45084971874736368, 44.39999999999999858, 47.55282581475768211 ) ) ;
#2362=EDGE_LOOP ( 'NONE', ( #6480, #9687, #1391, #13902 ) ) ;
#2365=CARTESIAN_POINT ( 'NONE',  ( 0.000000000000000000, 0.000000000000000000, 0.000000000000000000 ) ) ;
#2366=FACE_OUTER_BOUND ( 'NONE', #5595, .T. ) ;
#2367=CARTESIAN_POINT ( 'NONE',  ( -15.40903463028481646, 39.52187500034139589, -47.42413220539093999 ) ) ;
#2370=CARTESIAN_POINT ( 'NONE',  ( 50.00000000000000000, 24.78125000068279959, -6.123233995736766085E-15 ) ) ;
#2372=CARTESIAN_POINT ( 'NONE',  ( 15.40903463028482356, 34.52187500034140299, 47.42413220539093999 ) ) ;
#2376=ORIENTED_EDGE ( 'NONE', *, *, #1542, .F. ) ;
#2381=CARTESIAN_POINT ( 'NONE',  ( -7.919222016226934890, 22.22999571913594963, 49.99999999999996447 ) ) ;
#2383=CARTESIAN_POINT ( 'NONE',  ( 49.86468353124999453, 32.95937500034138168, -16.20201782572376459 ) ) ;
#2388=CYLINDRICAL_SURFACE ( 'NONE', #6073, 50.00000000000000000 ) ;
#2399=CARTESIAN_POINT ( 'NONE',  ( 7.919222016226809657, 35.22999571913594963, -50.00000000000000000 ) ) ;
#2403=DIRECTION ( 'NONE',  ( -0.000000000000000000, 1.000000000000000000, -0.000000000000000000 ) ) ;
#2404=CARTESIAN_POINT ( 'NONE',  ( -7.827029700262156275, 6.837221630493822921, 98.48522124286309065 ) ) ;
#2410=CARTESIAN_POINT ( 'NONE',  ( 9.657523855033129090E-15, 48.28125000068279604, 52.57311121191334990 ) ) ;
#2414=CARTESIAN_POINT ( 'NONE',  ( 7.513064459987437071E-14, 42.28125000068280315, 50.00000000000000000 ) ) ;
#2418=B_SPLINE_CURVE_WITH_KNOTS ( 'NONE', 3,
 ( #11442, #4120, #10281, #9029, #14084, #14166, #6631, #1287, #114, #12601, #280, #6294, #7776, #15418, #12847, #1367, #7698, #2700, #9107, #9192, #7528, #3874, #1450, #6378, #6542, #2450 ),
 .UNSPECIFIED., .F., .F.,
 ( 4, 2, 2, 2, 2, 2, 2, 2, 2, 2, 2, 2, 4 ),
 ( 0.04214985370082251215, 0.04558239031788638429, 0.04729865862641832036, 0.04901492693495026337, 0.05244746355201414245, 0.05416373186054608546, 0.05588000016907802847, 0.05759626847760997148, 0.05931253678614191449, 0.06274507340320578663, 0.06446134171173772964, 0.06617761002026967265, 0.06961014663733354479 ),
 .UNSPECIFIED. ) ;
#2426=CARTESIAN_POINT ( 'NONE',  ( -49.86468353124999453, 23.82187500034139305, -16.20201782572375393 ) ) ;
#2427=CARTESIAN_POINT ( 'NONE',  ( -49.86468353124999453, 23.75937500034139660, -16.20201782572375393 ) ) ;
#2429=CARTESIAN_POINT ( 'NONE',  ( -15.40903463028481646, 37.52187500034139589, -47.42413220539093999 ) ) ;
#2430=DIRECTION ( 'NONE',  ( -0.000000000000000000, 1.000000000000000000, -0.000000000000000000 ) ) ;
#2431=CARTESIAN_POINT ( 'NONE',  ( 30.90169943749474157, 35.30000000000000426, -42.53254041760200721 ) ) ;
#2432=CARTESIAN_POINT ( 'NONE',  ( -3.210462471511496205E-15, 39.35937500034138736, -52.43083105670540789 ) ) ;
#2434=ADVANCED_FACE ( 'NONE', ( #7168 ), #10980, .F. ) ;
#2435=CARTESIAN_POINT ( 'NONE',  ( -15.45084971874737256, 43.60000000000000142, -47.55282581475767500 ) ) ;
#2441=EDGE_CURVE ( 'NONE', #12025, #9639, #13383, .T. ) ;
#2442=CARTESIAN_POINT ( 'NONE',  ( -50.00000000000000000, 34.00000000000000000, 0.000000000000000000 ) ) ;
#2446=CARTESIAN_POINT ( 'NONE',  ( -30.81806926056962226, 40.22187500034139873, 42.41743335407647919 ) ) ;
#2449=CARTESIAN_POINT ( 'NONE',  ( 50.00000000000000711, 26.68125000068279462, 16.24598481164530739 ) ) ;
#2450=CARTESIAN_POINT ( 'NONE',  ( -2.317185599438165467E-15, 40.00000000000004974, 92.94692077166139654 ) ) ;
#2451=EDGE_CURVE ( 'NONE', #9157, #2703, #4847, .T. ) ;
#2452=CARTESIAN_POINT ( 'NONE',  ( -49.86468353124999453, 31.82187500034139305, -16.20201782572375393 ) ) ;
#2461=CARTESIAN_POINT ( 'NONE',  ( -15.45084971874736368, 24.40000000000000213, 47.55282581475768211 ) ) ;
#2463=CARTESIAN_POINT ( 'NONE',  ( 40.34137639590981195, 29.05937500034139376, -29.30972558990011834 ) ) ;
#2465=CARTESIAN_POINT ( 'NONE',  ( -30.81806926056963292, 47.62187500034139731, -42.41743335407646498 ) ) ;
#2470=FACE_OUTER_BOUND ( 'NONE', #5821, .T. ) ;
#2483=FACE_OUTER_BOUND ( 'NONE', #12356, .T. ) ;
#2484=CARTESIAN_POINT ( 'NONE',  ( -30.81806926056963292, 49.55937500034139731, -42.41743335407647209 ) ) ;
#2487=CARTESIAN_POINT ( 'NONE',  ( 7.919222016226809657, 25.22999571913595318, -50.00000000000000000 ) ) ;
#2491=CARTESIAN_POINT ( 'NONE',  ( -15.45084971874736368, 48.18125000068280173, 47.55282581475768211 ) ) ;
#2494=CARTESIAN_POINT ( 'NONE',  ( -30.81806926056963292, 21.55937500034140086, -42.41743335407647209 ) ) ;
#2495=CARTESIAN_POINT ( 'NONE',  ( -3.111920190527341144E-15, 29.50000000000000000, -50.00000000000000000 ) ) ;
#2498=EDGE_LOOP ( 'NONE', ( #5485, #3317, #14275, #955, #738, #6323, #1719 ) ) ;
#2501=CARTESIAN_POINT ( 'NONE',  ( 15.45084971874736723, 33.39999999999999858, -47.55282581475768211 ) ) ;
#2502=CARTESIAN_POINT ( 'NONE',  ( -14.89227969048185152, 31.70859663795358330, 93.22745684670599076 ) ) ;
#2507=CARTESIAN_POINT ( 'NONE',  ( -40.34137639590981195, 22.12187500034139731, 29.30972558990012189 ) ) ;
#2508=CARTESIAN_POINT ( 'NONE',  ( -15.40903463028480580, 20.25937500034139660, 47.42413220539094709 ) ) ;
#2510=CARTESIAN_POINT ( 'NONE',  ( -15.40903463028480580, 38.32187500034140015, 47.42413220539094709 ) ) ;
#2511=DIRECTION ( 'NONE',  ( 0.000000000000000000, 0.000000000000000000, 1.000000000000000000 ) ) ;
#2512=CARTESIAN_POINT ( 'NONE',  ( -50.00000000000000000, 34.00000000000000000, 0.000000000000000000 ) ) ;
#2513=CARTESIAN_POINT ( 'NONE',  ( 15.40903463028481113, 37.25937500034140015, -47.42413220539094709 ) ) ;
#2515=CARTESIAN_POINT ( 'NONE',  ( -30.90169943749473802, 42.30000000000000426, 42.53254041760200721 ) ) ;
#2527=( BOUNDED_CURVE ( )  B_SPLINE_CURVE ( 2, ( #11646, #1578, #638, #3486, #12211, #8301, #7151, #10809, #10961, #13837, #3227, #10719, #13535 ),
 .UNSPECIFIED., .F., .T. ) 
 B_SPLINE_CURVE_WITH_KNOTS ( ( 3, 2, 2, 2, 2, 2, 3 ),
 ( 0.1166666666666666685, 0.1199999999999999956, 0.1266666666666666774, 0.1333333333333333315, 0.1400000000000000133, 0.1466666666666666674, 0.1499999999999999944 ),
 .UNSPECIFIED. ) 
 CURVE ( )  GEOMETRIC_REPRESENTATION_ITEM ( )  RATIONAL_B_SPLINE_CURVE ( ( 0.9755282581475768211, 0.9755282581475768211, 1.000000000000000000, 0.9510565162951535312, 1.000000000000000000, 0.9510565162951535312, 1.000000000000000000, 0.9510565162951535312, 1.000000000000000000, 0.9510565162951535312, 1.000000000000000000, 0.9755282581475768211, 0.9755282581475768211 ) ) 
 REPRESENTATION_ITEM ( '' )  );
#2531=CARTESIAN_POINT ( 'NONE',  ( 30.81806926056962936, 41.22187500034139873, -42.41743335407647209 ) ) ;
#2534=CARTESIAN_POINT ( 'NONE',  ( -15.45084971874736368, 28.18125000068279817, 47.55282581475768211 ) ) ;
#2537=CARTESIAN_POINT ( 'NONE',  ( 15.40903463028481113, 35.32187500034139305, -47.42413220539094709 ) ) ;
#2538=CARTESIAN_POINT ( 'NONE',  ( -2.445080149700054274E-14, 46.50000000000000711, 50.00000000000000000 ) ) ;
#2550=CARTESIAN_POINT ( 'NONE',  ( 49.86468353125001585, 28.75937500034139305, 16.20201782572375038 ) ) ;
#2551=CARTESIAN_POINT ( 'NONE',  ( -49.86468353125000164, 45.92187500034139447, 0.000000000000000000 ) ) ;
#2554=AXIS2_PLACEMENT_3D ( 'NONE', #15387, #4009, #9079 ) ;
#2567=AXIS2_PLACEMENT_3D ( 'NONE', #8509, #15911, #13493 ) ;
#2576=CARTESIAN_POINT ( 'NONE',  ( 40.45084971874737079, 24.98125000068279888, -29.38926261462366440 ) ) ;
#2578=CARTESIAN_POINT ( 'NONE',  ( -50.00000000000000000, 50.00000000000000000, 0.000000000000000000 ) ) ;
#2579=CARTESIAN_POINT ( 'NONE',  ( 40.45084971874737789, 40.58125000068280031, 29.38926261462365375 ) ) ;
#2588=ORIENTED_EDGE ( 'NONE', *, *, #8894, .T. ) ;
#2597=CARTESIAN_POINT ( 'NONE',  ( 15.40903463028481113, 25.25937500034139660, -47.42413220539094709 ) ) ;
#2599=CARTESIAN_POINT ( 'NONE',  ( 40.34137639590981195, 37.12187500034139731, -29.30972558990011834 ) ) ;
#2601=CARTESIAN_POINT ( 'NONE',  ( -40.45084971874737079, 30.20000000000000284, 29.38926261462367151 ) ) ;
#2603=CARTESIAN_POINT ( 'NONE',  ( 40.34137639590981195, 39.05937500034140442, -29.30972558990011834 ) ) ;
#2605=CARTESIAN_POINT ( 'NONE',  ( -3.219174618344376363E-15, 43.50000000000000000, -52.57311121191334990 ) ) ;
#2618=CARTESIAN_POINT ( 'NONE',  ( -30.81806926056962226, 42.22187500034139163, 42.41743335407647919 ) ) ;
#2619=CARTESIAN_POINT ( 'NONE',  ( -15.40903463028480580, 40.25937500034139305, 47.42413220539094709 ) ) ;
#2622=CARTESIAN_POINT ( 'NONE',  ( -3.219174618344376363E-15, 27.28125000068279249, -52.57311121191334990 ) ) ;
#2623=CARTESIAN_POINT ( 'NONE',  ( -15.45084971874737256, 35.38125000068279746, -47.55282581475767500 ) ) ;
#2624=CARTESIAN_POINT ( 'NONE',  ( 40.34137639590981195, 31.12187500034139731, -29.30972558990011834 ) ) ;
#2625=CARTESIAN_POINT ( 'NONE',  ( -49.99999999999999289, 28.10000000000000497, 16.24598481164533226 ) ) ;
#2627=ORIENTED_EDGE ( 'NONE', *, *, #12849, .T. ) ;
#2631=CARTESIAN_POINT ( 'NONE',  ( -7.919222016226934890, 24.44874571845315714, 49.99999999999996447 ) ) ;
#2633=CARTESIAN_POINT ( 'NONE',  ( 30.81806926056964002, 34.55937500034139731, 42.41743335407647209 ) ) ;
#2634=CARTESIAN_POINT ( 'NONE',  ( 9.631387414534489405E-15, 44.42187500034140157, 52.43083105670540789 ) ) ;
#2637=CARTESIAN_POINT ( 'NONE',  ( 0.000000000000000000, 50.00000000000000000, -85.01963570546854498 ) ) ;
#2647=VECTOR ( 'NONE', #4240, 1000.000000000000000 ) ;
#2659=CARTESIAN_POINT ( 'NONE',  ( 30.90169943749474157, 41.08125000068280031, -42.53254041760200721 ) ) ;
#2667=CARTESIAN_POINT ( 'NONE',  ( 7.919222016226809657, 43.22999571913594963, -50.00000000000000000 ) ) ;
#2668=CARTESIAN_POINT ( 'NONE',  ( 0.000000000000000000, 20.00000000000000355, 0.000000000000000000 ) ) ;
#2669=( BOUNDED_CURVE ( )  B_SPLINE_CURVE ( 2, ( #4867, #12420, #4695, #8575, #13399, #3350, #1011, #7017, #12163, #8424, #7107, #9923, #2094 ),
 .UNSPECIFIED., .F., .F. ) 
 B_SPLINE_CURVE_WITH_KNOTS ( ( 3, 2, 2, 2, 2, 2, 3 ),
 ( 0.4833333333333333370, 0.4866666666666666918, 0.4933333333333333459, 0.5000000000000000000, 0.5066666666666667096, 0.5133333333333333082, 0.5166666666666667185 ),
 .UNSPECIFIED. ) 
 CURVE ( )  GEOMETRIC_REPRESENTATION_ITEM ( )  RATIONAL_B_SPLINE_CURVE ( ( 0.9755282581475768211, 0.9755282581475768211, 1.000000000000000000, 0.9510565162951535312, 1.000000000000000000, 0.9510565162951535312, 1.000000000000000000, 0.9510565162951535312, 1.000000000000000000, 0.9510565162951535312, 1.000000000000000000, 0.9755282581475763770, 0.9755282581475768211 ) ) 
 REPRESENTATION_ITEM ( '' )  );
#2672=CARTESIAN_POINT ( 'NONE',  ( 30.90169943749475223, 32.70000000000000284, 42.53254041760199300 ) ) ;
#2677=CARTESIAN_POINT ( 'NONE',  ( -30.81806926056963292, 23.55937500034139376, -42.41743335407646498 ) ) ;
#2678=FACE_OUTER_BOUND ( 'NONE', #15899, .T. ) ;
#2679=CARTESIAN_POINT ( 'NONE',  ( 9.631387414534489405E-15, 30.42187500034139447, 52.43083105670540789 ) ) ;
#2681=CARTESIAN_POINT ( 'NONE',  ( 49.99999999999999289, 31.09999999999999787, -16.24598481164532160 ) ) ;
#2682=CARTESIAN_POINT ( 'NONE',  ( -40.34137639590981905, 31.65937500034139873, -29.30972558990011478 ) ) ;
#2684=CARTESIAN_POINT ( 'NONE',  ( 30.90169943749474157, 41.30000000000001137, -42.53254041760200721 ) ) ;
#2694=CARTESIAN_POINT ( 'NONE',  ( -49.86468353125000164, 39.92187500034139447, 0.000000000000000000 ) ) ;
#2695=CARTESIAN_POINT ( 'NONE',  ( -30.81806926056963292, 45.55937500034139731, -42.41743335407646498 ) ) ;
#2696=CARTESIAN_POINT ( 'NONE',  ( -5.823736356558307894E-14, 44.50000000000000000, 50.00000000000000000 ) ) ;
#2699=CARTESIAN_POINT ( 'NONE',  ( -3.219174618344376363E-15, 25.28125000068279604, -52.57311121191334990 ) ) ;
#2700=CARTESIAN_POINT ( 'NONE',  ( 8.787474317778430688, 37.67774414662245164, 92.94678285709053966 ) ) ;
#2701=CARTESIAN_POINT ( 'NONE',  ( 30.81806926056962936, 29.22187500034139873, -42.41743335407647209 ) ) ;
#2702=CARTESIAN_POINT ( 'NONE',  ( -3.111920190527341144E-15, 27.50000000000000000, -50.00000000000000000 ) ) ;
#2703=VERTEX_POINT ( 'NONE', #12553 ) ;
#2705=ORIENTED_EDGE ( 'NONE', *, *, #4334, .F. ) ;
#2710=CARTESIAN_POINT ( 'NONE',  ( -49.86468353124999453, 31.95937500034139944, 16.20201782572377525 ) ) ;
#2712=CARTESIAN_POINT ( 'NONE',  ( 40.34137639590981905, 44.72187500034139163, 29.30972558990010768 ) ) ;
#2717=ORIENTED_EDGE ( 'NONE', *, *, #13322, .F. ) ;
#2720=ORIENTED_EDGE ( 'NONE', *, *, #4595, .F. ) ;
#2721=CARTESIAN_POINT ( 'NONE',  ( 6.123233995736766085E-15, 20.00000000000000355, -50.00000000000000000 ) ) ;
#2722=ORIENTED_EDGE ( 'NONE', *, *, #1549, .T. ) ;
#2728=CARTESIAN_POINT ( 'NONE',  ( 50.00000000000000711, 26.89999999999999503, 16.24598481164530739 ) ) ;
#2731=CARTESIAN_POINT ( 'NONE',  ( -49.99999999999999289, 25.68125000068279817, -16.24598481164531449 ) ) ;
#2732=CARTESIAN_POINT ( 'NONE',  ( 50.00000000000000711, 24.68125000068279462, 16.24598481164530739 ) ) ;
#2735=CARTESIAN_POINT ( 'NONE',  ( 15.45084971874736723, 41.18125000068280173, -47.55282581475768211 ) ) ;
#2739=EDGE_CURVE ( 'NONE', #40, #9078, #689, .T. ) ;
#2741=VERTEX_POINT ( 'NONE', #556 ) ;
#2744=AXIS2_PLACEMENT_3D ( 'NONE', #14436, #2907, #2821 ) ;
#2749=EDGE_LOOP ( 'NONE', ( #3498, #3015, #13277, #12584 ) ) ;
#2755=CARTESIAN_POINT ( 'NONE',  ( -40.45084971874737079, 29.98125000068279888, 29.38926261462367151 ) ) ;
#2756=CARTESIAN_POINT ( 'NONE',  ( -40.34137639590981195, 24.05937500034139731, 29.30972558990012189 ) ) ;
#2757=CARTESIAN_POINT ( 'NONE',  ( -1.224646799147353217E-14, 0.000000000000000000, -100.0000000000000000 ) ) ;
#2758=CARTESIAN_POINT ( 'NONE',  ( -49.86468353124999453, 32.02187500034139589, 16.20201782572377169 ) ) ;
#2761=CARTESIAN_POINT ( 'NONE',  ( -49.99999999999999289, 34.10000000000000853, 16.24598481164533226 ) ) ;
#2762=CARTESIAN_POINT ( 'NONE',  ( 30.81806926056962936, 31.15937500034139518, -42.41743335407647209 ) ) ;
#2764=ORIENTED_EDGE ( 'NONE', *, *, #3779, .F. ) ;
#2766=EDGE_CURVE ( 'NONE', #16188, #14047, #10606, .T. ) ;
#2772=CIRCLE ( 'NONE', #12062, 50.00000000000000000 ) ;
#2777=CARTESIAN_POINT ( 'NONE',  ( -49.86468353124999453, 37.82187500034139305, -16.20201782572375393 ) ) ;
#2778=CARTESIAN_POINT ( 'NONE',  ( 49.86468353125001585, 44.75937500034139305, 16.20201782572375038 ) ) ;
#2781=CARTESIAN_POINT ( 'NONE',  ( -49.86468353125000164, 49.85937500034139447, 0.000000000000000000 ) ) ;
#2783=MECHANICAL_DESIGN_GEOMETRIC_PRESENTATION_REPRESENTATION('',(#4121),#12873);
#2784=CARTESIAN_POINT ( 'NONE',  ( -49.86468353125000164, 29.92187500034139802, 0.000000000000000000 ) ) ;
#2795=CARTESIAN_POINT ( 'NONE',  ( 49.86468353125001585, 22.75937500034139660, 16.20201782572375038 ) ) ;
#2798=CARTESIAN_POINT ( 'NONE',  ( -30.81806926056963292, 43.62187500034139020, -42.41743335407646498 ) ) ;
#2800=CARTESIAN_POINT ( 'NONE',  ( -15.40903463028480580, 46.32187500034140015, 47.42413220539094709 ) ) ;
#2804=VECTOR ( 'NONE', #1089, 1000.000000000000000 ) ;
#2814=DIRECTION ( 'NONE',  ( -0.000000000000000000, -1.000000000000000000, -0.000000000000000000 ) ) ;
#2816=CARTESIAN_POINT ( 'NONE',  ( -40.45084971874737789, 27.80000000000000071, -29.38926261462365730 ) ) ;
#2818=CARTESIAN_POINT ( 'NONE',  ( 30.81806926056962936, 47.15937500034138452, -42.41743335407647209 ) ) ;
#2821=DIRECTION ( 'NONE',  ( 0.000000000000000000, 0.000000000000000000, 1.000000000000000000 ) ) ;
#2824=CARTESIAN_POINT ( 'NONE',  ( -15.40903463028481646, 21.52187500034139589, -47.42413220539093999 ) ) ;
#2827=CARTESIAN_POINT ( 'NONE',  ( -15.45084971874737256, 37.38125000068279746, -47.55282581475767500 ) ) ;
#2841=CARTESIAN_POINT ( 'NONE',  ( -11.57407943811421802, 35.63861574361248330, 92.99953801807581044 ) ) ;
#2845=CARTESIAN_POINT ( 'NONE',  ( -15.45084971874737256, 29.38125000068279746, -47.55282581475767500 ) ) ;
#2847=CARTESIAN_POINT ( 'NONE',  ( 2.894151059106554236, 5.231075460314085213, 99.03700517889676291 ) ) ;
#2848=CARTESIAN_POINT ( 'NONE',  ( -46.79661121261588619, 20.00000000000000355, 17.22183559214931492 ) ) ;
#2849=CARTESIAN_POINT ( 'NONE',  ( -49.86468353124999453, 28.02187500034139589, 16.20201782572377169 ) ) ;
#2852=CARTESIAN_POINT ( 'NONE',  ( -49.99999999999999289, 31.89999999999999858, -16.24598481164531449 ) ) ;
#2853=CARTESIAN_POINT ( 'NONE',  ( 49.86468353125001585, 32.75937500034140015, 16.20201782572375038 ) ) ;
#2859=ORIENTED_EDGE ( 'NONE', *, *, #8927, .T. ) ;
#2863=CYLINDRICAL_SURFACE ( 'NONE', #14977, 50.00000000000000000 ) ;
#2867=CARTESIAN_POINT ( 'NONE',  ( -30.81806926056963292, 33.62187500034139731, -42.41743335407647209 ) ) ;
#2868=CARTESIAN_POINT ( 'NONE',  ( 49.86468353125000164, 32.85937500034139447, -6.106662507704105588E-15 ) ) ;
#2872=CARTESIAN_POINT ( 'NONE',  ( 30.90169943749474157, 23.08125000068279320, -42.53254041760200721 ) ) ;
#2874=( BOUNDED_CURVE ( )  B_SPLINE_CURVE ( 2, ( #4425, #5597, #1904, #13304, #498, #4342, #8070, #334, #8161, #9407, #10494, #3084, #4183 ),
 .UNSPECIFIED., .F., .F. ) 
 B_SPLINE_CURVE_WITH_KNOTS ( ( 3, 2, 2, 2, 2, 2, 3 ),
 ( 0.8833333333333334147, 0.8866666666666667140, 0.8933333333333333126, 0.9000000000000000222, 0.9066666666666666208, 0.9133333333333333304, 0.9166666666666667407 ),
 .UNSPECIFIED. ) 
 CURVE ( )  GEOMETRIC_REPRESENTATION_ITEM ( )  RATIONAL_B_SPLINE_CURVE ( ( 0.9755282581475768211, 0.9755282581475771542, 1.000000000000000000, 0.9510565162951535312, 1.000000000000000000, 0.9510565162951535312, 1.000000000000000000, 0.9510565162951535312, 1.000000000000000000, 0.9510565162951535312, 1.000000000000000000, 0.9755282581475763770, 0.9755282581475768211 ) ) 
 REPRESENTATION_ITEM ( '' )  );
#2875=CARTESIAN_POINT ( 'NONE',  ( 9.631387414534489405E-15, 28.42187500034139092, 52.43083105670540789 ) ) ;
#2883=CARTESIAN_POINT ( 'NONE',  ( 7.919222016226693306, 30.33250428222964246, 50.00000000000003553 ) ) ;
#2885=CARTESIAN_POINT ( 'NONE',  ( -49.86468353125000164, 21.85937500034139802, 0.000000000000000000 ) ) ;
#2887=DIRECTION ( 'NONE',  ( 0.000000000000000000, 0.000000000000000000, 1.000000000000000000 ) ) ;
#2888=CARTESIAN_POINT ( 'NONE',  ( 49.86468353124999453, 43.02187500034138878, -16.20201782572376104 ) ) ;
#2890=DIRECTION ( 'NONE',  ( -0.000000000000000000, 1.000000000000000000, -0.000000000000000000 ) ) ;
#2893=CARTESIAN_POINT ( 'NONE',  ( -49.86468353124999453, 48.02187500034139589, 16.20201782572377525 ) ) ;
#2895=ORIENTED_EDGE ( 'NONE', *, *, #7557, .F. ) ;
#2901=CARTESIAN_POINT ( 'NONE',  ( -40.45084971874737079, 43.98125000068279888, 29.38926261462367151 ) ) ;
#2903=DIRECTION ( 'NONE',  ( -0.000000000000000000, 1.000000000000000000, -0.000000000000000000 ) ) ;
#2904=CARTESIAN_POINT ( 'NONE',  ( 50.00000000000000000, 27.00000000000000355, -6.123233995736766085E-15 ) ) ;
#2906=CARTESIAN_POINT ( 'NONE',  ( -49.86468353124999453, 41.75937500034139305, -16.20201782572375393 ) ) ;
#2907=DIRECTION ( 'NONE',  ( -0.000000000000000000, 1.000000000000000000, -0.000000000000000000 ) ) ;
#2910=CARTESIAN_POINT ( 'NONE',  ( 30.90169943749475578, 40.48125000068279888, 42.53254041760200010 ) ) ;
#2913=CARTESIAN_POINT ( 'NONE',  ( 7.919222016226693306, 22.33250428222964601, 50.00000000000003553 ) ) ;
#2914=EDGE_CURVE ( 'NONE', #4422, #5607, #13285, .T. ) ;
#2923=ORIENTED_EDGE ( 'NONE', *, *, #13600, .T. ) ;
#2924=CARTESIAN_POINT ( 'NONE',  ( 1.235979693235591175E-19, 4.999999999999997335, 99.11836509645767990 ) ) ;
#2930=CARTESIAN_POINT ( 'NONE',  ( -46.38089879718444308, 20.00000000000000355, 18.31192695794416636 ) ) ;
#2931=CARTESIAN_POINT ( 'NONE',  ( 15.40903463028481113, 29.32187500034139660, -47.42413220539094709 ) ) ;
#2934=CARTESIAN_POINT ( 'NONE',  ( -40.34137639590981195, 32.05937500034139731, 29.30972558990012189 ) ) ;
#2939=ORIENTED_EDGE ( 'NONE', *, *, #5033, .F. ) ;
#2945=CARTESIAN_POINT ( 'NONE',  ( 15.40903463028482356, 36.52187500034139589, 47.42413220539093999 ) ) ;
#2946=CARTESIAN_POINT ( 'NONE',  ( -15.40903463028481646, 37.45937500034139589, -47.42413220539093999 ) ) ;
#2949=CARTESIAN_POINT ( 'NONE',  ( 15.40903463028482356, 48.45937500034140299, 47.42413220539093999 ) ) ;
#2951=CARTESIAN_POINT ( 'NONE',  ( -40.34137639590981905, 27.72187500034139873, -29.30972558990011478 ) ) ;
#2962=CARTESIAN_POINT ( 'NONE',  ( 40.34137639590981905, 26.65937500034139518, 29.30972558990010768 ) ) ;
#2964=( BOUNDED_CURVE ( )  B_SPLINE_CURVE ( 2, ( #7331, #13384, #1907, #11072, #658, #3247, #9746, #8319, #8404, #13473, #2080, #10982, #16045 ),
 .UNSPECIFIED., .F., .T. ) 
 B_SPLINE_CURVE_WITH_KNOTS ( ( 3, 2, 2, 2, 2, 2, 3 ),
 ( 0.5833333333333333703, 0.5866666666666666696, 0.5933333333333333792, 0.5999999999999999778, 0.6066666666666666874, 0.6133333333333332860, 0.6166666666666666963 ),
 .UNSPECIFIED. ) 
 CURVE ( )  GEOMETRIC_REPRESENTATION_ITEM ( )  RATIONAL_B_SPLINE_CURVE ( ( 0.9755282581475768211, 0.9755282581475771542, 1.000000000000000000, 0.9510565162951535312, 1.000000000000000000, 0.9510565162951535312, 1.000000000000000000, 0.9510565162951535312, 1.000000000000000000, 0.9510565162951535312, 1.000000000000000000, 0.9755282581475763770, 0.9755282581475768211 ) ) 
 REPRESENTATION_ITEM ( '' )  );
#2966=CARTESIAN_POINT ( 'NONE',  ( 15.40903463028481113, 41.32187500034140015, -47.42413220539094709 ) ) ;
#2968=CARTESIAN_POINT ( 'NONE',  ( 40.34137639590981905, 46.72187500034139873, 29.30972558990010768 ) ) ;
#2975=CARTESIAN_POINT ( 'NONE',  ( 0.000000000000000000, 28.00000000000000355, -10.00000000000000000 ) ) ;
#2978=CARTESIAN_POINT ( 'NONE',  ( 40.45084971874737079, 25.19999999999999929, -29.38926261462366440 ) ) ;
#2979=CARTESIAN_POINT ( 'NONE',  ( -15.40903463028480580, 46.25937500034140015, 47.42413220539094709 ) ) ;
#2980=CYLINDRICAL_SURFACE ( 'NONE', #2744, 50.00000000000000000 ) ;
#2986=CARTESIAN_POINT ( 'NONE',  ( 40.45084971874737789, 34.58125000068280031, 29.38926261462365375 ) ) ;
#2991=ORIENTED_EDGE ( 'NONE', *, *, #294, .T. ) ;
#2994=EDGE_LOOP ( 'NONE', ( #15651, #3835, #7901, #608 ) ) ;
#2995=FACE_OUTER_BOUND ( 'NONE', #3645, .T. ) ;
#2996=DIRECTION ( 'NONE',  ( -0.000000000000000000, 1.000000000000000000, -0.000000000000000000 ) ) ;
#3006=CARTESIAN_POINT ( 'NONE',  ( -48.07045810499274552, 20.00000000000000355, 13.25585611146461140 ) ) ;
#3007=CARTESIAN_POINT ( 'NONE',  ( 49.86468353125000164, 26.92187500034139802, -6.106662507704105588E-15 ) ) ;
#3010=CARTESIAN_POINT ( 'NONE',  ( -15.40903463028481646, 35.45937500034139589, -47.42413220539093999 ) ) ;
#3015=ORIENTED_EDGE ( 'NONE', *, *, #10406, .T. ) ;
#3022=CARTESIAN_POINT ( 'NONE',  ( 49.86468353124999453, 37.02187500034138878, -16.20201782572376459 ) ) ;
#3023=CARTESIAN_POINT ( 'NONE',  ( 30.81806926056962936, 39.15937500034139873, -42.41743335407646498 ) ) ;
#3026=CARTESIAN_POINT ( 'NONE',  ( -3.219174618344376363E-15, 23.28125000068279959, -52.57311121191334990 ) ) ;
#3029=CARTESIAN_POINT ( 'NONE',  ( 49.86468353125001585, 24.82187500034139305, 16.20201782572375038 ) ) ;
#3038=CARTESIAN_POINT ( 'NONE',  ( 49.86468353124999453, 24.95937500034139234, -16.20201782572376459 ) ) ;
#3042=CIRCLE ( 'NONE', #12338, 10.00000000000000000 ) ;
#3043=CARTESIAN_POINT ( 'NONE',  ( -40.34137639590981905, 41.72187500034139873, -29.30972558990011478 ) ) ;
#3044=CARTESIAN_POINT ( 'NONE',  ( -15.40903463028480580, 44.32187500034140015, 47.42413220539094709 ) ) ;
#3045=CARTESIAN_POINT ( 'NONE',  ( 15.45084971874736723, 31.39999999999999858, -47.55282581475768211 ) ) ;
#3046=ORIENTED_EDGE ( 'NONE', *, *, #15738, .F. ) ;
#3054=CARTESIAN_POINT ( 'NONE',  ( 0.000000000000000000, 45.07596123493892293, 0.000000000000000000 ) ) ;
#3057=CARTESIAN_POINT ( 'NONE',  ( 30.90169943749475578, 22.69999999999999929, 42.53254041760200010 ) ) ;
#3058=CARTESIAN_POINT ( 'NONE',  ( 15.40903463028481113, 41.25937500034139305, -47.42413220539094709 ) ) ;
#3064=CARTESIAN_POINT ( 'NONE',  ( -3.219174618344376363E-15, 33.28125000068280315, -52.57311121191334990 ) ) ;
#3070=ORIENTED_EDGE ( 'NONE', *, *, #3752, .T. ) ;
#3072=EDGE_LOOP ( 'NONE', ( #5934, #6574, #10932, #11783 ) ) ;
#3084=CARTESIAN_POINT ( 'NONE',  ( 7.919222016226693306, 22.55125428154684286, 50.00000000000003553 ) ) ;
#3087=CARTESIAN_POINT ( 'NONE',  ( -30.90169943749473447, 38.08125000068280031, 42.53254041760200721 ) ) ;
#3088=CARTESIAN_POINT ( 'NONE',  ( 14.90054083259177453, 13.30529623682518370, 96.51097829310403142 ) ) ;
#3089=CARTESIAN_POINT ( 'NONE',  ( -47.07787634996812187, 19.99999999999999645, 16.43739640347152786 ) ) ;
#3090=EDGE_CURVE ( 'NONE', #6101, #7762, #6471, .T. ) ;
#3091=CARTESIAN_POINT ( 'NONE',  ( -3.210462471511496205E-15, 25.42187500034139447, -52.43083105670540789 ) ) ;
#3092=CARTESIAN_POINT ( 'NONE',  ( -7.919222016226934890, 22.44874571845315714, 49.99999999999996447 ) ) ;
#3096=CARTESIAN_POINT ( 'NONE',  ( 30.81806926056964002, 24.55937500034139376, 42.41743335407647209 ) ) ;
#3111=CARTESIAN_POINT ( 'NONE',  ( -30.81806926056963292, 29.62187500034139376, -42.41743335407647209 ) ) ;
#3112=CARTESIAN_POINT ( 'NONE',  ( -40.34137639590981905, 35.65937500034139873, -29.30972558990011478 ) ) ;
#3113=CARTESIAN_POINT ( 'NONE',  ( -7.919222016226816763, 43.55125428154684641, -49.99999999999999289 ) ) ;
#3116=CARTESIAN_POINT ( 'NONE',  ( 30.90169943749474157, 21.08125000068279675, -42.53254041760200721 ) ) ;
#3119=CARTESIAN_POINT ( 'NONE',  ( -49.86468353125000164, 21.92187500034139802, 0.000000000000000000 ) ) ;
#3129=CARTESIAN_POINT ( 'NONE',  ( 40.34137639590981195, 23.05937500034139731, -29.30972558990011834 ) ) ;
#3132=CARTESIAN_POINT ( 'NONE',  ( 9.657523855033129090E-15, 38.50000000000000711, 52.57311121191334990 ) ) ;
#3133=CARTESIAN_POINT ( 'NONE',  ( 40.34137639590981195, 49.12187500034139731, -29.30972558990011834 ) ) ;
#3139=LINE ( 'NONE', #2975, #15053 ) ;
#3143=CARTESIAN_POINT ( 'NONE',  ( -30.81806926056962226, 46.15937500034139873, 42.41743335407647919 ) ) ;
#3144=CARTESIAN_POINT ( 'NONE',  ( 6.123233995736766085E-15, 20.00000000000000355, -50.00000000000000000 ) ) ;
#3158=( BOUNDED_CURVE ( )  B_SPLINE_CURVE ( 2, ( #9624, #14928, #8703, #1124, #880, #6219, #8461 ),
 .UNSPECIFIED., .F., .F. ) 
 B_SPLINE_CURVE_WITH_KNOTS ( ( 3, 2, 2, 3 ),
 ( 0.000000000000000000, 0.006666666666666667095, 0.01333333333333333419, 0.01666666666666666990 ),
 .UNSPECIFIED. ) 
 CURVE ( )  GEOMETRIC_REPRESENTATION_ITEM ( )  RATIONAL_B_SPLINE_CURVE ( ( 1.000000000000000000, 0.9510565162951535312, 1.000000000000000000, 0.9510565162951535312, 1.000000000000000000, 0.9755282581475768211, 0.9755282581475768211 ) ) 
 REPRESENTATION_ITEM ( '' )  );
#3160=ADVANCED_FACE ( 'NONE', ( #126 ), #12994, .T. ) ;
#3164=FACE_OUTER_BOUND ( 'NONE', #14409, .T. ) ;
#3167=EDGE_CURVE ( 'NONE', #842, #13696, #15350, .T. ) ;
#3170=DIRECTION ( 'NONE',  ( -0.000000000000000000, 1.000000000000000000, -0.000000000000000000 ) ) ;
#3173=CARTESIAN_POINT ( 'NONE',  ( 17.50000000000000355, 21.92738356273111222, 94.52735820379716358 ) ) ;
#3174=CARTESIAN_POINT ( 'NONE',  ( -47.44954343046507717, 20.00000000000001066, 15.33151233206156228 ) ) ;
#3175=CARTESIAN_POINT ( 'NONE',  ( 49.86468353125001585, 22.82187500034139305, 16.20201782572375038 ) ) ;
#3178=CARTESIAN_POINT ( 'NONE',  ( 40.34137639590981195, 25.05937500034139376, -29.30972558990011834 ) ) ;
#3180=ORIENTED_EDGE ( 'NONE', *, *, #12207, .T. ) ;
#3182=VERTEX_POINT ( 'NONE', #7393 ) ;
#3188=CARTESIAN_POINT ( 'NONE',  ( 30.81806926056962936, 27.22187500034139518, -42.41743335407647209 ) ) ;
#3189=CARTESIAN_POINT ( 'NONE',  ( 15.40903463028482356, 36.45937500034139589, 47.42413220539093999 ) ) ;
#3193=CARTESIAN_POINT ( 'NONE',  ( 15.40903463028482356, 42.45937500034140299, 47.42413220539093999 ) ) ;
#3195=CARTESIAN_POINT ( 'NONE',  ( -40.45084971874737789, 49.80000000000000426, -29.38926261462365730 ) ) ;
#3198=ORIENTED_EDGE ( 'NONE', *, *, #6749, .T. ) ;
#3202=( BOUNDED_CURVE ( )  B_SPLINE_CURVE ( 2, ( #12058, #7915, #1673, #9411, #8166, #13235, #1833, #6927, #16218, #10983, #2240, #10904, #10827 ),
 .UNSPECIFIED., .F., .F. ) 
 B_SPLINE_CURVE_WITH_KNOTS ( ( 3, 2, 2, 2, 2, 2, 3 ),
 ( 0.08333333333333334259, 0.08666666666666666963, 0.09333333333333333759, 0.1000000000000000056, 0.1066666666666666735, 0.1133333333333333276, 0.1166666666666666685 ),
 .UNSPECIFIED. ) 
 CURVE ( )  GEOMETRIC_REPRESENTATION_ITEM ( )  RATIONAL_B_SPLINE_CURVE ( ( 0.9755282581475768211, 0.9755282581475768211, 1.000000000000000000, 0.9510565162951535312, 1.000000000000000000, 0.9510565162951535312, 1.000000000000000000, 0.9510565162951535312, 1.000000000000000000, 0.9510565162951535312, 1.000000000000000000, 0.9755282581475767101, 0.9755282581475768211 ) ) 
 REPRESENTATION_ITEM ( '' )  );
#3206=CARTESIAN_POINT ( 'NONE',  ( 49.86468353125000164, 46.92187500034139447, -6.106662507704105588E-15 ) ) ;
#3209=CARTESIAN_POINT ( 'NONE',  ( -15.45084971874737256, 35.60000000000000142, -47.55282581475767500 ) ) ;
#3211=CARTESIAN_POINT ( 'NONE',  ( 40.34137639590981905, 38.72187500034139873, 29.30972558990010768 ) ) ;
#3213=ORIENTED_EDGE ( 'NONE', *, *, #8420, .T. ) ;
#3219=CARTESIAN_POINT ( 'NONE',  ( 8.660254037844387298, 20.00000000000000355, 5.000000000000000000 ) ) ;
#3220=LINE ( 'NONE', #13119, #519 ) ;
#3221=CARTESIAN_POINT ( 'NONE',  ( 15.45084971874737789, 36.38125000068279746, 47.55282581475767500 ) ) ;
#3222=CARTESIAN_POINT ( 'NONE',  ( -49.86468353124999453, 37.75937500034140015, -16.20201782572375393 ) ) ;
#3223=CARTESIAN_POINT ( 'NONE',  ( 9.631387414534489405E-15, 46.35937500034139447, 52.43083105670540789 ) ) ;
#3225=CARTESIAN_POINT ( 'NONE',  ( -49.86468353125000164, 19.92187500034139447, 0.000000000000000000 ) ) ;
#3227=CARTESIAN_POINT ( 'NONE',  ( -15.45084971874737256, 45.60000000000000142, -47.55282581475767500 ) ) ;
#3231=ADVANCED_BREP_SHAPE_REPRESENTATION ( '', ( #8848, #15812 ), #1480 ) ;
#3247=CARTESIAN_POINT ( 'NONE',  ( -49.99999999999999289, 32.10000000000000142, 16.24598481164533226 ) ) ;
#3252=CARTESIAN_POINT ( 'NONE',  ( -46.00570371104000600, 20.06239642599078365, 21.51344788172391631 ) ) ;
#3255=CARTESIAN_POINT ( 'NONE',  ( -15.40903463028481646, 27.45937500034139944, -47.42413220539093999 ) ) ;
#3261=ORIENTED_EDGE ( 'NONE', *, *, #16032, .T. ) ;
#3262=DIRECTION ( 'NONE',  ( -0.000000000000000000, 1.000000000000000000, -0.000000000000000000 ) ) ;
#3269=CARTESIAN_POINT ( 'NONE',  ( 40.34137639590981905, 28.72187500034139873, 29.30972558990010768 ) ) ;
#3270=CARTESIAN_POINT ( 'NONE',  ( -49.86468353124999453, 31.75937500034140015, -16.20201782572375393 ) ) ;
#3271=CARTESIAN_POINT ( 'NONE',  ( 8.446640517145639571E-15, 26.28125000068279959, 50.00000000000000000 ) ) ;
#3275=CARTESIAN_POINT ( 'NONE',  ( -49.86468353124999453, 41.95937500034138878, 16.20201782572377525 ) ) ;
#3278=CARTESIAN_POINT ( 'NONE',  ( 9.631387414534489405E-15, 24.42187500034139447, 52.43083105670540789 ) ) ;
#3279=ORIENTED_EDGE ( 'NONE', *, *, #4297, .T. ) ;
#3285=CARTESIAN_POINT ( 'NONE',  ( 0.000000000000000000, 20.00000000000000355, 0.000000000000000000 ) ) ;
#3287=CARTESIAN_POINT ( 'NONE',  ( 30.81806926056964002, 48.62187500034139731, 42.41743335407647209 ) ) ;
#3290=CARTESIAN_POINT ( 'NONE',  ( -30.90169943749474868, 39.70000000000000284, -42.53254041760200721 ) ) ;
#3293=CARTESIAN_POINT ( 'NONE',  ( 49.86468353125000164, 40.92187500034139447, -6.106662507704105588E-15 ) ) ;
#3304=CARTESIAN_POINT ( 'NONE',  ( 49.99999999999999289, 27.10000000000000142, -16.24598481164532160 ) ) ;
#3306=CARTESIAN_POINT ( 'NONE',  ( 40.34137639590981195, 35.05937500034139731, -29.30972558990011834 ) ) ;
#3310=CARTESIAN_POINT ( 'NONE',  ( -2.547328955960238000E-13, 34.28125000068279604, 49.99999999999999289 ) ) ;
#3311=CARTESIAN_POINT ( 'NONE',  ( 0.000000000000000000, 50.00000000000000000, 0.000000000000000000 ) ) ;
#3314=ORIENTED_EDGE ( 'NONE', *, *, #9141, .F. ) ;
#3317=ORIENTED_EDGE ( 'NONE', *, *, #6451, .T. ) ;
#3318=VERTEX_POINT ( 'NONE', #11155 ) ;
#3319=ORIENTED_EDGE ( 'NONE', *, *, #8755, .T. ) ;
#3332=CARTESIAN_POINT ( 'NONE',  ( -30.90169943749473447, 48.30000000000000426, 42.53254041760200721 ) ) ;
#3335=CARTESIAN_POINT ( 'NONE',  ( -45.80914010100533318, 19.99999999999998934, 19.69865795820142296 ) ) ;
#3336=CARTESIAN_POINT ( 'NONE',  ( 40.34137639590981905, 24.72187500034139873, 29.30972558990010768 ) ) ;
#3339=CARTESIAN_POINT ( 'NONE',  ( 49.86468353125001585, 22.75937500034139660, 16.20201782572375038 ) ) ;
#3350=CARTESIAN_POINT ( 'NONE',  ( 49.99999999999999289, 35.10000000000000853, -16.24598481164532160 ) ) ;
#3353=CARTESIAN_POINT ( 'NONE',  ( 9.631387414534489405E-15, 30.42187500034139447, 52.43083105670540789 ) ) ;
#3354=CARTESIAN_POINT ( 'NONE',  ( 15.40903463028482356, 26.45937500034139589, 47.42413220539093999 ) ) ;
#3360=CARTESIAN_POINT ( 'NONE',  ( -15.40903463028481646, 43.45937500034139589, -47.42413220539093999 ) ) ;
#3364=CARTESIAN_POINT ( 'NONE',  ( -30.90169943749474868, 49.70000000000000284, -42.53254041760200721 ) ) ;
#3374=EDGE_CURVE ( 'NONE', #9264, #11588, #9646, .T. ) ;
#3375=CARTESIAN_POINT ( 'NONE',  ( 1.293669679204937499E-13, 41.28125000068279604, -50.00000000000000000 ) ) ;
#3377=CARTESIAN_POINT ( 'NONE',  ( 40.34137639590981905, 48.72187500034139873, 29.30972558990010768 ) ) ;
#3380=CARTESIAN_POINT ( 'NONE',  ( -3.219174618344376363E-15, 35.28125000068280315, -52.57311121191334990 ) ) ;
#3381=CARTESIAN_POINT ( 'NONE',  ( 30.90169943749474157, 39.30000000000000426, -42.53254041760200721 ) ) ;
#3383=CARTESIAN_POINT ( 'NONE',  ( -40.34137639590981905, 37.72187500034139873, -29.30972558990011478 ) ) ;
#3393=CARTESIAN_POINT ( 'NONE',  ( -7.919222016226870942, 40.22999571913594963, 49.99999999999997158 ) ) ;
#3395=CARTESIAN_POINT ( 'NONE',  ( 15.45084971874736723, 27.40000000000000213, -47.55282581475768211 ) ) ;
#3397=CARTESIAN_POINT ( 'NONE',  ( -49.86468353125000164, 37.85937500034139447, 0.000000000000000000 ) ) ;
#3398=CARTESIAN_POINT ( 'NONE',  ( -15.40903463028480580, 48.25937500034140015, 47.42413220539094709 ) ) ;
#3418=AXIS2_PLACEMENT_3D ( 'NONE', #15258, #16350, #16194 ) ;
#3419=CARTESIAN_POINT ( 'NONE',  ( -2.547328955960238000E-13, 20.49999999999999645, 49.99999999999999289 ) ) ;
#3425=ADVANCED_FACE ( 'NONE', ( #2483 ), #9980, .F. ) ;
#3428=CARTESIAN_POINT ( 'NONE',  ( 9.631387414534489405E-15, 20.42187500034139447, 52.43083105670540789 ) ) ;
#3431=CARTESIAN_POINT ( 'NONE',  ( -40.34137639590981195, 26.05937500034139731, 29.30972558990012189 ) ) ;
#3432=CARTESIAN_POINT ( 'NONE',  ( -15.45084971874736368, 42.18125000068279462, 47.55282581475768211 ) ) ;
#3433=CARTESIAN_POINT ( 'NONE',  ( -15.45084971874736368, 30.40000000000000213, 47.55282581475768211 ) ) ;
#3441=CARTESIAN_POINT ( 'NONE',  ( 0.000000000000000000, 20.00000000000000355, -10.00000000000000000 ) ) ;
#3443=CARTESIAN_POINT ( 'NONE',  ( -3.210462471511496205E-15, 29.42187500034139092, -52.43083105670540789 ) ) ;
#3444=CARTESIAN_POINT ( 'NONE',  ( -30.81806926056963292, 29.55937500034139376, -42.41743335407646498 ) ) ;
#3448=CARTESIAN_POINT ( 'NONE',  ( 15.40903463028481113, 45.25937500034140015, -47.42413220539094709 ) ) ;
#3450=CARTESIAN_POINT ( 'NONE',  ( -15.45084971874737256, 49.60000000000000853, -47.55282581475767500 ) ) ;
#3457=CARTESIAN_POINT ( 'NONE',  ( 50.00000000000000711, 40.68125000068280173, 16.24598481164530739 ) ) ;
#3459=CARTESIAN_POINT ( 'NONE',  ( -30.81806926056963292, 21.55937500034140086, -42.41743335407647209 ) ) ;
#3463=CARTESIAN_POINT ( 'NONE',  ( -40.45084971874737789, 31.58125000068280031, -29.38926261462365730 ) ) ;
#3466=CARTESIAN_POINT ( 'NONE',  ( 49.86468353125001585, 42.82187500034139305, 16.20201782572375038 ) ) ;
#3475=CARTESIAN_POINT ( 'NONE',  ( -40.45084971874737079, 39.98125000068279888, 29.38926261462367151 ) ) ;
#3479=CARTESIAN_POINT ( 'NONE',  ( 9.657523855033129090E-15, 20.50000000000000355, 52.57311121191334990 ) ) ;
#3480=CARTESIAN_POINT ( 'NONE',  ( -49.86468353125000164, 35.85937500034140157, 0.000000000000000000 ) ) ;
#3481=CARTESIAN_POINT ( 'NONE',  ( 15.40903463028482356, 48.45937500034140299, 47.42413220539093999 ) ) ;
#3486=CARTESIAN_POINT ( 'NONE',  ( -30.90169943749473447, 46.30000000000000426, 42.53254041760200721 ) ) ;
#3495=FACE_OUTER_BOUND ( 'NONE', #6655, .T. ) ;
#3498=ORIENTED_EDGE ( 'NONE', *, *, #10033, .F. ) ;
#3501=CARTESIAN_POINT ( 'NONE',  ( -17.36041212498391673, 20.22110460638136331, 94.85899783816353192 ) ) ;
#3508=CARTESIAN_POINT ( 'NONE',  ( -30.90169943749473802, 44.08125000068279320, 42.53254041760200721 ) ) ;
#3512=CARTESIAN_POINT ( 'NONE',  ( -49.86468353124999453, 21.75937500034140015, -16.20201782572375393 ) ) ;
#3514=CARTESIAN_POINT ( 'NONE',  ( -30.90169943749474513, 29.69999999999999929, -42.53254041760200721 ) ) ;
#3516=CARTESIAN_POINT ( 'NONE',  ( 7.919222016226791006, 44.55125428154683931, 50.00000000000000711 ) ) ;
#3520=CARTESIAN_POINT ( 'NONE',  ( -29.32979127811529096, 20.09142360399907190, 43.04328433925359576 ) ) ;
#3524=CARTESIAN_POINT ( 'NONE',  ( -49.86468353125000164, 23.92187500034139447, 0.000000000000000000 ) ) ;
#3525=CARTESIAN_POINT ( 'NONE',  ( 30.81806926056962936, 31.15937500034139163, -42.41743335407646498 ) ) ;
#3526=CARTESIAN_POINT ( 'NONE',  ( 50.00000000000000711, 26.68125000068279462, 16.24598481164530739 ) ) ;
#3527=CARTESIAN_POINT ( 'NONE',  ( -3.210462471511496205E-15, 37.42187500034140157, -52.43083105670540789 ) ) ;
#3529=CARTESIAN_POINT ( 'NONE',  ( -15.40903463028481646, 45.45937500034139589, -47.42413220539093999 ) ) ;
#3532=CARTESIAN_POINT ( 'NONE',  ( 49.99999999999999289, 47.10000000000000853, -16.24598481164532160 ) ) ;
#3533=ORIENTED_EDGE ( 'NONE', *, *, #16361, .T. ) ;
#3541=CARTESIAN_POINT ( 'NONE',  ( -3.210462471511496205E-15, 47.42187500034138736, -52.43083105670540789 ) ) ;
#3544=EDGE_CURVE ( 'NONE', #15116, #11630, #1147, .T. ) ;
#3545=CARTESIAN_POINT ( 'NONE',  ( 9.657523855033129090E-15, 36.28125000068278894, 52.57311121191334990 ) ) ;
#3546=CARTESIAN_POINT ( 'NONE',  ( 49.86468353124999453, 43.02187500034138878, -16.20201782572376459 ) ) ;
#3560=CARTESIAN_POINT ( 'NONE',  ( -30.81806926056963292, 39.55937500034139731, -42.41743335407647209 ) ) ;
#3561=CARTESIAN_POINT ( 'NONE',  ( 15.40903463028481113, 45.25937500034140015, -47.42413220539094709 ) ) ;
#3566=CARTESIAN_POINT ( 'NONE',  ( -1.240322475938754499E-13, 36.50000000000000711, 50.00000000000000000 ) ) ;
#3568=ORIENTED_EDGE ( 'NONE', *, *, #14634, .T. ) ;
#3569=ADVANCED_FACE ( 'NONE', ( #11232 ), #16377, .F. ) ;
#3574=AXIS2_PLACEMENT_3D ( 'NONE', #2074, #8009, #1608 ) ;
#3577=FILL_AREA_STYLE_COLOUR ( '', #1974 ) ;
#3583=CARTESIAN_POINT ( 'NONE',  ( 0.000000000000000000, 20.00000000000000355, 0.000000000000000000 ) ) ;
#3584=FACE_OUTER_BOUND ( 'NONE', #11947, .T. ) ;
#3587=CARTESIAN_POINT ( 'NONE',  ( 0.000000000000000000, 20.00000000000000355, 0.000000000000000000 ) ) ;
#3588=CARTESIAN_POINT ( 'NONE',  ( 30.90169943749474157, 45.08125000068279320, -42.53254041760200721 ) ) ;
#3592=CARTESIAN_POINT ( 'NONE',  ( 49.86468353125000164, 20.85937500034139802, -6.106662507704105588E-15 ) ) ;
#3605=( BOUNDED_SURFACE ( )  B_SPLINE_SURFACE ( 1, 2, ( 
 ( #8205, #15760, #11776, #4141, #14351, #543, #13273, #4388, #3133, #9124, #6651, #300, #6567, #11865, #7959, #6810, #10457, #10629, #11625, #2893, #10378, #13196, #222, #4229, #11700, #11944, #377, #5327, #5397, #15513, #14184, #9216, #2968, #465, #9452, #4308, #2800, #14269, #9373, #8116, #13032, #14508, #9298, #8036, #1800, #7876, #1634, #6729, #5479, #12953, #1557, #14424, #13109, #10551, #15607, #6892, #3044, #5635, #1714, #10700, #5568, #6968, #12103, #7294, #1872, #14836, #791, #9699, #11122, #3546, #15930, #3466, #11028, #12020, #620, #12190, #8523, #712, #5881, #5716, #2117, #10786, #10943, #9615, #4552, #7206, #13513, #14663, #869, #15852, #3293, #951, #12350, #1951, #16183, #4474, #4634, #8599, #5965, #8361, #16096, #9540, #10866, #4812, #8449, #12267, #13592, #13350, #9865, #2197, #14585, #6052, #3211, #14916, #8282, #13432, #7043, #16008, #5796, #2042, #7131, #14749, #3383, #4731, #9789, #1288, #4889, #13759, #6295, #8776, #5065, #2286, #15339, #15089, #7378, #12444, #7531, #10197, #7455, #12602, #1035, #13918, #6132, #1196, #4977, #16338, #2537, #8860, #10037, #12691, #13674, #3717, #12770, #7700, #2372, #6460, #11203, #16431, #3956, #6381, #11280, #11443, #16255, #6209, #11518, #3796, #7617, #15250, #8693, #5225, #3876, #9946, #8949, #15001, #116, #3637, #13838, #12522, #11364, #1368, #1113, #2452, #10117, #15168, #10282, #36, #5141, #14005, #2624, #1618, #4122, #361, #14085, #10687, #10441, #15741, #6877, #5625, #1452, #9108, #2784, #9031, #14335, #15497, #9280, #12937, #13094, #2701, #5384, #12848, #15670, #7777, #6711, #14167, #14406, #2875, #6544, #7858, #1543, #203, #6632, #5464, #2951, #11928, #6796, #11606, #282, #11845, #10613, #11684, #530, #11762, #10530, #4293, #5309, #9195, #14254, #7942, #10359, #15419, #1699, #15588, #4038, #13015, #9355, #450, #8100, #4213, #13178, #8018, #5551, #3029, #1784, #4370, #857, #3278, #12175, #13577, #6035, #1936, #5950, #13497, #7028, #13256, #604, #11107, #7117, #7192, #9437, #5865, #12083, #13409, #690, #4538, #2182, #774, #7278, #11011, #5783, #12254, #3119, #9525, #12335, #10850, #15915, #9601, #4711, #16076, #8512, #14571, #8346, #8191, #14648, #4617, #2023, #10928, #9773, #15992, #2104, #9681, #14819 ),
 ( #8433, #14731, #3195, #3364, #3450, #936, #6953, #14487, #1856, #12007, #5697, #10767, #15830, #4459, #8268, #13333, #8840, #16414, #4876, #9933, #11267, #7513, #12583, #11426, #3856, #14986, #13822, #9852, #8924, #3532, #5047, #12673, #10100, #15074, #16324, #11348, #6362, #6439, #4796, #8584, #1270, #12430, #11189, #2268, #5124, #13987, #4961, #8679, #19, #15152, #1022, #13900, #7365, #16167, #10177, #14904, #2359, #13658, #8761, #10021, #15227, #3703, #12751, #16242, #2435, #2605, #7441, #7681, #6118, #1099, #1180, #3616, #1348, #6277, #13745, #12508, #3777, #2515, #7597, #6193, #3939, #15319, #9012, #12829, #14068, #1431, #7758, #2684, #11500, #97, #5201, #10259, #8281, #12102, #708, #11264, #1096, #15071, #15850, #9614, #9451, #5795, #10942, #3290, #13347, #6189, #10864, #3381, #7129, #13742, #618, #7508, #4385, #8448, #4633, #3132, #16007, #9697, #14662, #14748, #7042, #9538, #13431, #16321, #7438, #13272, #12580, #3700, #15929, #1949, #2040, #4956, #4551, #12187, #5715, #2355, #12504, #4473, #14584, #8360, #790, #5880, #10017, #8757, #3209, #13819, #14504, #2431, #8204, #1177, #10699, #15757, #1870, #6966, #12019, #10783, #12995, #11345, #15148, #2761, #2512, #1267, #8833, #11665, #10422, #11497, #15223, #1521, #11577, #7591, #4019, #13897, #6272, #7837, #16411, #8918, #5044, #15316, #6436, #5366, #5197, #2852, #6359, #3936, #9169, #13984, #6610, #10097, #7678, #2681, #10173, #261, #9008, #12911, #12670, #14065, #10253, #1345, #2601, #12748, #3774, #11423, #7919, #7755, #9088, #16, #12825, #94, #1428, #5120, #3853, #15476, #6518, #4098, #183, #5287, #14227, #10338, #15399, #14145, #1810, #15447, #2816, #1569, #5411, #10469, #4319, #10639, #8134, #9137, #2904, #2728, #15527, #4241, #13044, #6662, #15691, #4157, #13120, #390, #6824, #10391, #553, #14113, #1727, #14361, #12878, #9308, #2978, #7972, #8048, #311, #7890, #6743, #9384, #475, #6581, #5646, #13206, #9229, #11712, #11790, #14434, #14282, #5494, #4065, #11877, #5578, #14196, #12965, #1646, #10563, #15616, #3057, #6901, #11955, #10712, #7806, #3988, #1484, #9060, #11638, #232, #5339, #15940, #10955, #5975, #6064, #4398, #8215, #12279, #12030, #10802, #1885, #4743, #3479, #4562, #8293, #11041, #4648, #632 ) ),
 .UNSPECIFIED., .F., .F., .T. ) 
 B_SPLINE_SURFACE_WITH_KNOTS ( ( 2, 2 ),
 ( 3, 2, 2, 2, 2, 2, 2, 2, 2, 2, 2, 2, 2, 2, 2, 2, 2, 2, 2, 2, 2, 2, 2, 2, 2, 2, 2, 2, 2, 2, 2, 2, 2, 2, 2, 2, 2, 2, 2, 2, 2, 2, 2, 2, 2, 2, 2, 2, 2, 2, 2, 2, 2, 2, 2, 2, 2, 2, 2, 2, 2, 2, 2, 2, 2, 2, 2, 2, 2, 2, 2, 2, 2, 2, 2, 2, 2, 2, 2, 2, 2, 2, 2, 2, 2, 2, 2, 2, 2, 2, 2, 2, 2, 2, 2, 2, 2, 2, 2, 2, 2, 2, 2, 2, 2, 2, 2, 2, 2, 2, 2, 2, 2, 2, 2, 2, 2, 2, 2, 2, 2, 2, 2, 2, 2, 2, 2, 2, 2, 2, 2, 2, 2, 2, 2, 2, 2, 2, 2, 2, 2, 2, 2, 2, 2, 2, 2, 2, 2, 2, 3 ),
 ( 0.000000000000000000, 1.000000000000000000 ),
 ( 0.000000000000000000, 0.006666666666666667095, 0.01333333333333333419, 0.02000000000000000042, 0.02666666666666666838, 0.03333333333333333287, 0.04000000000000000083, 0.04666666666666666879, 0.05333333333333333676, 0.05999999999999999778, 0.06666666666666666574, 0.07333333333333333370, 0.08000000000000000167, 0.08666666666666666963, 0.09333333333333333759, 0.1000000000000000056, 0.1066666666666666735, 0.1133333333333333276, 0.1199999999999999956, 0.1266666666666666774, 0.1333333333333333315, 0.1400000000000000133, 0.1466666666666666674, 0.1533333333333333215, 0.1600000000000000033, 0.1666666666666666574, 0.1733333333333333393, 0.1799999999999999933, 0.1866666666666666752, 0.1933333333333333293, 0.2000000000000000111, 0.2066666666666666652, 0.2133333333333333470, 0.2200000000000000011, 0.2266666666666666552, 0.2333333333333333370, 0.2399999999999999911, 0.2466666666666666730, 0.2533333333333333548, 0.2600000000000000089, 0.2666666666666666630, 0.2733333333333333171, 0.2800000000000000266, 0.2866666666666666807, 0.2933333333333333348, 0.2999999999999999889, 0.3066666666666666430, 0.3133333333333333526, 0.3200000000000000067, 0.3266666666666666607, 0.3333333333333333148, 0.3400000000000000244, 0.3466666666666666785, 0.3533333333333333326, 0.3599999999999999867, 0.3666666666666666408, 0.3733333333333333504, 0.3800000000000000044, 0.3866666666666666585, 0.3933333333333333126, 0.4000000000000000222, 0.4066666666666666763, 0.4133333333333333304, 0.4199999999999999845, 0.4266666666666666941, 0.4333333333333333481, 0.4400000000000000022, 0.4466666666666666563, 0.4533333333333333104, 0.4600000000000000200, 0.4666666666666666741, 0.4733333333333333282, 0.4799999999999999822, 0.4866666666666666918, 0.4933333333333333459, 0.5000000000000000000, 0.5066666666666667096, 0.5133333333333333082, 0.5200000000000000178, 0.5266666666666666163, 0.5333333333333333259, 0.5400000000000000355, 0.5466666666666666341, 0.5533333333333333437, 0.5600000000000000533, 0.5666666666666666519, 0.5733333333333333615, 0.5799999999999999600, 0.5866666666666666696, 0.5933333333333333792, 0.5999999999999999778, 0.6066666666666666874, 0.6133333333333332860, 0.6199999999999999956, 0.6266666666666667052, 0.6333333333333333037, 0.6400000000000000133, 0.6466666666666666119, 0.6533333333333333215, 0.6600000000000000311, 0.6666666666666666297, 0.6733333333333333393, 0.6800000000000000488, 0.6866666666666666474, 0.6933333333333333570, 0.6999999999999999556, 0.7066666666666666652, 0.7133333333333333748, 0.7199999999999999734, 0.7266666666666666829, 0.7333333333333332815, 0.7399999999999999911, 0.7466666666666667007, 0.7533333333333332993, 0.7600000000000000089, 0.7666666666666667185, 0.7733333333333333171, 0.7800000000000000266, 0.7866666666666666252, 0.7933333333333333348, 0.8000000000000000444, 0.8066666666666666430, 0.8133333333333333526, 0.8199999999999999512, 0.8266666666666666607, 0.8333333333333333703, 0.8399999999999999689, 0.8466666666666666785, 0.8533333333333333881, 0.8599999999999999867, 0.8666666666666666963, 0.8733333333333332948, 0.8800000000000000044, 0.8866666666666667140, 0.8933333333333333126, 0.9000000000000000222, 0.9066666666666666208, 0.9133333333333333304, 0.9200000000000000400, 0.9266666666666666385, 0.9333333333333333481, 0.9399999999999999467, 0.9466666666666666563, 0.9533333333333333659, 0.9599999999999999645, 0.9666666666666666741, 0.9733333333333333837, 0.9799999999999999822, 0.9866666666666666918, 0.9933333333333332904, 1.000000000000000000 ),
 .UNSPECIFIED. ) 
 GEOMETRIC_REPRESENTATION_ITEM ( )  RATIONAL_B_SPLINE_SURFACE ( (
 ( 1.000000000000000000, 0.9510565162951535312, 1.000000000000000000, 0.9510565162951535312, 1.000000000000000000, 0.9510565162951535312, 1.000000000000000000, 0.9510565162951535312, 1.000000000000000000, 0.9510565162951535312, 1.000000000000000000, 0.9510565162951535312, 1.000000000000000000, 0.9510565162951535312, 1.000000000000000000, 0.9510565162951535312, 1.000000000000000000, 0.9510565162951535312, 1.000000000000000000, 0.9510565162951535312, 1.000000000000000000, 0.9510565162951535312, 1.000000000000000000, 0.9510565162951535312, 1.000000000000000000, 0.9510565162951535312, 1.000000000000000000, 0.9510565162951535312, 1.000000000000000000, 0.9510565162951535312, 1.000000000000000000, 0.9510565162951535312, 1.000000000000000000, 0.9510565162951535312, 1.000000000000000000, 0.9510565162951535312, 1.000000000000000000, 0.9510565162951535312, 1.000000000000000000, 0.9510565162951535312, 1.000000000000000000, 0.9510565162951535312, 1.000000000000000000, 0.9510565162951535312, 1.000000000000000000, 0.9510565162951535312, 1.000000000000000000, 0.9510565162951535312, 1.000000000000000000, 0.9510565162951535312, 1.000000000000000000, 0.9510565162951535312, 1.000000000000000000, 0.9510565162951535312, 1.000000000000000000, 0.9510565162951535312, 1.000000000000000000, 0.9510565162951535312, 1.000000000000000000, 0.9510565162951535312, 1.000000000000000000, 0.9510565162951535312, 1.000000000000000000, 0.9510565162951535312, 1.000000000000000000, 0.9510565162951535312, 1.000000000000000000, 0.9510565162951535312, 1.000000000000000000, 0.9510565162951535312, 1.000000000000000000, 0.9510565162951535312, 1.000000000000000000, 0.9510565162951535312, 1.000000000000000000, 0.9510565162951535312, 1.000000000000000000, 0.9510565162951535312, 1.000000000000000000, 0.9510565162951535312, 1.000000000000000000, 0.9510565162951535312, 1.000000000000000000, 0.9510565162951535312, 1.000000000000000000, 0.9510565162951535312, 1.000000000000000000, 0.9510565162951535312, 1.000000000000000000, 0.9510565162951535312, 1.000000000000000000, 0.9510565162951535312, 1.000000000000000000, 0.9510565162951535312, 1.000000000000000000, 0.9510565162951535312, 1.000000000000000000, 0.9510565162951535312, 1.000000000000000000, 0.9510565162951535312, 1.000000000000000000, 0.9510565162951535312, 1.000000000000000000, 0.9510565162951535312, 1.000000000000000000, 0.9510565162951535312, 1.000000000000000000, 0.9510565162951535312, 1.000000000000000000, 0.9510565162951535312, 1.000000000000000000, 0.9510565162951535312, 1.000000000000000000, 0.9510565162951535312, 1.000000000000000000, 0.9510565162951535312, 1.000000000000000000, 0.9510565162951535312, 1.000000000000000000, 0.9510565162951535312, 1.000000000000000000, 0.9510565162951535312, 1.000000000000000000, 0.9510565162951535312, 1.000000000000000000, 0.9510565162951535312, 1.000000000000000000, 0.9510565162951535312, 1.000000000000000000, 0.9510565162951535312, 1.000000000000000000, 0.9510565162951535312, 1.000000000000000000, 0.9510565162951535312, 1.000000000000000000, 0.9510565162951535312, 1.000000000000000000, 0.9510565162951535312, 1.000000000000000000, 0.9510565162951535312, 1.000000000000000000, 0.9510565162951535312, 1.000000000000000000, 0.9510565162951535312, 1.000000000000000000, 0.9510565162951535312, 1.000000000000000000, 0.9510565162951535312, 1.000000000000000000, 0.9510565162951535312, 1.000000000000000000, 0.9510565162951535312, 1.000000000000000000, 0.9510565162951535312, 1.000000000000000000, 0.9510565162951535312, 1.000000000000000000, 0.9510565162951535312, 1.000000000000000000, 0.9510565162951535312, 1.000000000000000000, 0.9510565162951535312, 1.000000000000000000, 0.9510565162951535312, 1.000000000000000000, 0.9510565162951535312, 1.000000000000000000, 0.9510565162951535312, 1.000000000000000000, 0.9510565162951535312, 1.000000000000000000, 0.9510565162951535312, 1.000000000000000000, 0.9510565162951535312, 1.000000000000000000, 0.9510565162951535312, 1.000000000000000000, 0.9510565162951535312, 1.000000000000000000, 0.9510565162951535312, 1.000000000000000000, 0.9510565162951535312, 1.000000000000000000, 0.9510565162951535312, 1.000000000000000000, 0.9510565162951535312, 1.000000000000000000, 0.9510565162951535312, 1.000000000000000000, 0.9510565162951535312, 1.000000000000000000, 0.9510565162951535312, 1.000000000000000000, 0.9510565162951535312, 1.000000000000000000, 0.9510565162951535312, 1.000000000000000000, 0.9510565162951535312, 1.000000000000000000, 0.9510565162951535312, 1.000000000000000000, 0.9510565162951535312, 1.000000000000000000, 0.9510565162951535312, 1.000000000000000000, 0.9510565162951535312, 1.000000000000000000, 0.9510565162951535312, 1.000000000000000000, 0.9510565162951535312, 1.000000000000000000, 0.9510565162951535312, 1.000000000000000000, 0.9510565162951535312, 1.000000000000000000, 0.9510565162951535312, 1.000000000000000000, 0.9510565162951535312, 1.000000000000000000, 0.9510565162951535312, 1.000000000000000000, 0.9510565162951535312, 1.000000000000000000, 0.9510565162951535312, 1.000000000000000000, 0.9510565162951535312, 1.000000000000000000, 0.9510565162951535312, 1.000000000000000000, 0.9510565162951535312, 1.000000000000000000, 0.9510565162951535312, 1.000000000000000000, 0.9510565162951535312, 1.000000000000000000, 0.9510565162951535312, 1.000000000000000000, 0.9510565162951535312, 1.000000000000000000, 0.9510565162951535312, 1.000000000000000000, 0.9510565162951535312, 1.000000000000000000, 0.9510565162951535312, 1.000000000000000000, 0.9510565162951535312, 1.000000000000000000, 0.9510565162951535312, 1.000000000000000000, 0.9510565162951535312, 1.000000000000000000, 0.9510565162951535312, 1.000000000000000000, 0.9510565162951535312, 1.000000000000000000, 0.9510565162951535312, 1.000000000000000000, 0.9510565162951535312, 1.000000000000000000, 0.9510565162951535312, 1.000000000000000000, 0.9510565162951535312, 1.000000000000000000, 0.9510565162951535312, 1.000000000000000000, 0.9510565162951535312, 1.000000000000000000, 0.9510565162951535312, 1.000000000000000000, 0.9510565162951535312, 1.000000000000000000, 0.9510565162951535312, 1.000000000000000000, 0.9510565162951535312, 1.000000000000000000, 0.9510565162951535312, 1.000000000000000000, 0.9510565162951535312, 1.000000000000000000, 0.9510565162951535312, 1.000000000000000000, 0.9510565162951535312, 1.000000000000000000, 0.9510565162951535312, 1.000000000000000000, 0.9510565162951535312, 1.000000000000000000, 0.9510565162951535312, 1.000000000000000000, 0.9510565162951535312, 1.000000000000000000, 0.9510565162951535312, 1.000000000000000000, 0.9510565162951535312, 1.000000000000000000, 0.9510565162951535312, 1.000000000000000000, 0.9510565162951535312, 1.000000000000000000, 0.9510565162951535312, 1.000000000000000000),
 ( 1.000000000000000000, 0.9510565162951535312, 1.000000000000000000, 0.9510565162951535312, 1.000000000000000000, 0.9510565162951535312, 1.000000000000000000, 0.9510565162951535312, 1.000000000000000000, 0.9510565162951535312, 1.000000000000000000, 0.9510565162951535312, 1.000000000000000000, 0.9510565162951535312, 1.000000000000000000, 0.9510565162951535312, 1.000000000000000000, 0.9510565162951535312, 1.000000000000000000, 0.9510565162951535312, 1.000000000000000000, 0.9510565162951535312, 1.000000000000000000, 0.9510565162951535312, 1.000000000000000000, 0.9510565162951535312, 1.000000000000000000, 0.9510565162951535312, 1.000000000000000000, 0.9510565162951535312, 1.000000000000000000, 0.9510565162951535312, 1.000000000000000000, 0.9510565162951535312, 1.000000000000000000, 0.9510565162951535312, 1.000000000000000000, 0.9510565162951535312, 1.000000000000000000, 0.9510565162951535312, 1.000000000000000000, 0.9510565162951535312, 1.000000000000000000, 0.9510565162951535312, 1.000000000000000000, 0.9510565162951535312, 1.000000000000000000, 0.9510565162951535312, 1.000000000000000000, 0.9510565162951535312, 1.000000000000000000, 0.9510565162951535312, 1.000000000000000000, 0.9510565162951535312, 1.000000000000000000, 0.9510565162951535312, 1.000000000000000000, 0.9510565162951535312, 1.000000000000000000, 0.9510565162951535312, 1.000000000000000000, 0.9510565162951535312, 1.000000000000000000, 0.9510565162951535312, 1.000000000000000000, 0.9510565162951535312, 1.000000000000000000, 0.9510565162951535312, 1.000000000000000000, 0.9510565162951535312, 1.000000000000000000, 0.9510565162951535312, 1.000000000000000000, 0.9510565162951535312, 1.000000000000000000, 0.9510565162951535312, 1.000000000000000000, 0.9510565162951535312, 1.000000000000000000, 0.9510565162951535312, 1.000000000000000000, 0.9510565162951535312, 1.000000000000000000, 0.9510565162951535312, 1.000000000000000000, 0.9510565162951535312, 1.000000000000000000, 0.9510565162951535312, 1.000000000000000000, 0.9510565162951535312, 1.000000000000000000, 0.9510565162951535312, 1.000000000000000000, 0.9510565162951535312, 1.000000000000000000, 0.9510565162951535312, 1.000000000000000000, 0.9510565162951535312, 1.000000000000000000, 0.9510565162951535312, 1.000000000000000000, 0.9510565162951535312, 1.000000000000000000, 0.9510565162951535312, 1.000000000000000000, 0.9510565162951535312, 1.000000000000000000, 0.9510565162951535312, 1.000000000000000000, 0.9510565162951535312, 1.000000000000000000, 0.9510565162951535312, 1.000000000000000000, 0.9510565162951535312, 1.000000000000000000, 0.9510565162951535312, 1.000000000000000000, 0.9510565162951535312, 1.000000000000000000, 0.9510565162951535312, 1.000000000000000000, 0.9510565162951535312, 1.000000000000000000, 0.9510565162951535312, 1.000000000000000000, 0.9510565162951535312, 1.000000000000000000, 0.9510565162951535312, 1.000000000000000000, 0.9510565162951535312, 1.000000000000000000, 0.9510565162951535312, 1.000000000000000000, 0.9510565162951535312, 1.000000000000000000, 0.9510565162951535312, 1.000000000000000000, 0.9510565162951535312, 1.000000000000000000, 0.9510565162951535312, 1.000000000000000000, 0.9510565162951535312, 1.000000000000000000, 0.9510565162951535312, 1.000000000000000000, 0.9510565162951535312, 1.000000000000000000, 0.9510565162951535312, 1.000000000000000000, 0.9510565162951535312, 1.000000000000000000, 0.9510565162951535312, 1.000000000000000000, 0.9510565162951535312, 1.000000000000000000, 0.9510565162951535312, 1.000000000000000000, 0.9510565162951535312, 1.000000000000000000, 0.9510565162951535312, 1.000000000000000000, 0.9510565162951535312, 1.000000000000000000, 0.9510565162951535312, 1.000000000000000000, 0.9510565162951535312, 1.000000000000000000, 0.9510565162951535312, 1.000000000000000000, 0.9510565162951535312, 1.000000000000000000, 0.9510565162951535312, 1.000000000000000000, 0.9510565162951535312, 1.000000000000000000, 0.9510565162951535312, 1.000000000000000000, 0.9510565162951535312, 1.000000000000000000, 0.9510565162951535312, 1.000000000000000000, 0.9510565162951535312, 1.000000000000000000, 0.9510565162951535312, 1.000000000000000000, 0.9510565162951535312, 1.000000000000000000, 0.9510565162951535312, 1.000000000000000000, 0.9510565162951535312, 1.000000000000000000, 0.9510565162951535312, 1.000000000000000000, 0.9510565162951535312, 1.000000000000000000, 0.9510565162951535312, 1.000000000000000000, 0.9510565162951535312, 1.000000000000000000, 0.9510565162951535312, 1.000000000000000000, 0.9510565162951535312, 1.000000000000000000, 0.9510565162951535312, 1.000000000000000000, 0.9510565162951535312, 1.000000000000000000, 0.9510565162951535312, 1.000000000000000000, 0.9510565162951535312, 1.000000000000000000, 0.9510565162951535312, 1.000000000000000000, 0.9510565162951535312, 1.000000000000000000, 0.9510565162951535312, 1.000000000000000000, 0.9510565162951535312, 1.000000000000000000, 0.9510565162951535312, 1.000000000000000000, 0.9510565162951535312, 1.000000000000000000, 0.9510565162951535312, 1.000000000000000000, 0.9510565162951535312, 1.000000000000000000, 0.9510565162951535312, 1.000000000000000000, 0.9510565162951535312, 1.000000000000000000, 0.9510565162951535312, 1.000000000000000000, 0.9510565162951535312, 1.000000000000000000, 0.9510565162951535312, 1.000000000000000000, 0.9510565162951535312, 1.000000000000000000, 0.9510565162951535312, 1.000000000000000000, 0.9510565162951535312, 1.000000000000000000, 0.9510565162951535312, 1.000000000000000000, 0.9510565162951535312, 1.000000000000000000, 0.9510565162951535312, 1.000000000000000000, 0.9510565162951535312, 1.000000000000000000, 0.9510565162951535312, 1.000000000000000000, 0.9510565162951535312, 1.000000000000000000, 0.9510565162951535312, 1.000000000000000000, 0.9510565162951535312, 1.000000000000000000, 0.9510565162951535312, 1.000000000000000000, 0.9510565162951535312, 1.000000000000000000, 0.9510565162951535312, 1.000000000000000000, 0.9510565162951535312, 1.000000000000000000, 0.9510565162951535312, 1.000000000000000000, 0.9510565162951535312, 1.000000000000000000, 0.9510565162951535312, 1.000000000000000000, 0.9510565162951535312, 1.000000000000000000, 0.9510565162951535312, 1.000000000000000000, 0.9510565162951535312, 1.000000000000000000, 0.9510565162951535312, 1.000000000000000000, 0.9510565162951535312, 1.000000000000000000, 0.9510565162951535312, 1.000000000000000000, 0.9510565162951535312, 1.000000000000000000, 0.9510565162951535312, 1.000000000000000000, 0.9510565162951535312, 1.000000000000000000, 0.9510565162951535312, 1.000000000000000000, 0.9510565162951535312, 1.000000000000000000, 0.9510565162951535312, 1.000000000000000000, 0.9510565162951535312, 1.000000000000000000, 0.9510565162951535312, 1.000000000000000000) ) ) 
 REPRESENTATION_ITEM ( '' )  SURFACE ( )  );
#3606=CARTESIAN_POINT ( 'NONE',  ( 7.513064459987437071E-14, 42.28125000068280315, 50.00000000000000000 ) ) ;
#3608=CARTESIAN_POINT ( 'NONE',  ( -15.40903463028480580, 20.32187500034139660, 47.42413220539094709 ) ) ;
#3609=CARTESIAN_POINT ( 'NONE',  ( 15.40903463028482356, 32.45937500034138878, 47.42413220539093999 ) ) ;
#3610=CARTESIAN_POINT ( 'NONE',  ( 17.50000000000000000, 22.50000000000000355, 80.00000000000000000 ) ) ;
#3611=CARTESIAN_POINT ( 'NONE',  ( 30.81806926056964002, 32.62187500034140442, 42.41743335407646498 ) ) ;
#3613=CARTESIAN_POINT ( 'NONE',  ( -49.86468353124999453, 41.75937500034139305, -16.20201782572375393 ) ) ;
#3616=CARTESIAN_POINT ( 'NONE',  ( 50.00000000000000711, 42.89999999999999858, 16.24598481164530739 ) ) ;
#3629=CARTESIAN_POINT ( 'NONE',  ( 49.86468353125001585, 42.82187500034139305, 16.20201782572375038 ) ) ;
#3631=FACE_OUTER_BOUND ( 'NONE', #1957, .T. ) ;
#3635=CARTESIAN_POINT ( 'NONE',  ( -50.00000000000000000, 25.78125000068279959, 0.000000000000000000 ) ) ;
#3637=CARTESIAN_POINT ( 'NONE',  ( 9.631387414534489405E-15, 32.42187500034139447, 52.43083105670540789 ) ) ;
#3643=ORIENTED_EDGE ( 'NONE', *, *, #2037, .T. ) ;
#3645=EDGE_LOOP ( 'NONE', ( #7472, #10327, #10768, #13301 ) ) ;
#3648=CARTESIAN_POINT ( 'NONE',  ( -40.45084971874737079, 23.98125000068279888, 29.38926261462367151 ) ) ;
#3650=CARTESIAN_POINT ( 'NONE',  ( -30.81806926056962226, 32.15937500034139873, 42.41743335407647919 ) ) ;
#3651=CARTESIAN_POINT ( 'NONE',  ( 9.631387414534489405E-15, 40.35937500034139447, 52.43083105670540789 ) ) ;
#3665=ORIENTED_EDGE ( 'NONE', *, *, #3967, .F. ) ;
#3668=CARTESIAN_POINT ( 'NONE',  ( -7.919222016226934890, 20.44874571845315714, 49.99999999999996447 ) ) ;
#3672=EDGE_CURVE ( 'NONE', #6301, #5249, #16457, .T. ) ;
#3675=DIRECTION ( 'NONE',  ( -0.000000000000000000, 1.000000000000000000, -0.000000000000000000 ) ) ;
#3677=CARTESIAN_POINT ( 'NONE',  ( 15.45084971874736723, 45.18125000068280173, -47.55282581475768211 ) ) ;
#3679=CARTESIAN_POINT ( 'NONE',  ( -49.99999999999999289, 25.89999999999999858, -16.24598481164531449 ) ) ;
#3682=EDGE_CURVE ( 'NONE', #14909, #383, #7971, .T. ) ;
#3694=CARTESIAN_POINT ( 'NONE',  ( 0.000000000000000000, 50.00000000000000000, 50.00000000000000000 ) ) ;
#3695=CARTESIAN_POINT ( 'NONE',  ( -15.40903463028481646, 25.52187500034139589, -47.42413220539093999 ) ) ;
#3696=CARTESIAN_POINT ( 'NONE',  ( 40.34137639590981905, 22.65937500034139518, 29.30972558990010768 ) ) ;
#3697=CARTESIAN_POINT ( 'NONE',  ( 0.000000000000000000, 50.00000000000000000, 0.000000000000000000 ) ) ;
#3698=CARTESIAN_POINT ( 'NONE',  ( 15.40903463028481113, 33.32187500034139305, -47.42413220539094709 ) ) ;
#3700=CARTESIAN_POINT ( 'NONE',  ( 30.90169943749474157, 37.30000000000000426, -42.53254041760200721 ) ) ;
#3701=CARTESIAN_POINT ( 'NONE',  ( -40.34137639590981905, 41.65937500034139873, -29.30972558990011478 ) ) ;
#3703=CARTESIAN_POINT ( 'NONE',  ( -49.99999999999999289, 43.90000000000000568, -16.24598481164531449 ) ) ;
#3708=( BOUNDED_CURVE ( )  B_SPLINE_CURVE ( 2, ( #3375, #2281, #6126, #5790, #13504, #16249, #5957, #3457, #12436, #11196, #14994, #2033, #1029 ),
 .UNSPECIFIED., .F., .F. ) 
 B_SPLINE_CURVE_WITH_KNOTS ( ( 3, 2, 2, 2, 2, 2, 3 ),
 ( 0.2833333333333333814, 0.2866666666666666807, 0.2933333333333333348, 0.2999999999999999889, 0.3066666666666666430, 0.3133333333333333526, 0.3166666666666667074 ),
 .UNSPECIFIED. ) 
 CURVE ( )  GEOMETRIC_REPRESENTATION_ITEM ( )  RATIONAL_B_SPLINE_CURVE ( ( 0.9755282581475768211, 0.9755282581475770431, 1.000000000000000000, 0.9510565162951535312, 1.000000000000000000, 0.9510565162951535312, 1.000000000000000000, 0.9510565162951535312, 1.000000000000000000, 0.9510565162951535312, 1.000000000000000000, 0.9755282581475765991, 0.9755282581475768211 ) ) 
 REPRESENTATION_ITEM ( '' )  );
#3712=CARTESIAN_POINT ( 'NONE',  ( -49.86468353124999453, 44.02187500034139589, 16.20201782572377525 ) ) ;
#3715=CARTESIAN_POINT ( 'NONE',  ( 40.45084971874737789, 28.58125000068280031, 29.38926261462365375 ) ) ;
#3717=CARTESIAN_POINT ( 'NONE',  ( 49.86468353125001585, 34.82187500034140015, 16.20201782572375038 ) ) ;
#3723=ADVANCED_FACE ( 'NONE', ( #8047 ), #7699, .T. ) ;
#3728=CARTESIAN_POINT ( 'NONE',  ( 40.34137639590981905, 32.65937500034139873, 29.30972558990010768 ) ) ;
#3729=CARTESIAN_POINT ( 'NONE',  ( -15.40903463028480580, 46.32187500034140015, 47.42413220539094709 ) ) ;
#3737=ORIENTED_EDGE ( 'NONE', *, *, #3374, .T. ) ;
#3743=CARTESIAN_POINT ( 'NONE',  ( -30.81806926056963292, 47.55937500034139731, -42.41743335407647209 ) ) ;
#3748=SHAPE_REPRESENTATION_RELATIONSHIP ( 'NONE' , 'NONE' ,  #9477, #3231 ) ;
#3750=CARTESIAN_POINT ( 'NONE',  ( 50.00000000000000711, 46.68125000068278752, 16.24598481164530739 ) ) ;
#3752=EDGE_CURVE ( 'NONE', #4896, #12984, #14596, .T. ) ;
#3753=CARTESIAN_POINT ( 'NONE',  ( 15.45084971874736723, 47.18125000068280173, -47.55282581475768211 ) ) ;
#3760=ORIENTED_EDGE ( 'NONE', *, *, #14987, .T. ) ;
#3764=CARTESIAN_POINT ( 'NONE',  ( -17.50000000000000000, 22.50000000000000000, 94.42467108177066848 ) ) ;
#3768=CARTESIAN_POINT ( 'NONE',  ( 2.600676159226421000E-13, 33.49999999999999289, -49.99999999999999289 ) ) ;
#3769=CARTESIAN_POINT ( 'NONE',  ( 49.86468353124999453, 25.02187500034139589, -16.20201782572376459 ) ) ;
#3770=CARTESIAN_POINT ( 'NONE',  ( 30.81806926056962936, 23.15937500034139518, -42.41743335407646498 ) ) ;
#3772=CARTESIAN_POINT ( 'NONE',  ( 49.86468353125001585, 34.82187500034139305, 16.20201782572375038 ) ) ;
#3774=CARTESIAN_POINT ( 'NONE',  ( -50.00000000000000000, 30.00000000000000355, 0.000000000000000000 ) ) ;
#3775=CARTESIAN_POINT ( 'NONE',  ( 49.86468353125000164, 40.85937500034139447, -6.106662507704105588E-15 ) ) ;
#3777=CARTESIAN_POINT ( 'NONE',  ( -15.45084971874736368, 42.39999999999999858, 47.55282581475768211 ) ) ;
#3779=EDGE_CURVE ( 'NONE', #1788, #8741, #3220, .T. ) ;
#3788=EDGE_CURVE ( 'NONE', #4733, #10001, #1884, .T. ) ;
#3789=CARTESIAN_POINT ( 'NONE',  ( -40.34137639590981905, 39.72187500034139873, -29.30972558990011478 ) ) ;
#3794=CARTESIAN_POINT ( 'NONE',  ( 50.00000000000000711, 28.68125000068279462, 16.24598481164530739 ) ) ;
#3796=CARTESIAN_POINT ( 'NONE',  ( -3.210462471511496205E-15, 33.42187500034140157, -52.43083105670540789 ) ) ;
#3806=CARTESIAN_POINT ( 'NONE',  ( 49.86468353125001585, 32.75937500034140015, 16.20201782572375038 ) ) ;
#3809=CARTESIAN_POINT ( 'NONE',  ( 15.40903463028481113, 45.32187500034140015, -47.42413220539094709 ) ) ;
#3821=CARTESIAN_POINT ( 'NONE',  ( 50.00000000000000711, 34.68125000068279462, 16.24598481164530739 ) ) ;
#3831=CARTESIAN_POINT ( 'NONE',  ( 50.00000000000000711, 44.68125000068278752, 16.24598481164530739 ) ) ;
#3832=CARTESIAN_POINT ( 'NONE',  ( 50.00000000000000711, 44.68125000068278752, 16.24598481164530739 ) ) ;
#3835=ORIENTED_EDGE ( 'NONE', *, *, #3779, .T. ) ;
#3836=AXIS2_PLACEMENT_3D ( 'NONE', #6300, #9197, #11445 ) ;
#3849=CARTESIAN_POINT ( 'NONE',  ( 30.81806926056964002, 24.55937500034139376, 42.41743335407646498 ) ) ;
#3851=CARTESIAN_POINT ( 'NONE',  ( -30.81806926056962226, 36.22187500034139163, 42.41743335407647209 ) ) ;
#3853=CARTESIAN_POINT ( 'NONE',  ( 50.00000000000000000, 29.00000000000000000, -6.123233995736766085E-15 ) ) ;
#3854=CARTESIAN_POINT ( 'NONE',  ( 49.86468353124999453, 38.95937500034139589, -16.20201782572376459 ) ) ;
#3856=CARTESIAN_POINT ( 'NONE',  ( -15.45084971874737256, 47.60000000000000142, -47.55282581475767500 ) ) ;
#3868=CARTESIAN_POINT ( 'NONE',  ( -30.81806926056963292, 43.62187500034139020, -42.41743335407647209 ) ) ;
#3873=CARTESIAN_POINT ( 'NONE',  ( -40.45084971874737079, 25.98125000068279888, 29.38926261462367151 ) ) ;
#3874=CARTESIAN_POINT ( 'NONE',  ( 4.539827090575156987, 39.41081929220959523, 92.94164601386977154 ) ) ;
#3876=CARTESIAN_POINT ( 'NONE',  ( 49.86468353125000164, 32.92187500034139447, -6.106662507704105588E-15 ) ) ;
#3888=CARTESIAN_POINT ( 'NONE',  ( 30.81806926056964002, 28.55937500034139731, 42.41743335407647209 ) ) ;
#3890=CARTESIAN_POINT ( 'NONE',  ( -3.210462471511496205E-15, 47.42187500034138736, -52.43083105670540789 ) ) ;
#3899=ORIENTED_EDGE ( 'NONE', *, *, #14634, .F. ) ;
#3902=CARTESIAN_POINT ( 'NONE',  ( -30.90169943749474513, 45.48125000068279178, -42.53254041760200721 ) ) ;
#3905=CARTESIAN_POINT ( 'NONE',  ( 40.45084971874737079, 34.98125000068279888, -29.38926261462366440 ) ) ;
#3910=CARTESIAN_POINT ( 'NONE',  ( 30.81806926056962936, 49.15937500034138452, -42.41743335407647209 ) ) ;
#3913=CARTESIAN_POINT ( 'NONE',  ( 40.45084971874737789, 24.58125000068280031, 29.38926261462365375 ) ) ;
#3915=CARTESIAN_POINT ( 'NONE',  ( 30.90169943749474157, 43.08125000068280031, -42.53254041760200721 ) ) ;
#3916=CARTESIAN_POINT ( 'NONE',  ( 7.919222016226791006, 44.33250428222964246, 50.00000000000000711 ) ) ;
#3921=ORIENTED_EDGE ( 'NONE', *, *, #4905, .F. ) ;
#3922=DIRECTION ( 'NONE',  ( -1.000000000000000000, 0.000000000000000000, 0.000000000000000000 ) ) ;
#3928=CARTESIAN_POINT ( 'NONE',  ( -8.798974116419094216, 37.67024782698770480, 92.94692907539341320 ) ) ;
#3932=CARTESIAN_POINT ( 'NONE',  ( -40.34137639590981905, 25.65937500034139518, -29.30972558990011478 ) ) ;
#3934=CARTESIAN_POINT ( 'NONE',  ( 49.86468353124999453, 31.02187500034139589, -16.20201782572376104 ) ) ;
#3936=CARTESIAN_POINT ( 'NONE',  ( -30.90169943749474868, 31.70000000000000639, -42.53254041760200721 ) ) ;
#3937=CARTESIAN_POINT ( 'NONE',  ( -40.34137639590981195, 40.05937500034140442, 29.30972558990012189 ) ) ;
#3939=CARTESIAN_POINT ( 'NONE',  ( -50.00000000000000000, 42.00000000000000000, 0.000000000000000000 ) ) ;
#3950=CARTESIAN_POINT ( 'NONE',  ( 49.86468353125000164, 40.92187500034139447, -6.106662507704105588E-15 ) ) ;
#3951=CARTESIAN_POINT ( 'NONE',  ( -3.210462471511496205E-15, 39.35937500034138736, -52.43083105670540789 ) ) ;
#3954=CARTESIAN_POINT ( 'NONE',  ( 9.657523855033129090E-15, 26.28125000068279604, 52.57311121191334990 ) ) ;
#3955=CARTESIAN_POINT ( 'NONE',  ( -50.00000000000000000, 35.78125000068280315, 0.000000000000000000 ) ) ;
#3956=CARTESIAN_POINT ( 'NONE',  ( -40.34137639590981195, 34.12187500034139731, 29.30972558990012189 ) ) ;
#3964=CARTESIAN_POINT ( 'NONE',  ( -30.90169943749473447, 24.29999999999999716, 42.53254041760200721 ) ) ;
#3966=CARTESIAN_POINT ( 'NONE',  ( -40.34137639590981195, 32.05937500034139731, 29.30972558990012189 ) ) ;
#3967=EDGE_CURVE ( 'NONE', #15517, #6639, #5803, .T. ) ;
#3970=CARTESIAN_POINT ( 'NONE',  ( 30.81806926056962936, 49.22187500034139873, -42.41743335407646498 ) ) ;
#3975=EDGE_CURVE ( 'NONE', #11191, #10619, #16224, .T. ) ;
#3983=EDGE_CURVE ( 'NONE', #8741, #15936, #3158, .T. ) ;
#3988=CARTESIAN_POINT ( 'NONE',  ( -40.45084971874737079, 22.19999999999999929, 29.38926261462367151 ) ) ;
#3989=CARTESIAN_POINT ( 'NONE',  ( -49.86468353125000164, 47.85937500034139447, 0.000000000000000000 ) ) ;
#3991=CARTESIAN_POINT ( 'NONE',  ( -15.45084971874736368, 26.18125000068280173, 47.55282581475768211 ) ) ;
#3993=( NAMED_UNIT ( * ) SI_UNIT ( $, .STERADIAN. ) SOLID_ANGLE_UNIT ( ) );
#3995=CARTESIAN_POINT ( 'NONE',  ( -15.45084971874736368, 38.18125000068280173, 47.55282581475768211 ) ) ;
#4002=VERTEX_POINT ( 'NONE', #13603 ) ;
#4009=DIRECTION ( 'NONE',  ( -0.000000000000000000, 1.000000000000000000, -0.000000000000000000 ) ) ;
#4010=CARTESIAN_POINT ( 'NONE',  ( -15.97130229800533208, 29.67577800940753363, 93.41205153599007360 ) ) ;
#4014=CARTESIAN_POINT ( 'NONE',  ( -40.34137639590981195, 22.05937500034139731, 29.30972558990012189 ) ) ;
#4016=ADVANCED_FACE ( 'NONE', ( #4742, #2208 ), #16268, .T. ) ;
#4017=CARTESIAN_POINT ( 'NONE',  ( 49.86468353125001585, 28.82187500034139305, 16.20201782572375038 ) ) ;
#4019=CARTESIAN_POINT ( 'NONE',  ( 50.00000000000000000, 33.00000000000000000, -6.123233995736766085E-15 ) ) ;
#4020=CARTESIAN_POINT ( 'NONE',  ( -30.81806926056963292, 33.55937500034138310, -42.41743335407647209 ) ) ;
#4025=ORIENTED_EDGE ( 'NONE', *, *, #15235, .T. ) ;
#4031=CARTESIAN_POINT ( 'NONE',  ( -40.34137639590981905, 35.72187500034139163, -29.30972558990011478 ) ) ;
#4032=CARTESIAN_POINT ( 'NONE',  ( -49.86468353124999453, 39.75937500034139305, -16.20201782572375393 ) ) ;
#4035=CARTESIAN_POINT ( 'NONE',  ( 30.90169943749475578, 22.48125000068279533, 42.53254041760200010 ) ) ;
#4037=( BOUNDED_CURVE ( )  B_SPLINE_CURVE ( 2, ( #2176, #12248, #15909, #14814, #4533, #13572, #16160, #2099, #10923, #14899, #4871, #1015, #11006 ),
 .UNSPECIFIED., .F., .T. ) 
 B_SPLINE_CURVE_WITH_KNOTS ( ( 3, 2, 2, 2, 2, 2, 3 ),
 ( 0.4500000000000000111, 0.4533333333333333104, 0.4600000000000000200, 0.4666666666666666741, 0.4733333333333333282, 0.4799999999999999822, 0.4833333333333333370 ),
 .UNSPECIFIED. ) 
 CURVE ( )  GEOMETRIC_REPRESENTATION_ITEM ( )  RATIONAL_B_SPLINE_CURVE ( ( 0.9755282581475768211, 0.9755282581475770431, 1.000000000000000000, 0.9510565162951535312, 1.000000000000000000, 0.9510565162951535312, 1.000000000000000000, 0.9510565162951535312, 1.000000000000000000, 0.9510565162951535312, 1.000000000000000000, 0.9755282581475768211, 0.9755282581475768211 ) ) 
 REPRESENTATION_ITEM ( '' )  );
#4038=CARTESIAN_POINT ( 'NONE',  ( -40.34137639590981905, 25.72187500034139518, -29.30972558990011478 ) ) ;
#4048=CARTESIAN_POINT ( 'NONE',  ( 40.34137639590981195, 25.05937500034139376, -29.30972558990011834 ) ) ;
#4051=CARTESIAN_POINT ( 'NONE',  ( -40.34137639590981195, 44.12187500034139731, 29.30972558990012189 ) ) ;
#4059=DIRECTION ( 'NONE',  ( -0.000000000000000000, 1.000000000000000000, -0.000000000000000000 ) ) ;
#4061=ORIENTED_EDGE ( 'NONE', *, *, #16244, .T. ) ;
#4062=VERTEX_POINT ( 'NONE', #15176 ) ;
#4065=CARTESIAN_POINT ( 'NONE',  ( -3.219174618344376363E-15, 23.50000000000000000, -52.57311121191334990 ) ) ;
#4066=CARTESIAN_POINT ( 'NONE',  ( 30.81806926056964002, 48.55937500034138310, 42.41743335407647209 ) ) ;
#4068=CARTESIAN_POINT ( 'NONE',  ( 7.919222016226693306, 24.33250428222964246, 50.00000000000003553 ) ) ;
#4070=CARTESIAN_POINT ( 'NONE',  ( 49.86468353125000164, 24.92187500034139802, -6.106662507704105588E-15 ) ) ;
#4072=CARTESIAN_POINT ( 'NONE',  ( -3.219174618344376363E-15, 41.28125000068280315, -52.57311121191334990 ) ) ;
#4075=CARTESIAN_POINT ( 'NONE',  ( 50.00000000000000711, 20.68125000068279817, 16.24598481164530739 ) ) ;
#4083=CARTESIAN_POINT ( 'NONE',  ( 15.45084971874737789, 42.60000000000000142, 47.55282581475767500 ) ) ;
#4089=CARTESIAN_POINT ( 'NONE',  ( -2.317185599438165467E-15, 40.00000000000004974, 92.94692077166139654 ) ) ;
#4092=CARTESIAN_POINT ( 'NONE',  ( -30.90169943749474513, 29.48125000068279888, -42.53254041760200721 ) ) ;
#4093=CARTESIAN_POINT ( 'NONE',  ( 7.829870898593951800, 6.838588860456279228, 98.48475986922689174 ) ) ;
#4095=CARTESIAN_POINT ( 'NONE',  ( 49.86468353125000164, 30.92187500034139802, -6.106662507704105588E-15 ) ) ;
#4098=CARTESIAN_POINT ( 'NONE',  ( 30.90169943749475578, 28.70000000000000284, 42.53254041760200010 ) ) ;
#4099=CARTESIAN_POINT ( 'NONE',  ( 49.86468353125000164, 30.85937500034139802, -6.106662507704105588E-15 ) ) ;
#4106=ORIENTED_EDGE ( 'NONE', *, *, #3090, .F. ) ;
#4111=CARTESIAN_POINT ( 'NONE',  ( -30.90169943749473447, 38.29999999999999716, 42.53254041760200721 ) ) ;
#4115=CARTESIAN_POINT ( 'NONE',  ( 15.40903463028482356, 34.52187500034140299, 47.42413220539093999 ) ) ;
#4116=CARTESIAN_POINT ( 'NONE',  ( 15.40903463028481113, 43.25937500034139305, -47.42413220539094709 ) ) ;
#4119=CARTESIAN_POINT ( 'NONE',  ( 15.45084971874737789, 24.38125000068279746, 47.55282581475767500 ) ) ;
#4120=CARTESIAN_POINT ( 'NONE',  ( 17.50000000000001421, 23.63086963147864239, 94.22187259348842758 ) ) ;
#4121=STYLED_ITEM ( 'NONE', ( #1982 ), #8848 ) ;
#4122=CARTESIAN_POINT ( 'NONE',  ( 49.86468353125000164, 30.92187500034139802, -6.106662507704105588E-15 ) ) ;
#4123=CARTESIAN_POINT ( 'NONE',  ( -15.45084971874737256, 27.60000000000000142, -47.55282581475767500 ) ) ;
#4127=CARTESIAN_POINT ( 'NONE',  ( 30.90169943749475223, 48.48125000068279888, 42.53254041760199300 ) ) ;
#4131=CARTESIAN_POINT ( 'NONE',  ( 40.45084971874737079, 30.98125000068279888, -29.38926261462366440 ) ) ;
#4134=CARTESIAN_POINT ( 'NONE',  ( -40.34137639590981195, 22.05937500034139731, 29.30972558990012189 ) ) ;
#4138=CARTESIAN_POINT ( 'NONE',  ( -40.34137639590981195, 42.12187500034139731, 29.30972558990012189 ) ) ;
#4141=CARTESIAN_POINT ( 'NONE',  ( -30.81806926056963292, 49.62187500034139020, -42.41743335407647209 ) ) ;
#4143=VECTOR ( 'NONE', #8941, 1000.000000000000000 ) ;
#4145=ORIENTED_EDGE ( 'NONE', *, *, #8705, .T. ) ;
#4150=CARTESIAN_POINT ( 'NONE',  ( -2.445080149700054274E-14, 46.28125000068280315, 50.00000000000000000 ) ) ;
#4157=CARTESIAN_POINT ( 'NONE',  ( -30.90169943749473802, 26.29999999999999716, 42.53254041760200721 ) ) ;
#4158=CARTESIAN_POINT ( 'NONE',  ( -40.34137639590981195, 42.05937500034139731, 29.30972558990012189 ) ) ;
#4161=CARTESIAN_POINT ( 'NONE',  ( -49.99999999999999289, 31.68125000068279462, -16.24598481164531449 ) ) ;
#4167=CARTESIAN_POINT ( 'NONE',  ( 9.657523855033129090E-15, 42.28125000068278894, 52.57311121191334990 ) ) ;
#4169=CARTESIAN_POINT ( 'NONE',  ( 50.00000000000000711, 22.68125000068279817, 16.24598481164530739 ) ) ;
#4175=VERTEX_POINT ( 'NONE', #11692 ) ;
#4180=EDGE_CURVE ( 'NONE', #7762, #12541, #12086, .T. ) ;
#4183=CARTESIAN_POINT ( 'NONE',  ( -2.547328955960238000E-13, 22.49999999999999645, 49.99999999999999289 ) ) ;
#4188=CARTESIAN_POINT ( 'NONE',  ( 11.63664291089594371, 9.379540242982125520, 97.65878401859123414 ) ) ;
#4189=CARTESIAN_POINT ( 'NONE',  ( -46.56218328577778465, 20.00000000000000355, 17.84593874833660720 ) ) ;
#4190=CARTESIAN_POINT ( 'NONE',  ( -40.34137639590981905, 29.72187500034139518, -29.30972558990011478 ) ) ;
#4193=CARTESIAN_POINT ( 'NONE',  ( -40.45084971874737079, 22.19999999999999929, 29.38926261462367151 ) ) ;
#4195=CARTESIAN_POINT ( 'NONE',  ( 30.81806926056962936, 33.15937500034139873, -42.41743335407647209 ) ) ;
#4204=CARTESIAN_POINT ( 'NONE',  ( -7.919222016226870942, 38.44874571845316069, 49.99999999999997158 ) ) ;
#4207=CARTESIAN_POINT ( 'NONE',  ( 30.81806926056962936, 37.22187500034139873, -42.41743335407647209 ) ) ;
#4208=CARTESIAN_POINT ( 'NONE',  ( 9.631387414534489405E-15, 34.35937500034140157, 52.43083105670540789 ) ) ;
#4211=CARTESIAN_POINT ( 'NONE',  ( 40.34137639590981905, 48.65937500034139873, 29.30972558990010768 ) ) ;
#4213=CARTESIAN_POINT ( 'NONE',  ( 30.81806926056962936, 25.22187500034139873, -42.41743335407647209 ) ) ;
#4214=CARTESIAN_POINT ( 'NONE',  ( -30.90169943749474513, 27.48125000068279888, -42.53254041760200721 ) ) ;
#4218=ORIENTED_EDGE ( 'NONE', *, *, #2226, .F. ) ;
#4219=CARTESIAN_POINT ( 'NONE',  ( 50.00000000000000000, 48.78125000068279604, -6.123233995736766085E-15 ) ) ;
#4223=CARTESIAN_POINT ( 'NONE',  ( 15.40903463028481113, 25.25937500034139660, -47.42413220539094709 ) ) ;
#4225=CARTESIAN_POINT ( 'NONE',  ( -49.86468353124999453, 42.02187500034139589, 16.20201782572377169 ) ) ;
#4229=CARTESIAN_POINT ( 'NONE',  ( -30.81806926056963292, 47.62187500034139731, -42.41743335407647209 ) ) ;
#4240=DIRECTION ( 'NONE',  ( -0.000000000000000000, 1.000000000000000000, -0.000000000000000000 ) ) ;
#4241=CARTESIAN_POINT ( 'NONE',  ( 30.90169943749475578, 26.70000000000000284, 42.53254041760200010 ) ) ;
#4243=CARTESIAN_POINT ( 'NONE',  ( 9.631387414534489405E-15, 46.35937500034139447, 52.43083105670540789 ) ) ;
#4249=CARTESIAN_POINT ( 'NONE',  ( -49.99999999999999289, 33.68125000068278752, -16.24598481164531449 ) ) ;
#4251=CARTESIAN_POINT ( 'NONE',  ( 40.45084971874737079, 20.98125000068279888, -29.38926261462366440 ) ) ;
#4255=VECTOR ( 'NONE', #2903, 1000.000000000000000 ) ;
#4257=ORIENTED_EDGE ( 'NONE', *, *, #2451, .F. ) ;
#4259=DIRECTION ( 'NONE',  ( 0.000000000000000000, 1.000000000000000000, 0.000000000000000000 ) ) ;
#4266=CARTESIAN_POINT ( 'NONE',  ( -49.99999999999999289, 37.68125000068279462, -16.24598481164531449 ) ) ;
#4268=CARTESIAN_POINT ( 'NONE',  ( 10.76154604949448768, 8.652744724135910559, 97.88922921878788941 ) ) ;
#4270=CARTESIAN_POINT ( 'NONE',  ( 9.631387414534489405E-15, 28.42187500034139447, 52.43083105670540789 ) ) ;
#4271=CARTESIAN_POINT ( 'NONE',  ( -7.919222016226688865, 21.55125428154684641, -50.00000000000003553 ) ) ;
#4273=CARTESIAN_POINT ( 'NONE',  ( 40.34137639590981905, 30.65937500034139518, 29.30972558990010768 ) ) ;
#4282=CARTESIAN_POINT ( 'NONE',  ( -30.90169943749474513, 37.70000000000000284, -42.53254041760200721 ) ) ;
#4285=CARTESIAN_POINT ( 'NONE',  ( 15.40903463028482356, 38.52187500034139589, 47.42413220539093999 ) ) ;
#4286=CARTESIAN_POINT ( 'NONE',  ( 30.81806926056964002, 38.55937500034139731, 42.41743335407646498 ) ) ;
#4288=( BOUNDED_SURFACE ( )  B_SPLINE_SURFACE ( 1, 2, ( 
 ( #15046, #12403, #7251, #15125, #10149, #8562, #8732, #16297, #4934, #8646, #2333, #6007, #6247, #13797, #16385, #2410, #2491, #7488, #12308, #11241, #910, #2160, #6168, #5096, #12558, #8811, #11075, #1076, #7414, #14962, #13716, #3750, #5019, #12484, #995, #16143, #11319, #1153, #13554, #7568, #9990, #9908, #6096, #4851, #10072, #13875, #12644, #3588, #1241, #11399, #4771, #3831, #15841, #15201, #16219, #9829, #14879, #3508, #13632, #2242, #11163, #12725, #7978, #14119, #6412, #1403, #1653, #3915, #1577, #13052, #15535, #6670, #1321, #5345, #11719, #4167, #318, #14289, #157, #9236, #15454, #7655, #15289, #5418, #11473, #4072, #2735, #2659, #5175, #10317, #7897, #6752, #2579, #2910, #11797, #12972, #10475, #12884, #396, #70, #5505, #10569, #1496, #10231, #15624, #8896, #13958, #8984, #14042, #11645, #7733, #12800, #6494, #11550, #5266, #15373, #3995, #9068, #7813, #6588, #239, #10397, #9144, #14202, #2827, #10645, #1034, #16006, #13127, #11026, #5583, #14367, #8447, #1734, #12441, #3545, #7292, #8522, #13591, #16094, #14915, #4729, #15698, #4325, #2285, #3380, #2196, #10941, #14747, #6131, #7377, #9393, #2986, #8598, #4632, #14440, #12349, #13510, #1816, #4811, #8145, #4249, #13212, #2116, #9696, #3064, #8055, #7205, #6833, #9788, #16181, #6908, #5879, #11883, #11962, #11121, #483, #12266, #789, #868, #5963, #14834, #3463, #950, #6049, #9862, #13673, #11201, #9314, #1111, #8857, #7527, #11362, #5063, #15247, #1194, #1286, #10115, #6458, #1366, #6293, #16429, #15088, #6540, #12689, #15165, #9944, #13916, #14999, #12846, #10036, #3794, #3715, #8945, #15335, #11516, #2534, #14003, #7454, #8773, #5221, #16253, #4976, #13836, #12520, #2622, #6377, #4888, #10280, #7615, #12599, #2449, #11441, #5139, #7697, #3954, #34, #10195, #3873, #6207, #3635, #113, #12768, #9028, #14083, #2699, #7775, #1449, #8691, #13758, #2370, #11278, #16337, #9106, #4119, #4368, #6630, #4290, #10684, #1782, #9353, #15417, #8016, #14404, #6875, #3026, #526, #2872, #11926, #1696, #10355, #1540, #8097, #4035, #6793, #5461, #5383, #7856, #13013, #10611, #15739, #5306, #5623, #9433, #15668, #13175, #14484, #3116, #8189, #12935, #11681, #13254, #14332, #1854, #11603, #10527, #201, #10439, #14165, #11841, #14252 ),
 ( #2781, #279, #15495, #1616, #448, #9191, #7939, #13091, #6708, #11760, #359, #15586, #4211, #5549, #2949, #9278, #2021, #12172, #15826, #16072, #7190, #9770, #2102, #12332, #13494, #601, #4615, #5695, #12005, #15989, #14902, #854, #2179, #10763, #10926, #772, #8344, #7115, #13575, #14817, #5862, #687, #4457, #9522, #3529, #6032, #3448, #11009, #4708, #12251, #933, #5948, #13330, #8266, #4794, #9678, #8510, #13405, #14728, #8582, #9850, #1934, #14569, #11105, #3360, #7025, #7276, #8431, #4536, #16164, #10848, #6950, #15912, #13656, #3193, #12080, #5781, #9599, #14646, #3275, #13985, #3613, #3701, #11185, #13743, #8919, #16240, #16412, #4874, #10018, #3775, #1097, #8677, #7439, #8758, #6190, #6115, #12505, #3937, #2356, #11346, #15072, #13820, #7509, #1268, #2432, #8834, #12581, #2603, #3854, #1178, #6273, #11265, #9010, #15149, #5045, #12427, #10098, #1020, #15317, #16322, #13898, #4957, #11424, #1346, #7679, #2513, #17, #9931, #7592, #12749, #2265, #12671, #6360, #14984, #5121, #6437, #10174, #11498, #95, #15224, #5198, #10254, #7363, #3010, #15721, #14389, #344, #6519, #1761, #11666, #5605, #510, #15649, #9089, #5288, #14146, #7756, #5367, #7920, #6863, #15477, #10423, #4020, #10670, #9170, #11578, #4195, #15401, #12826, #1599, #2853, #184, #6778, #14315, #428, #9259, #8081, #2934, #1429, #11741, #10339, #2682, #6693, #4352, #8001, #9339, #2762, #5443, #12996, #4099, #14228, #4273, #5532, #10506, #7838, #12912, #11821, #13075, #14066, #13153, #15565, #1678, #6611, #10593, #11910, #1522, #262, #666, #15973, #14630, #583, #16146, #9752, #12154, #12064, #13557, #7174, #913, #838, #4594, #5929, #13240, #8492, #3255, #6934, #1913, #2163, #4435, #2085, #7255, #16053, #12235, #1838, #5846, #10988, #4683, #14797, #3431, #5763, #12312, #9658, #8172, #15805, #6010, #11986, #14708, #8325, #3178, #5677, #10832, #8411, #11079, #3096, #9417, #14462, #13479, #10747, #9506, #14551, #8249, #13314, #7008, #15896, #755, #4520, #9585, #13390, #1998, #7095, #10909, #3339, #7418, #12407, #16300, #9992, #9833, #1157, #13962, #11403, #15050, #3512, #14882, #2494, #8814, #11244, #10075, #8650, #8565, #6251, #3592, #13635, #6339, #1325, #16222, #16389, #7491, #12561, #4938, #2337, #5099 ) ),
 .UNSPECIFIED., .F., .F., .F. ) 
 B_SPLINE_SURFACE_WITH_KNOTS ( ( 2, 2 ),
 ( 3, 2, 2, 2, 2, 2, 2, 2, 2, 2, 2, 2, 2, 2, 2, 2, 2, 2, 2, 2, 2, 2, 2, 2, 2, 2, 2, 2, 2, 2, 2, 2, 2, 2, 2, 2, 2, 2, 2, 2, 2, 2, 2, 2, 2, 2, 2, 2, 2, 2, 2, 2, 2, 2, 2, 2, 2, 2, 2, 2, 2, 2, 2, 2, 2, 2, 2, 2, 2, 2, 2, 2, 2, 2, 2, 2, 2, 2, 2, 2, 2, 2, 2, 2, 2, 2, 2, 2, 2, 2, 2, 2, 2, 2, 2, 2, 2, 2, 2, 2, 2, 2, 2, 2, 2, 2, 2, 2, 2, 2, 2, 2, 2, 2, 2, 2, 2, 2, 2, 2, 2, 2, 2, 2, 2, 2, 2, 2, 2, 2, 2, 2, 2, 2, 2, 2, 2, 2, 2, 2, 2, 2, 2, 2, 2, 2, 2, 2, 2, 2, 3 ),
 ( 0.000000000000000000, 1.000000000000000000 ),
 ( 0.000000000000000000, 0.006666666666666667095, 0.01333333333333333419, 0.02000000000000000042, 0.02666666666666666838, 0.03333333333333333287, 0.04000000000000000083, 0.04666666666666666879, 0.05333333333333333676, 0.05999999999999999778, 0.06666666666666666574, 0.07333333333333333370, 0.08000000000000000167, 0.08666666666666666963, 0.09333333333333333759, 0.1000000000000000056, 0.1066666666666666735, 0.1133333333333333276, 0.1199999999999999956, 0.1266666666666666774, 0.1333333333333333315, 0.1400000000000000133, 0.1466666666666666674, 0.1533333333333333215, 0.1600000000000000033, 0.1666666666666666574, 0.1733333333333333393, 0.1799999999999999933, 0.1866666666666666752, 0.1933333333333333293, 0.2000000000000000111, 0.2066666666666666652, 0.2133333333333333470, 0.2200000000000000011, 0.2266666666666666552, 0.2333333333333333370, 0.2399999999999999911, 0.2466666666666666730, 0.2533333333333333548, 0.2600000000000000089, 0.2666666666666666630, 0.2733333333333333171, 0.2800000000000000266, 0.2866666666666666807, 0.2933333333333333348, 0.2999999999999999889, 0.3066666666666666430, 0.3133333333333333526, 0.3200000000000000067, 0.3266666666666666607, 0.3333333333333333148, 0.3400000000000000244, 0.3466666666666666785, 0.3533333333333333326, 0.3599999999999999867, 0.3666666666666666408, 0.3733333333333333504, 0.3800000000000000044, 0.3866666666666666585, 0.3933333333333333126, 0.4000000000000000222, 0.4066666666666666763, 0.4133333333333333304, 0.4199999999999999845, 0.4266666666666666941, 0.4333333333333333481, 0.4400000000000000022, 0.4466666666666666563, 0.4533333333333333104, 0.4600000000000000200, 0.4666666666666666741, 0.4733333333333333282, 0.4799999999999999822, 0.4866666666666666918, 0.4933333333333333459, 0.5000000000000000000, 0.5066666666666667096, 0.5133333333333333082, 0.5200000000000000178, 0.5266666666666666163, 0.5333333333333333259, 0.5400000000000000355, 0.5466666666666666341, 0.5533333333333333437, 0.5600000000000000533, 0.5666666666666666519, 0.5733333333333333615, 0.5799999999999999600, 0.5866666666666666696, 0.5933333333333333792, 0.5999999999999999778, 0.6066666666666666874, 0.6133333333333332860, 0.6199999999999999956, 0.6266666666666667052, 0.6333333333333333037, 0.6400000000000000133, 0.6466666666666666119, 0.6533333333333333215, 0.6600000000000000311, 0.6666666666666666297, 0.6733333333333333393, 0.6800000000000000488, 0.6866666666666666474, 0.6933333333333333570, 0.6999999999999999556, 0.7066666666666666652, 0.7133333333333333748, 0.7199999999999999734, 0.7266666666666666829, 0.7333333333333332815, 0.7399999999999999911, 0.7466666666666667007, 0.7533333333333332993, 0.7600000000000000089, 0.7666666666666667185, 0.7733333333333333171, 0.7800000000000000266, 0.7866666666666666252, 0.7933333333333333348, 0.8000000000000000444, 0.8066666666666666430, 0.8133333333333333526, 0.8199999999999999512, 0.8266666666666666607, 0.8333333333333333703, 0.8399999999999999689, 0.8466666666666666785, 0.8533333333333333881, 0.8599999999999999867, 0.8666666666666666963, 0.8733333333333332948, 0.8800000000000000044, 0.8866666666666667140, 0.8933333333333333126, 0.9000000000000000222, 0.9066666666666666208, 0.9133333333333333304, 0.9200000000000000400, 0.9266666666666666385, 0.9333333333333333481, 0.9399999999999999467, 0.9466666666666666563, 0.9533333333333333659, 0.9599999999999999645, 0.9666666666666666741, 0.9733333333333333837, 0.9799999999999999822, 0.9866666666666666918, 0.9933333333333332904, 1.000000000000000000 ),
 .UNSPECIFIED. ) 
 GEOMETRIC_REPRESENTATION_ITEM ( )  RATIONAL_B_SPLINE_SURFACE ( (
 ( 1.000000000000000000, 0.9510565162951535312, 1.000000000000000000, 0.9510565162951535312, 1.000000000000000000, 0.9510565162951535312, 1.000000000000000000, 0.9510565162951535312, 1.000000000000000000, 0.9510565162951535312, 1.000000000000000000, 0.9510565162951535312, 1.000000000000000000, 0.9510565162951535312, 1.000000000000000000, 0.9510565162951535312, 1.000000000000000000, 0.9510565162951535312, 1.000000000000000000, 0.9510565162951535312, 1.000000000000000000, 0.9510565162951535312, 1.000000000000000000, 0.9510565162951535312, 1.000000000000000000, 0.9510565162951535312, 1.000000000000000000, 0.9510565162951535312, 1.000000000000000000, 0.9510565162951535312, 1.000000000000000000, 0.9510565162951535312, 1.000000000000000000, 0.9510565162951535312, 1.000000000000000000, 0.9510565162951535312, 1.000000000000000000, 0.9510565162951535312, 1.000000000000000000, 0.9510565162951535312, 1.000000000000000000, 0.9510565162951535312, 1.000000000000000000, 0.9510565162951535312, 1.000000000000000000, 0.9510565162951535312, 1.000000000000000000, 0.9510565162951535312, 1.000000000000000000, 0.9510565162951535312, 1.000000000000000000, 0.9510565162951535312, 1.000000000000000000, 0.9510565162951535312, 1.000000000000000000, 0.9510565162951535312, 1.000000000000000000, 0.9510565162951535312, 1.000000000000000000, 0.9510565162951535312, 1.000000000000000000, 0.9510565162951535312, 1.000000000000000000, 0.9510565162951535312, 1.000000000000000000, 0.9510565162951535312, 1.000000000000000000, 0.9510565162951535312, 1.000000000000000000, 0.9510565162951535312, 1.000000000000000000, 0.9510565162951535312, 1.000000000000000000, 0.9510565162951535312, 1.000000000000000000, 0.9510565162951535312, 1.000000000000000000, 0.9510565162951535312, 1.000000000000000000, 0.9510565162951535312, 1.000000000000000000, 0.9510565162951535312, 1.000000000000000000, 0.9510565162951535312, 1.000000000000000000, 0.9510565162951535312, 1.000000000000000000, 0.9510565162951535312, 1.000000000000000000, 0.9510565162951535312, 1.000000000000000000, 0.9510565162951535312, 1.000000000000000000, 0.9510565162951535312, 1.000000000000000000, 0.9510565162951535312, 1.000000000000000000, 0.9510565162951535312, 1.000000000000000000, 0.9510565162951535312, 1.000000000000000000, 0.9510565162951535312, 1.000000000000000000, 0.9510565162951535312, 1.000000000000000000, 0.9510565162951535312, 1.000000000000000000, 0.9510565162951535312, 1.000000000000000000, 0.9510565162951535312, 1.000000000000000000, 0.9510565162951535312, 1.000000000000000000, 0.9510565162951535312, 1.000000000000000000, 0.9510565162951535312, 1.000000000000000000, 0.9510565162951535312, 1.000000000000000000, 0.9510565162951535312, 1.000000000000000000, 0.9510565162951535312, 1.000000000000000000, 0.9510565162951535312, 1.000000000000000000, 0.9510565162951535312, 1.000000000000000000, 0.9510565162951535312, 1.000000000000000000, 0.9510565162951535312, 1.000000000000000000, 0.9510565162951535312, 1.000000000000000000, 0.9510565162951535312, 1.000000000000000000, 0.9510565162951535312, 1.000000000000000000, 0.9510565162951535312, 1.000000000000000000, 0.9510565162951535312, 1.000000000000000000, 0.9510565162951535312, 1.000000000000000000, 0.9510565162951535312, 1.000000000000000000, 0.9510565162951535312, 1.000000000000000000, 0.9510565162951535312, 1.000000000000000000, 0.9510565162951535312, 1.000000000000000000, 0.9510565162951535312, 1.000000000000000000, 0.9510565162951535312, 1.000000000000000000, 0.9510565162951535312, 1.000000000000000000, 0.9510565162951535312, 1.000000000000000000, 0.9510565162951535312, 1.000000000000000000, 0.9510565162951535312, 1.000000000000000000, 0.9510565162951535312, 1.000000000000000000, 0.9510565162951535312, 1.000000000000000000, 0.9510565162951535312, 1.000000000000000000, 0.9510565162951535312, 1.000000000000000000, 0.9510565162951535312, 1.000000000000000000, 0.9510565162951535312, 1.000000000000000000, 0.9510565162951535312, 1.000000000000000000, 0.9510565162951535312, 1.000000000000000000, 0.9510565162951535312, 1.000000000000000000, 0.9510565162951535312, 1.000000000000000000, 0.9510565162951535312, 1.000000000000000000, 0.9510565162951535312, 1.000000000000000000, 0.9510565162951535312, 1.000000000000000000, 0.9510565162951535312, 1.000000000000000000, 0.9510565162951535312, 1.000000000000000000, 0.9510565162951535312, 1.000000000000000000, 0.9510565162951535312, 1.000000000000000000, 0.9510565162951535312, 1.000000000000000000, 0.9510565162951535312, 1.000000000000000000, 0.9510565162951535312, 1.000000000000000000, 0.9510565162951535312, 1.000000000000000000, 0.9510565162951535312, 1.000000000000000000, 0.9510565162951535312, 1.000000000000000000, 0.9510565162951535312, 1.000000000000000000, 0.9510565162951535312, 1.000000000000000000, 0.9510565162951535312, 1.000000000000000000, 0.9510565162951535312, 1.000000000000000000, 0.9510565162951535312, 1.000000000000000000, 0.9510565162951535312, 1.000000000000000000, 0.9510565162951535312, 1.000000000000000000, 0.9510565162951535312, 1.000000000000000000, 0.9510565162951535312, 1.000000000000000000, 0.9510565162951535312, 1.000000000000000000, 0.9510565162951535312, 1.000000000000000000, 0.9510565162951535312, 1.000000000000000000, 0.9510565162951535312, 1.000000000000000000, 0.9510565162951535312, 1.000000000000000000, 0.9510565162951535312, 1.000000000000000000, 0.9510565162951535312, 1.000000000000000000, 0.9510565162951535312, 1.000000000000000000, 0.9510565162951535312, 1.000000000000000000, 0.9510565162951535312, 1.000000000000000000, 0.9510565162951535312, 1.000000000000000000, 0.9510565162951535312, 1.000000000000000000, 0.9510565162951535312, 1.000000000000000000, 0.9510565162951535312, 1.000000000000000000, 0.9510565162951535312, 1.000000000000000000, 0.9510565162951535312, 1.000000000000000000, 0.9510565162951535312, 1.000000000000000000, 0.9510565162951535312, 1.000000000000000000, 0.9510565162951535312, 1.000000000000000000, 0.9510565162951535312, 1.000000000000000000, 0.9510565162951535312, 1.000000000000000000, 0.9510565162951535312, 1.000000000000000000, 0.9510565162951535312, 1.000000000000000000, 0.9510565162951535312, 1.000000000000000000, 0.9510565162951535312, 1.000000000000000000, 0.9510565162951535312, 1.000000000000000000, 0.9510565162951535312, 1.000000000000000000, 0.9510565162951535312, 1.000000000000000000, 0.9510565162951535312, 1.000000000000000000, 0.9510565162951535312, 1.000000000000000000, 0.9510565162951535312, 1.000000000000000000, 0.9510565162951535312, 1.000000000000000000, 0.9510565162951535312, 1.000000000000000000, 0.9510565162951535312, 1.000000000000000000, 0.9510565162951535312, 1.000000000000000000, 0.9510565162951535312, 1.000000000000000000, 0.9510565162951535312, 1.000000000000000000),
 ( 1.000000000000000000, 0.9510565162951535312, 1.000000000000000000, 0.9510565162951535312, 1.000000000000000000, 0.9510565162951535312, 1.000000000000000000, 0.9510565162951535312, 1.000000000000000000, 0.9510565162951535312, 1.000000000000000000, 0.9510565162951535312, 1.000000000000000000, 0.9510565162951535312, 1.000000000000000000, 0.9510565162951535312, 1.000000000000000000, 0.9510565162951535312, 1.000000000000000000, 0.9510565162951535312, 1.000000000000000000, 0.9510565162951535312, 1.000000000000000000, 0.9510565162951535312, 1.000000000000000000, 0.9510565162951535312, 1.000000000000000000, 0.9510565162951535312, 1.000000000000000000, 0.9510565162951535312, 1.000000000000000000, 0.9510565162951535312, 1.000000000000000000, 0.9510565162951535312, 1.000000000000000000, 0.9510565162951535312, 1.000000000000000000, 0.9510565162951535312, 1.000000000000000000, 0.9510565162951535312, 1.000000000000000000, 0.9510565162951535312, 1.000000000000000000, 0.9510565162951535312, 1.000000000000000000, 0.9510565162951535312, 1.000000000000000000, 0.9510565162951535312, 1.000000000000000000, 0.9510565162951535312, 1.000000000000000000, 0.9510565162951535312, 1.000000000000000000, 0.9510565162951535312, 1.000000000000000000, 0.9510565162951535312, 1.000000000000000000, 0.9510565162951535312, 1.000000000000000000, 0.9510565162951535312, 1.000000000000000000, 0.9510565162951535312, 1.000000000000000000, 0.9510565162951535312, 1.000000000000000000, 0.9510565162951535312, 1.000000000000000000, 0.9510565162951535312, 1.000000000000000000, 0.9510565162951535312, 1.000000000000000000, 0.9510565162951535312, 1.000000000000000000, 0.9510565162951535312, 1.000000000000000000, 0.9510565162951535312, 1.000000000000000000, 0.9510565162951535312, 1.000000000000000000, 0.9510565162951535312, 1.000000000000000000, 0.9510565162951535312, 1.000000000000000000, 0.9510565162951535312, 1.000000000000000000, 0.9510565162951535312, 1.000000000000000000, 0.9510565162951535312, 1.000000000000000000, 0.9510565162951535312, 1.000000000000000000, 0.9510565162951535312, 1.000000000000000000, 0.9510565162951535312, 1.000000000000000000, 0.9510565162951535312, 1.000000000000000000, 0.9510565162951535312, 1.000000000000000000, 0.9510565162951535312, 1.000000000000000000, 0.9510565162951535312, 1.000000000000000000, 0.9510565162951535312, 1.000000000000000000, 0.9510565162951535312, 1.000000000000000000, 0.9510565162951535312, 1.000000000000000000, 0.9510565162951535312, 1.000000000000000000, 0.9510565162951535312, 1.000000000000000000, 0.9510565162951535312, 1.000000000000000000, 0.9510565162951535312, 1.000000000000000000, 0.9510565162951535312, 1.000000000000000000, 0.9510565162951535312, 1.000000000000000000, 0.9510565162951535312, 1.000000000000000000, 0.9510565162951535312, 1.000000000000000000, 0.9510565162951535312, 1.000000000000000000, 0.9510565162951535312, 1.000000000000000000, 0.9510565162951535312, 1.000000000000000000, 0.9510565162951535312, 1.000000000000000000, 0.9510565162951535312, 1.000000000000000000, 0.9510565162951535312, 1.000000000000000000, 0.9510565162951535312, 1.000000000000000000, 0.9510565162951535312, 1.000000000000000000, 0.9510565162951535312, 1.000000000000000000, 0.9510565162951535312, 1.000000000000000000, 0.9510565162951535312, 1.000000000000000000, 0.9510565162951535312, 1.000000000000000000, 0.9510565162951535312, 1.000000000000000000, 0.9510565162951535312, 1.000000000000000000, 0.9510565162951535312, 1.000000000000000000, 0.9510565162951535312, 1.000000000000000000, 0.9510565162951535312, 1.000000000000000000, 0.9510565162951535312, 1.000000000000000000, 0.9510565162951535312, 1.000000000000000000, 0.9510565162951535312, 1.000000000000000000, 0.9510565162951535312, 1.000000000000000000, 0.9510565162951535312, 1.000000000000000000, 0.9510565162951535312, 1.000000000000000000, 0.9510565162951535312, 1.000000000000000000, 0.9510565162951535312, 1.000000000000000000, 0.9510565162951535312, 1.000000000000000000, 0.9510565162951535312, 1.000000000000000000, 0.9510565162951535312, 1.000000000000000000, 0.9510565162951535312, 1.000000000000000000, 0.9510565162951535312, 1.000000000000000000, 0.9510565162951535312, 1.000000000000000000, 0.9510565162951535312, 1.000000000000000000, 0.9510565162951535312, 1.000000000000000000, 0.9510565162951535312, 1.000000000000000000, 0.9510565162951535312, 1.000000000000000000, 0.9510565162951535312, 1.000000000000000000, 0.9510565162951535312, 1.000000000000000000, 0.9510565162951535312, 1.000000000000000000, 0.9510565162951535312, 1.000000000000000000, 0.9510565162951535312, 1.000000000000000000, 0.9510565162951535312, 1.000000000000000000, 0.9510565162951535312, 1.000000000000000000, 0.9510565162951535312, 1.000000000000000000, 0.9510565162951535312, 1.000000000000000000, 0.9510565162951535312, 1.000000000000000000, 0.9510565162951535312, 1.000000000000000000, 0.9510565162951535312, 1.000000000000000000, 0.9510565162951535312, 1.000000000000000000, 0.9510565162951535312, 1.000000000000000000, 0.9510565162951535312, 1.000000000000000000, 0.9510565162951535312, 1.000000000000000000, 0.9510565162951535312, 1.000000000000000000, 0.9510565162951535312, 1.000000000000000000, 0.9510565162951535312, 1.000000000000000000, 0.9510565162951535312, 1.000000000000000000, 0.9510565162951535312, 1.000000000000000000, 0.9510565162951535312, 1.000000000000000000, 0.9510565162951535312, 1.000000000000000000, 0.9510565162951535312, 1.000000000000000000, 0.9510565162951535312, 1.000000000000000000, 0.9510565162951535312, 1.000000000000000000, 0.9510565162951535312, 1.000000000000000000, 0.9510565162951535312, 1.000000000000000000, 0.9510565162951535312, 1.000000000000000000, 0.9510565162951535312, 1.000000000000000000, 0.9510565162951535312, 1.000000000000000000, 0.9510565162951535312, 1.000000000000000000, 0.9510565162951535312, 1.000000000000000000, 0.9510565162951535312, 1.000000000000000000, 0.9510565162951535312, 1.000000000000000000, 0.9510565162951535312, 1.000000000000000000, 0.9510565162951535312, 1.000000000000000000, 0.9510565162951535312, 1.000000000000000000, 0.9510565162951535312, 1.000000000000000000, 0.9510565162951535312, 1.000000000000000000, 0.9510565162951535312, 1.000000000000000000, 0.9510565162951535312, 1.000000000000000000, 0.9510565162951535312, 1.000000000000000000, 0.9510565162951535312, 1.000000000000000000, 0.9510565162951535312, 1.000000000000000000, 0.9510565162951535312, 1.000000000000000000, 0.9510565162951535312, 1.000000000000000000, 0.9510565162951535312, 1.000000000000000000, 0.9510565162951535312, 1.000000000000000000, 0.9510565162951535312, 1.000000000000000000, 0.9510565162951535312, 1.000000000000000000, 0.9510565162951535312, 1.000000000000000000, 0.9510565162951535312, 1.000000000000000000) ) ) 
 REPRESENTATION_ITEM ( '' )  SURFACE ( )  );
#4290=CARTESIAN_POINT ( 'NONE',  ( -30.90169943749473802, 24.08125000068279675, 42.53254041760200721 ) ) ;
#4293=CARTESIAN_POINT ( 'NONE',  ( 30.81806926056964002, 26.62187500034139731, 42.41743335407647209 ) ) ;
#4297=EDGE_CURVE ( 'NONE', #6400, #12892, #11556, .T. ) ;
#4302=CARTESIAN_POINT ( 'NONE',  ( -7.919222016226934890, 34.22999571913595673, 49.99999999999996447 ) ) ;
#4304=CARTESIAN_POINT ( 'NONE',  ( 49.86468353125000164, 24.85937500034139802, -6.106662507704105588E-15 ) ) ;
#4305=CARTESIAN_POINT ( 'NONE',  ( -1.240322475938754499E-13, 36.28125000068280315, 50.00000000000000000 ) ) ;
#4306=CARTESIAN_POINT ( 'NONE',  ( -30.81806926056963292, 41.62187500034139020, -42.41743335407646498 ) ) ;
#4308=CARTESIAN_POINT ( 'NONE',  ( 9.631387414534489405E-15, 46.42187500034139447, 52.43083105670540789 ) ) ;
#4314=EDGE_CURVE ( 'NONE', #7369, #13993, #13783, .T. ) ;
#4316=CARTESIAN_POINT ( 'NONE',  ( 50.00000000000000711, 38.68125000068280173, 16.24598481164530739 ) ) ;
#4319=CARTESIAN_POINT ( 'NONE',  ( 15.45084971874736723, 27.40000000000000213, -47.55282581475768211 ) ) ;
#4320=CARTESIAN_POINT ( 'NONE',  ( -49.86468353124999453, 41.95937500034138878, 16.20201782572377525 ) ) ;
#4321=CARTESIAN_POINT ( 'NONE',  ( -7.919222016226804328, 26.22999571913594963, 50.00000000000000000 ) ) ;
#4325=CARTESIAN_POINT ( 'NONE',  ( -30.90169943749474868, 35.48125000068279888, -42.53254041760200721 ) ) ;
#4334=EDGE_CURVE ( 'NONE', #10001, #12012, #3708, .T. ) ;
#4342=CARTESIAN_POINT ( 'NONE',  ( 49.99999999999999289, 23.10000000000000142, -16.24598481164532160 ) ) ;
#4346=CARTESIAN_POINT ( 'NONE',  ( -50.00000000000000000, 37.78125000068280315, 0.000000000000000000 ) ) ;
#4347=FACE_OUTER_BOUND ( 'NONE', #4834, .T. ) ;
#4349=CARTESIAN_POINT ( 'NONE',  ( 49.86468353125000164, 20.92187500034139802, -6.106662507704105588E-15 ) ) ;
#4352=CARTESIAN_POINT ( 'NONE',  ( -15.40903463028481646, 31.45937500034139944, -47.42413220539093999 ) ) ;
#4354=CARTESIAN_POINT ( 'NONE',  ( 1.293669679204937499E-13, 39.50000000000000711, -50.00000000000000000 ) ) ;
#4363=CARTESIAN_POINT ( 'NONE',  ( -3.210462471511496205E-15, 35.42187500034140157, -52.43083105670540789 ) ) ;
#4364=CARTESIAN_POINT ( 'NONE',  ( -40.34137639590981195, 36.05937500034139731, 29.30972558990012189 ) ) ;
#4365=CARTESIAN_POINT ( 'NONE',  ( -30.90169943749473447, 44.30000000000000426, 42.53254041760200721 ) ) ;
#4368=CARTESIAN_POINT ( 'NONE',  ( 9.657523855033129090E-15, 24.28125000068279959, 52.57311121191334990 ) ) ;
#4370=CARTESIAN_POINT ( 'NONE',  ( 30.81806926056964002, 24.62187500034139731, 42.41743335407647209 ) ) ;
#4371=CIRCLE ( 'NONE', #3574, 100.0000000000000000 ) ;
#4377=( BOUNDED_CURVE ( )  B_SPLINE_CURVE ( 2, ( #1150, #11313, #5580, #152, #5341, #9139, #12880, #4161, #1729, #7809, #11879, #9386, #9231 ),
 .UNSPECIFIED., .F., .T. ) 
 B_SPLINE_CURVE_WITH_KNOTS ( ( 3, 2, 2, 2, 2, 2, 3 ),
 ( 0.5833333333333333703, 0.5866666666666666696, 0.5933333333333333792, 0.5999999999999999778, 0.6066666666666666874, 0.6133333333333332860, 0.6166666666666666963 ),
 .UNSPECIFIED. ) 
 CURVE ( )  GEOMETRIC_REPRESENTATION_ITEM ( )  RATIONAL_B_SPLINE_CURVE ( ( 0.9755282581475768211, 0.9755282581475771542, 1.000000000000000000, 0.9510565162951535312, 1.000000000000000000, 0.9510565162951535312, 1.000000000000000000, 0.9510565162951535312, 1.000000000000000000, 0.9510565162951535312, 1.000000000000000000, 0.9755282581475763770, 0.9755282581475768211 ) ) 
 REPRESENTATION_ITEM ( '' )  );
#4381=CARTESIAN_POINT ( 'NONE',  ( -49.86468353124999453, 23.95937500034138878, 16.20201782572377525 ) ) ;
#4385=CARTESIAN_POINT ( 'NONE',  ( 40.45084971874737789, 38.80000000000000426, 29.38926261462365375 ) ) ;
#4388=CARTESIAN_POINT ( 'NONE',  ( 30.81806926056962936, 49.22187500034139873, -42.41743335407647209 ) ) ;
#4391=ADVANCED_FACE ( 'NONE', ( #2366 ), #9608, .F. ) ;
#4396=CYLINDRICAL_SURFACE ( 'NONE', #10509, 50.00000000000000000 ) ;
#4398=CARTESIAN_POINT ( 'NONE',  ( 40.45084971874737079, 21.19999999999999929, -29.38926261462366440 ) ) ;
#4399=CARTESIAN_POINT ( 'NONE',  ( -15.40903463028481646, 43.45937500034139589, -47.42413220539093999 ) ) ;
#4400=CARTESIAN_POINT ( 'NONE',  ( -3.210462471511496205E-15, 47.35937500034138736, -52.43083105670540789 ) ) ;
#4413=ORIENTED_EDGE ( 'NONE', *, *, #73, .T. ) ;
#4414=CARTESIAN_POINT ( 'NONE',  ( 30.90169943749473802, 43.30000000000000426, -42.53254041760200721 ) ) ;
#4417=AXIS2_PLACEMENT_3D ( 'NONE', #82, #6, #1509 ) ;
#4422=VERTEX_POINT ( 'NONE', #14740 ) ;
#4425=CARTESIAN_POINT ( 'NONE',  ( 2.600676159226420495E-13, 23.50000000000000000, -49.99999999999999289 ) ) ;
#4430=CARTESIAN_POINT ( 'NONE',  ( 13.22646626819541282, 11.02685957165896014, 97.16024423813598787 ) ) ;
#4432=CARTESIAN_POINT ( 'NONE',  ( -15.40903463028480580, 24.32187500034139660, 47.42413220539094709 ) ) ;
#4435=CARTESIAN_POINT ( 'NONE',  ( 40.34137639590981195, 27.05937500034139731, -29.30972558990011834 ) ) ;
#4439=CARTESIAN_POINT ( 'NONE',  ( -40.45084971874737789, 29.80000000000000071, -29.38926261462365730 ) ) ;
#4447=CIRCLE ( 'NONE', #13718, 10.00000000000000000 ) ;
#4450=AXIS2_PLACEMENT_3D ( 'NONE', #4821, #14594, #10874 ) ;
#4452=CARTESIAN_POINT ( 'NONE',  ( -49.86468353125000164, 27.92187500034139447, 0.000000000000000000 ) ) ;
#4453=CARTESIAN_POINT ( 'NONE',  ( -30.81806926056962226, 36.15937500034139163, 42.41743335407647209 ) ) ;
#4454=CARTESIAN_POINT ( 'NONE',  ( -15.45084971874736368, 44.39999999999999858, 47.55282581475768211 ) ) ;
#4457=CARTESIAN_POINT ( 'NONE',  ( -40.34137639590981905, 45.65937500034139873, -29.30972558990011478 ) ) ;
#4459=CARTESIAN_POINT ( 'NONE',  ( 30.90169943749475578, 48.69999999999999574, 42.53254041760200010 ) ) ;
#4469=CARTESIAN_POINT ( 'NONE',  ( -49.86468353125000164, 47.92187500034139447, 0.000000000000000000 ) ) ;
#4473=CARTESIAN_POINT ( 'NONE',  ( -30.90169943749473802, 36.29999999999998295, 42.53254041760200721 ) ) ;
#4474=CARTESIAN_POINT ( 'NONE',  ( 9.631387414534489405E-15, 40.42187500034138736, 52.43083105670540789 ) ) ;
#4478=ORIENTED_EDGE ( 'NONE', *, *, #6749, .F. ) ;
#4480=( BOUNDED_CURVE ( )  B_SPLINE_CURVE ( 2, ( #8218, #7057, #16022, #11043, #10714, #883, #5977, #4650, #9715, #16113, #4745, #14853, #13284, #12032, #3481, #14679, #3398, #13606, #15942, #2132, #5729, #2211, #11957, #555, #9471, #4400, #14521, #8374, #634, #13448, #10805, #4488, #8464, #9553, #2057, #3223, #4564, #14600, #12122, #727, #9627, #7145, #806, #2695, #1363, #1050, #3561, #8707, #6534, #6625, #970, #2778, #7851, #11600, #197, #12931, #1536, #11678, #8614, #13687, #276, #5380, #10435, #11513, #16197, #15491, #4116, #9185, #14249, #7308, #4825, #12367, #6066, #15332, #11135, #9025, #9880, #14931, #10352, #2304, #10276, #13772, #12843, #11216, #7392, #14080, #6144, #12456, #9102, #7694, #1446, #16271, #4902, #9960, #15016, #3651, #2619, #5303, #7771, #15414, #12764, #4032, #6454, #5216, #109, #3951, #14162, #3023, #13250, #14565, #7936, #6872, #13169, #4286, #8094, #9518, #5691, #1778, #13087, #1612, #596, #6790, #11923, #523, #2946, #6705, #5618, #5456, #10681, #15733, #1928, #11834, #11755, #14329, #3189, #356, #1693, #4453, #4364, #5546, #9429, #14477, #3112, #8184, #445, #1850, #10521, #15583, #10608, #12075, #8013, #12000, #7021, #8262, #10759, #4208, #6946, #15819, #13326, #679, #5778, #9274, #15664, #9350, #10844, #4532, #15908, #14400, #9595, #13009, #2868, #9926, #16159, #768, #3609, #1014, #8669, #929, #5942, #8506, #2351, #3270, #4790, #13490, #8340, #16236, #14813, #3525, #10922, #9673, #7433, #12500, #850, #13738, #8577, #14898, #2260, #8428, #1093, #9846, #13402, #6185, #13571, #3444, #11259, #2098, #16317, #4952, #4610, #2014, #14642, #9766, #15984, #7356, #7271, #12247, #14980, #7186, #7111, #11005, #2175, #6027, #16067, #4700, #12327, #13652, #11099, #12423, #6111, #11182, #4870, #5858, #12166, #14723, #3354, #8752, #10248, #15310, #6353, #7673, #10169, #9003, #3932, #7831, #13815, #11339, #2597, #1263, #5114, #15219, #14061, #11419, #11491, #3849, #179, #11572, #12, #1341, #2756, #16406, #7504, #2427, #5039, #2677, #12575, #5193, #8914, #3770, #6268, #13979, #7751, #9084, #3696, #5283, #10334, #12820, #1421, #15394, #4014, #14140, #10094, #12906, #1173, #1516, #6606, #12744, #15142, #11660, #257, #6432, #89, #6514, #10011, #15067, #8829, #13892, #2508, #7587, #12665, #11816, #13148 ),
 .UNSPECIFIED., .F., .F. ) 
 B_SPLINE_CURVE_WITH_KNOTS ( ( 3, 2, 2, 2, 2, 2, 2, 2, 2, 2, 2, 2, 2, 2, 2, 2, 2, 2, 2, 2, 2, 2, 2, 2, 2, 2, 2, 2, 2, 2, 2, 2, 2, 2, 2, 2, 2, 2, 2, 2, 2, 2, 2, 2, 2, 2, 2, 2, 2, 2, 2, 2, 2, 2, 2, 2, 2, 2, 2, 2, 2, 2, 2, 2, 2, 2, 2, 2, 2, 2, 2, 2, 2, 2, 2, 2, 2, 2, 2, 2, 2, 2, 2, 2, 2, 2, 2, 2, 2, 2, 2, 2, 2, 2, 2, 2, 2, 2, 2, 2, 2, 2, 2, 2, 2, 2, 2, 2, 2, 2, 2, 2, 2, 2, 2, 2, 2, 2, 2, 2, 2, 2, 2, 2, 2, 2, 2, 2, 2, 2, 2, 2, 2, 2, 2, 2, 2, 2, 2, 2, 2, 2, 2, 2, 2, 2, 2, 2, 2, 2, 3 ),
 ( 0.000000000000000000, 0.006666666666666667095, 0.01333333333333333419, 0.02000000000000000042, 0.02666666666666666838, 0.03333333333333333287, 0.04000000000000000083, 0.04666666666666666879, 0.05333333333333333676, 0.05999999999999999778, 0.06666666666666666574, 0.07333333333333333370, 0.08000000000000000167, 0.08666666666666666963, 0.09333333333333333759, 0.1000000000000000056, 0.1066666666666666735, 0.1133333333333333276, 0.1199999999999999956, 0.1266666666666666774, 0.1333333333333333315, 0.1400000000000000133, 0.1466666666666666674, 0.1533333333333333215, 0.1600000000000000033, 0.1666666666666666574, 0.1733333333333333393, 0.1799999999999999933, 0.1866666666666666752, 0.1933333333333333293, 0.2000000000000000111, 0.2066666666666666652, 0.2133333333333333470, 0.2200000000000000011, 0.2266666666666666552, 0.2333333333333333370, 0.2399999999999999911, 0.2466666666666666730, 0.2533333333333333548, 0.2600000000000000089, 0.2666666666666666630, 0.2733333333333333171, 0.2800000000000000266, 0.2866666666666666807, 0.2933333333333333348, 0.2999999999999999889, 0.3066666666666666430, 0.3133333333333333526, 0.3200000000000000067, 0.3266666666666666607, 0.3333333333333333148, 0.3400000000000000244, 0.3466666666666666785, 0.3533333333333333326, 0.3599999999999999867, 0.3666666666666666408, 0.3733333333333333504, 0.3800000000000000044, 0.3866666666666666585, 0.3933333333333333126, 0.4000000000000000222, 0.4066666666666666763, 0.4133333333333333304, 0.4199999999999999845, 0.4266666666666666941, 0.4333333333333333481, 0.4400000000000000022, 0.4466666666666666563, 0.4533333333333333104, 0.4600000000000000200, 0.4666666666666666741, 0.4733333333333333282, 0.4799999999999999822, 0.4866666666666666918, 0.4933333333333333459, 0.5000000000000000000, 0.5066666666666667096, 0.5133333333333333082, 0.5200000000000000178, 0.5266666666666666163, 0.5333333333333333259, 0.5400000000000000355, 0.5466666666666666341, 0.5533333333333333437, 0.5600000000000000533, 0.5666666666666666519, 0.5733333333333333615, 0.5799999999999999600, 0.5866666666666666696, 0.5933333333333333792, 0.5999999999999999778, 0.6066666666666666874, 0.6133333333333332860, 0.6199999999999999956, 0.6266666666666667052, 0.6333333333333333037, 0.6400000000000000133, 0.6466666666666666119, 0.6533333333333333215, 0.6600000000000000311, 0.6666666666666666297, 0.6733333333333333393, 0.6800000000000000488, 0.6866666666666666474, 0.6933333333333333570, 0.6999999999999999556, 0.7066666666666666652, 0.7133333333333333748, 0.7199999999999999734, 0.7266666666666666829, 0.7333333333333332815, 0.7399999999999999911, 0.7466666666666667007, 0.7533333333333332993, 0.7600000000000000089, 0.7666666666666667185, 0.7733333333333333171, 0.7800000000000000266, 0.7866666666666666252, 0.7933333333333333348, 0.8000000000000000444, 0.8066666666666666430, 0.8133333333333333526, 0.8199999999999999512, 0.8266666666666666607, 0.8333333333333333703, 0.8399999999999999689, 0.8466666666666666785, 0.8533333333333333881, 0.8599999999999999867, 0.8666666666666666963, 0.8733333333333332948, 0.8800000000000000044, 0.8866666666666667140, 0.8933333333333333126, 0.9000000000000000222, 0.9066666666666666208, 0.9133333333333333304, 0.9200000000000000400, 0.9266666666666666385, 0.9333333333333333481, 0.9399999999999999467, 0.9466666666666666563, 0.9533333333333333659, 0.9599999999999999645, 0.9666666666666666741, 0.9733333333333333837, 0.9799999999999999822, 0.9866666666666666918, 0.9933333333333332904, 0.9953403926135619972 ),
 .UNSPECIFIED. ) 
 CURVE ( )  GEOMETRIC_REPRESENTATION_ITEM ( )  RATIONAL_B_SPLINE_CURVE ( ( 1.000000000000000000, 0.9510565162951535312, 1.000000000000000000, 0.9510565162951535312, 1.000000000000000000, 0.9510565162951535312, 1.000000000000000000, 0.9510565162951535312, 1.000000000000000000, 0.9510565162951535312, 1.000000000000000000, 0.9510565162951535312, 1.000000000000000000, 0.9510565162951535312, 1.000000000000000000, 0.9510565162951535312, 1.000000000000000000, 0.9510565162951535312, 1.000000000000000000, 0.9510565162951535312, 1.000000000000000000, 0.9510565162951535312, 1.000000000000000000, 0.9510565162951535312, 1.000000000000000000, 0.9510565162951535312, 1.000000000000000000, 0.9510565162951535312, 1.000000000000000000, 0.9510565162951535312, 1.000000000000000000, 0.9510565162951535312, 1.000000000000000000, 0.9510565162951535312, 1.000000000000000000, 0.9510565162951535312, 1.000000000000000000, 0.9510565162951535312, 1.000000000000000000, 0.9510565162951535312, 1.000000000000000000, 0.9510565162951535312, 1.000000000000000000, 0.9510565162951535312, 1.000000000000000000, 0.9510565162951535312, 1.000000000000000000, 0.9510565162951535312, 1.000000000000000000, 0.9510565162951535312, 1.000000000000000000, 0.9510565162951535312, 1.000000000000000000, 0.9510565162951535312, 1.000000000000000000, 0.9510565162951535312, 1.000000000000000000, 0.9510565162951535312, 1.000000000000000000, 0.9510565162951535312, 1.000000000000000000, 0.9510565162951535312, 1.000000000000000000, 0.9510565162951535312, 1.000000000000000000, 0.9510565162951535312, 1.000000000000000000, 0.9510565162951535312, 1.000000000000000000, 0.9510565162951535312, 1.000000000000000000, 0.9510565162951535312, 1.000000000000000000, 0.9510565162951535312, 1.000000000000000000, 0.9510565162951535312, 1.000000000000000000, 0.9510565162951535312, 1.000000000000000000, 0.9510565162951535312, 1.000000000000000000, 0.9510565162951535312, 1.000000000000000000, 0.9510565162951535312, 1.000000000000000000, 0.9510565162951535312, 1.000000000000000000, 0.9510565162951535312, 1.000000000000000000, 0.9510565162951535312, 1.000000000000000000, 0.9510565162951535312, 1.000000000000000000, 0.9510565162951535312, 1.000000000000000000, 0.9510565162951535312, 1.000000000000000000, 0.9510565162951535312, 1.000000000000000000, 0.9510565162951535312, 1.000000000000000000, 0.9510565162951535312, 1.000000000000000000, 0.9510565162951535312, 1.000000000000000000, 0.9510565162951535312, 1.000000000000000000, 0.9510565162951535312, 1.000000000000000000, 0.9510565162951535312, 1.000000000000000000, 0.9510565162951535312, 1.000000000000000000, 0.9510565162951535312, 1.000000000000000000, 0.9510565162951535312, 1.000000000000000000, 0.9510565162951535312, 1.000000000000000000, 0.9510565162951535312, 1.000000000000000000, 0.9510565162951535312, 1.000000000000000000, 0.9510565162951535312, 1.000000000000000000, 0.9510565162951535312, 1.000000000000000000, 0.9510565162951535312, 1.000000000000000000, 0.9510565162951535312, 1.000000000000000000, 0.9510565162951535312, 1.000000000000000000, 0.9510565162951535312, 1.000000000000000000, 0.9510565162951535312, 1.000000000000000000, 0.9510565162951535312, 1.000000000000000000, 0.9510565162951535312, 1.000000000000000000, 0.9510565162951535312, 1.000000000000000000, 0.9510565162951535312, 1.000000000000000000, 0.9510565162951535312, 1.000000000000000000, 0.9510565162951535312, 1.000000000000000000, 0.9510565162951535312, 1.000000000000000000, 0.9510565162951535312, 1.000000000000000000, 0.9510565162951535312, 1.000000000000000000, 0.9510565162951535312, 1.000000000000000000, 0.9510565162951535312, 1.000000000000000000, 0.9510565162951535312, 1.000000000000000000, 0.9510565162951535312, 1.000000000000000000, 0.9510565162951535312, 1.000000000000000000, 0.9510565162951535312, 1.000000000000000000, 0.9510565162951535312, 1.000000000000000000, 0.9510565162951535312, 1.000000000000000000, 0.9510565162951535312, 1.000000000000000000, 0.9510565162951535312, 1.000000000000000000, 0.9510565162951535312, 1.000000000000000000, 0.9510565162951535312, 1.000000000000000000, 0.9510565162951535312, 1.000000000000000000, 0.9510565162951535312, 1.000000000000000000, 0.9510565162951535312, 1.000000000000000000, 0.9510565162951535312, 1.000000000000000000, 0.9510565162951535312, 1.000000000000000000, 0.9510565162951535312, 1.000000000000000000, 0.9510565162951535312, 1.000000000000000000, 0.9510565162951535312, 1.000000000000000000, 0.9510565162951535312, 1.000000000000000000, 0.9510565162951535312, 1.000000000000000000, 0.9510565162951535312, 1.000000000000000000, 0.9510565162951535312, 1.000000000000000000, 0.9510565162951535312, 1.000000000000000000, 0.9510565162951535312, 1.000000000000000000, 0.9510565162951535312, 1.000000000000000000, 0.9510565162951535312, 1.000000000000000000, 0.9510565162951535312, 1.000000000000000000, 0.9510565162951535312, 1.000000000000000000, 0.9510565162951535312, 1.000000000000000000, 0.9510565162951535312, 1.000000000000000000, 0.9510565162951535312, 1.000000000000000000, 0.9510565162951535312, 1.000000000000000000, 0.9510565162951535312, 1.000000000000000000, 0.9510565162951535312, 1.000000000000000000, 0.9510565162951535312, 1.000000000000000000, 0.9510565162951535312, 1.000000000000000000, 0.9510565162951535312, 1.000000000000000000, 0.9510565162951535312, 1.000000000000000000, 0.9510565162951535312, 1.000000000000000000, 0.9510565162951535312, 1.000000000000000000, 0.9510565162951535312, 1.000000000000000000, 0.9510565162951535312, 1.000000000000000000, 0.9510565162951535312, 1.000000000000000000, 0.9510565162951535312, 1.000000000000000000, 0.9510565162951535312, 1.000000000000000000, 0.9510565162951535312, 1.000000000000000000, 0.9510565162951535312, 1.000000000000000000, 0.9510565162951535312, 1.000000000000000000, 0.9510565162951535312, 1.000000000000000000, 0.9510565162951535312, 1.000000000000000000, 0.9510565162951535312, 1.000000000000000000, 0.9510565162951535312, 1.000000000000000000, 0.9510565162951535312, 1.000000000000000000, 0.9510565162951535312, 1.000000000000000000, 0.9510565162951535312, 1.000000000000000000, 0.9510565162951535312, 1.000000000000000000, 0.9510565162951535312, 1.000000000000000000, 0.9510565162951535312, 1.000000000000000000, 0.9510565162951535312, 1.000000000000000000, 0.9510565162951535312, 1.000000000000000000, 0.9510565162951535312, 1.000000000000000000, 0.9510565162951535312, 1.000000000000000000, 0.9510565162951535312, 1.000000000000000000, 0.9510565162951535312, 1.000000000000000000, 0.9510565162951535312, 1.000000000000000000, 0.9510565162951535312, 1.000000000000000000, 0.9510565162951535312, 1.000000000000000000, 0.9510565162951535312, 1.000000000000000000, 0.9510565162951535312, 1.000000000000000000, 0.9510565162951535312, 1.000000000000000000, 0.9852651290235199255, 0.9794023859079349359 ) ) 
 REPRESENTATION_ITEM ( '' )  );
#4487=CARTESIAN_POINT ( 'NONE',  ( 40.34137639590981905, 42.65937500034139873, 29.30972558990010768 ) ) ;
#4488=CARTESIAN_POINT ( 'NONE',  ( 49.86468353125001585, 46.75937500034140015, 16.20201782572375038 ) ) ;
#4493=CARTESIAN_POINT ( 'NONE',  ( -15.45084971874736368, 36.18125000068280173, 47.55282581475768211 ) ) ;
#4504=CARTESIAN_POINT ( 'NONE',  ( -40.45084971874737789, 39.80000000000000426, -29.38926261462365730 ) ) ;
#4506=ORIENTED_EDGE ( 'NONE', *, *, #7834, .T. ) ;
#4510=DIRECTION ( 'NONE',  ( 0.000000000000000000, 0.000000000000000000, 1.000000000000000000 ) ) ;
#4511=DIRECTION ( 'NONE',  ( 0.000000000000000000, 1.000000000000000000, 0.000000000000000000 ) ) ;
#4512=CARTESIAN_POINT ( 'NONE',  ( -40.45084971874737079, 48.20000000000000284, 29.38926261462367151 ) ) ;
#4516=CARTESIAN_POINT ( 'NONE',  ( 40.34137639590981195, 25.12187500034139376, -29.30972558990011834 ) ) ;
#4520=CARTESIAN_POINT ( 'NONE',  ( -3.210462471511496205E-15, 23.35937500034139802, -52.43083105670540789 ) ) ;
#4523=ORIENTED_EDGE ( 'NONE', *, *, #16244, .F. ) ;
#4526=FACE_OUTER_BOUND ( 'NONE', #2749, .T. ) ;
#4531=CARTESIAN_POINT ( 'NONE',  ( 49.86468353125001585, 28.82187500034139305, 16.20201782572375038 ) ) ;
#4532=CARTESIAN_POINT ( 'NONE',  ( -3.210462471511496205E-15, 33.35937500034139447, -52.43083105670540789 ) ) ;
#4533=CARTESIAN_POINT ( 'NONE',  ( -40.45084971874737079, 36.20000000000000284, 29.38926261462367151 ) ) ;
#4536=CARTESIAN_POINT ( 'NONE',  ( 40.34137639590981195, 43.05937500034139731, -29.30972558990011834 ) ) ;
#4538=CARTESIAN_POINT ( 'NONE',  ( 30.81806926056964002, 22.62187500034139731, 42.41743335407647209 ) ) ;
#4547=CARTESIAN_POINT ( 'NONE',  ( -49.86468353124999453, 45.82187500034140015, -16.20201782572375393 ) ) ;
#4551=CARTESIAN_POINT ( 'NONE',  ( 40.45084971874737789, 36.79999999999999716, 29.38926261462365375 ) ) ;
#4552=CARTESIAN_POINT ( 'NONE',  ( -15.40903463028481646, 41.52187500034139589, -47.42413220539093999 ) ) ;
#4561=DIRECTION ( 'NONE',  ( 0.000000000000000000, -1.000000000000000000, 0.000000000000000000 ) ) ;
#4562=CARTESIAN_POINT ( 'NONE',  ( -15.45084971874736368, 20.40000000000000213, 47.55282581475768211 ) ) ;
#4563=CARTESIAN_POINT ( 'NONE',  ( -15.40903463028480580, 36.25937500034140015, 47.42413220539094709 ) ) ;
#4564=CARTESIAN_POINT ( 'NONE',  ( -15.40903463028480580, 46.25937500034140015, 47.42413220539094709 ) ) ;
#4569=CARTESIAN_POINT ( 'NONE',  ( 50.00000000000000000, 37.00000000000000711, -6.123233995736766085E-15 ) ) ;
#4572=( BOUNDED_CURVE ( )  B_SPLINE_CURVE ( 2, ( #6106, #1088, #8745, #3520, #11254 ),
 .UNSPECIFIED., .F., .F. ) 
 B_SPLINE_CURVE_WITH_KNOTS ( ( 3, 2, 3 ),
 ( 0.9833333333333333925, 0.9866666666666666918, 0.9926850605967240115 ),
 .UNSPECIFIED. ) 
 CURVE ( )  GEOMETRIC_REPRESENTATION_ITEM ( )  RATIONAL_B_SPLINE_CURVE ( ( 0.9755282581475768211, 0.9755282581475771542, 1.000000000000000000, 0.9558158252132334942, 0.9914069812288479611 ) ) 
 REPRESENTATION_ITEM ( '' )  );
#4575=ORIENTED_EDGE ( 'NONE', *, *, #5307, .T. ) ;
#4581=CARTESIAN_POINT ( 'NONE',  ( -1.240322475938754499E-13, 38.50000000000000711, 50.00000000000000000 ) ) ;
#4582=CARTESIAN_POINT ( 'NONE',  ( -16.61395733222127191, 16.88676649784340711, 95.59049725886258386 ) ) ;
#4585=DIRECTION ( 'NONE',  ( 0.000000000000000000, 0.000000000000000000, 1.000000000000000000 ) ) ;
#4588=CARTESIAN_POINT ( 'NONE',  ( 2.978552182361884590E-14, 47.50000000000000711, -50.00000000000000000 ) ) ;
#4589=CARTESIAN_POINT ( 'NONE',  ( -45.11452830843730766, 20.00000000000000711, 21.24066852005664430 ) ) ;
#4590=CARTESIAN_POINT ( 'NONE',  ( 15.40903463028481113, 21.32187500034139660, -47.42413220539094709 ) ) ;
#4594=CARTESIAN_POINT ( 'NONE',  ( -49.86468353125000164, 27.85937500034139447, 0.000000000000000000 ) ) ;
#4595=EDGE_CURVE ( 'NONE', #11668, #9978, #14160, .T. ) ;
#4598=ORIENTED_EDGE ( 'NONE', *, *, #7340, .F. ) ;
#4603=EDGE_LOOP ( 'NONE', ( #4478, #4523, #5751, #8023, #2627, #12773, #14732, #11520, #9320, #3180, #4145, #2991, #13336, #12627, #11801, #9300, #3643, #2722, #13559, #9952, #2923, #3261, #3279, #8587, #13037, #3213, #14447, #2004, #1508, #12090, #6138, #6401, #12588, #7366 ) ) ;
#4606=DIRECTION ( 'NONE',  ( 0.000000000000000000, 1.000000000000000000, 0.000000000000000000 ) ) ;
#4607=CARTESIAN_POINT ( 'NONE',  ( -1.240322475938754499E-13, 40.50000000000000000, 50.00000000000000000 ) ) ;
#4608=CARTESIAN_POINT ( 'NONE',  ( 1.293669679204937499E-13, 39.50000000000000711, -50.00000000000000000 ) ) ;
#4609=CARTESIAN_POINT ( 'NONE',  ( -40.34137639590981905, 31.72187500034139873, -29.30972558990011478 ) ) ;
#4610=CARTESIAN_POINT ( 'NONE',  ( 40.34137639590981195, 29.05937500034139376, -29.30972558990011834 ) ) ;
#4615=CARTESIAN_POINT ( 'NONE',  ( 15.40903463028481113, 47.25937500034140015, -47.42413220539094709 ) ) ;
#4617=CARTESIAN_POINT ( 'NONE',  ( 30.81806926056964002, 20.62187500034139020, 42.41743335407647209 ) ) ;
#4619=EDGE_LOOP ( 'NONE', ( #8127, #405, #4257, #288 ) ) ;
#4628=CARTESIAN_POINT ( 'NONE',  ( -15.40903463028480580, 20.25937500034139660, 47.42413220539094709 ) ) ;
#4632=CARTESIAN_POINT ( 'NONE',  ( 15.45084971874737789, 34.38125000068280457, 47.55282581475767500 ) ) ;
#4633=CARTESIAN_POINT ( 'NONE',  ( 15.45084971874737789, 38.60000000000000142, 47.55282581475767500 ) ) ;
#4634=CARTESIAN_POINT ( 'NONE',  ( -15.40903463028480580, 40.32187500034140015, 47.42413220539094709 ) ) ;
#4647=CARTESIAN_POINT ( 'NONE',  ( 15.45084971874737789, 26.60000000000000142, 47.55282581475767500 ) ) ;
#4648=CARTESIAN_POINT ( 'NONE',  ( -49.99999999999999289, 20.09999999999999787, 16.24598481164533226 ) ) ;
#4649=CARTESIAN_POINT ( 'NONE',  ( 40.34137639590981905, 34.65937500034139873, 29.30972558990010768 ) ) ;
#4650=CARTESIAN_POINT ( 'NONE',  ( 30.81806926056962936, 49.15937500034139163, -42.41743335407646498 ) ) ;
#4652=CARTESIAN_POINT ( 'NONE',  ( 2.600676159226421000E-13, 33.28125000068279604, -49.99999999999999289 ) ) ;
#4653=CARTESIAN_POINT ( 'NONE',  ( -5.823736356558309156E-14, 44.50000000000000000, 50.00000000000000000 ) ) ;
#4665=CARTESIAN_POINT ( 'NONE',  ( 40.45084971874737789, 28.80000000000000426, 29.38926261462365375 ) ) ;
#4666=ORIENTED_EDGE ( 'NONE', *, *, #294, .F. ) ;
#4667=CARTESIAN_POINT ( 'NONE',  ( -30.90169943749473447, 48.08125000068279320, 42.53254041760200721 ) ) ;
#4669=CARTESIAN_POINT ( 'NONE',  ( -10.75298028539202200, 8.646267545471964411, 97.89130469945834534 ) ) ;
#4670=CYLINDRICAL_SURFACE ( 'NONE', #12393, 50.00000000000000000 ) ;
#4677=CARTESIAN_POINT ( 'NONE',  ( -45.60931600130317776, 20.00000000000001066, 20.15700215907655135 ) ) ;
#4678=CARTESIAN_POINT ( 'NONE',  ( -40.34137639590981905, 23.72187500034139873, -29.30972558990011478 ) ) ;
#4683=CARTESIAN_POINT ( 'NONE',  ( -15.40903463028480580, 26.25937500034140015, 47.42413220539094709 ) ) ;
#4684=CARTESIAN_POINT ( 'NONE',  ( -7.919222016226773242, 42.22999571913594963, 50.00000000000000711 ) ) ;
#4695=CARTESIAN_POINT ( 'NONE',  ( 15.45084971874736723, 35.39999999999999858, -47.55282581475768211 ) ) ;
#4699=CARTESIAN_POINT ( 'NONE',  ( -3.210462471511496205E-15, 31.42187500034139447, -52.43083105670540789 ) ) ;
#4700=CARTESIAN_POINT ( 'NONE',  ( -30.81806926056963292, 27.55937500034139376, -42.41743335407646498 ) ) ;
#4708=CARTESIAN_POINT ( 'NONE',  ( 40.34137639590981195, 45.05937500034139731, -29.30972558990011834 ) ) ;
#4711=CARTESIAN_POINT ( 'NONE',  ( 15.40903463028481113, 21.32187500034139660, -47.42413220539094709 ) ) ;
#4716=VERTEX_POINT ( 'NONE', #3441 ) ;
#4721=ORIENTED_EDGE ( 'NONE', *, *, #14864, .F. ) ;
#4724=CARTESIAN_POINT ( 'NONE',  ( -49.86468353124999453, 46.02187500034140299, 16.20201782572377525 ) ) ;
#4729=CARTESIAN_POINT ( 'NONE',  ( -49.99999999999999289, 35.68125000068278752, -16.24598481164531449 ) ) ;
#4731=CARTESIAN_POINT ( 'NONE',  ( -30.81806926056963292, 37.62187500034139020, -42.41743335407647209 ) ) ;
#4733=VERTEX_POINT ( 'NONE', #4608 ) ;
#4736=PLANE ( 'NONE',  #9457 ) ;
#4742=FACE_OUTER_BOUND ( 'NONE', #14988, .T. ) ;
#4743=CARTESIAN_POINT ( 'NONE',  ( 15.45084971874737789, 20.60000000000000142, 47.55282581475767500 ) ) ;
#4744=CARTESIAN_POINT ( 'NONE',  ( 15.40903463028482356, 36.45937500034139589, 47.42413220539093999 ) ) ;
#4745=CARTESIAN_POINT ( 'NONE',  ( 49.86468353125000164, 48.85937500034139447, -6.106662507704105588E-15 ) ) ;
#4746=CARTESIAN_POINT ( 'NONE',  ( -3.111920190527341144E-15, 25.50000000000000355, -50.00000000000000000 ) ) ;
#4747=CARTESIAN_POINT ( 'NONE',  ( -40.34137639590981905, 49.72187500034139873, -29.30972558990011478 ) ) ;
#4749=LINE ( 'NONE', #14684, #6575 ) ;
#4753=ORIENTED_EDGE ( 'NONE', *, *, #10033, .T. ) ;
#4760=CARTESIAN_POINT ( 'NONE',  ( 8.446640517145639571E-15, 28.49999999999999645, 50.00000000000000000 ) ) ;
#4764=CARTESIAN_POINT ( 'NONE',  ( 1.235979693235591175E-19, 4.999999999999997335, 99.11836509645767990 ) ) ;
#4765=FACE_OUTER_BOUND ( 'NONE', #10137, .T. ) ;
#4771=CARTESIAN_POINT ( 'NONE',  ( 50.00000000000000000, 44.78125000068280315, -6.123233995736766085E-15 ) ) ;
#4789=CARTESIAN_POINT ( 'NONE',  ( -15.40903463028481646, 27.52187500034139944, -47.42413220539093999 ) ) ;
#4790=CARTESIAN_POINT ( 'NONE',  ( -40.34137639590981905, 31.65937500034139873, -29.30972558990011478 ) ) ;
#4792=CARTESIAN_POINT ( 'NONE',  ( 15.40903463028482356, 36.52187500034139589, 47.42413220539093999 ) ) ;
#4794=CARTESIAN_POINT ( 'NONE',  ( 15.40903463028482356, 44.45937500034139589, 47.42413220539093999 ) ) ;
#4796=CARTESIAN_POINT ( 'NONE',  ( -40.45084971874737079, 46.20000000000000284, 29.38926261462367151 ) ) ;
#4805=DIRECTION ( 'NONE',  ( 0.000000000000000000, 0.000000000000000000, 1.000000000000000000 ) ) ;
#4807=CARTESIAN_POINT ( 'NONE',  ( 49.86468353124999453, 49.02187500034140299, -16.20201782572376459 ) ) ;
#4811=CARTESIAN_POINT ( 'NONE',  ( -49.99999999999999289, 33.88125000068280457, 16.24598481164533226 ) ) ;
#4812=CARTESIAN_POINT ( 'NONE',  ( -30.81806926056963292, 39.62187500034138310, -42.41743335407647209 ) ) ;
#4814=ORIENTED_EDGE ( 'NONE', *, *, #8129, .T. ) ;
#4821=CARTESIAN_POINT ( 'NONE',  ( 0.000000000000000000, 20.00000000000000355, 0.000000000000000000 ) ) ;
#4823=CARTESIAN_POINT ( 'NONE',  ( -15.45084971874737256, 23.38125000068280102, -47.55282581475767500 ) ) ;
#4824=CARTESIAN_POINT ( 'NONE',  ( -15.40903463028481646, 37.45937500034139589, -47.42413220539093999 ) ) ;
#4825=CARTESIAN_POINT ( 'NONE',  ( 49.86468353125000164, 42.85937500034140157, -6.106662507704105588E-15 ) ) ;
#4826=CARTESIAN_POINT ( 'NONE',  ( 30.90169943749475223, 24.69999999999999929, 42.53254041760199300 ) ) ;
#4834=EDGE_LOOP ( 'NONE', ( #11539, #16034, #16189, #7982 ) ) ;
#4835=VERTEX_POINT ( 'NONE', #15982 ) ;
#4840=FILL_AREA_STYLE ('',( #3577 ) ) ;
#4842=CARTESIAN_POINT ( 'NONE',  ( -15.45084971874736368, 48.18125000068280173, 47.55282581475768211 ) ) ;
#4847=LINE ( 'NONE', #906, #5029 ) ;
#4851=CARTESIAN_POINT ( 'NONE',  ( -30.90169943749474868, 45.48125000068279178, -42.53254041760200721 ) ) ;
#4854=CARTESIAN_POINT ( 'NONE',  ( -15.45084971874736368, 26.40000000000000213, 47.55282581475768211 ) ) ;
#4855=CARTESIAN_POINT ( 'NONE',  ( -50.00000000000000000, 41.78125000068280315, 0.000000000000000000 ) ) ;
#4859=ORIENTED_EDGE ( 'NONE', *, *, #7453, .F. ) ;
#4862=CARTESIAN_POINT ( 'NONE',  ( 7.919222016226818539, 49.44874571845315359, -50.00000000000000000 ) ) ;
#4867=CARTESIAN_POINT ( 'NONE',  ( -3.111920190527341144E-15, 35.50000000000000000, -50.00000000000000000 ) ) ;
#4869=CARTESIAN_POINT ( 'NONE',  ( 15.40903463028482356, 20.52187500034139589, 47.42413220539093999 ) ) ;
#4870=CARTESIAN_POINT ( 'NONE',  ( 49.86468353125000164, 26.85937500034139802, -6.106662507704105588E-15 ) ) ;
#4871=CARTESIAN_POINT ( 'NONE',  ( -15.45084971874737256, 35.60000000000000142, -47.55282581475767500 ) ) ;
#4872=CARTESIAN_POINT ( 'NONE',  ( -49.86468353125000164, 37.92187500034140157, 0.000000000000000000 ) ) ;
#4873=DIRECTION ( 'NONE',  ( -0.000000000000000000, -1.000000000000000000, -0.000000000000000000 ) ) ;
#4874=CARTESIAN_POINT ( 'NONE',  ( 40.34137639590981195, 41.05937500034139731, -29.30972558990011834 ) ) ;
#4876=CARTESIAN_POINT ( 'NONE',  ( -40.45084971874737079, 48.20000000000000284, 29.38926261462367151 ) ) ;
#4877=VERTEX_POINT ( 'NONE', #3606 ) ;
#4879=ORIENTED_EDGE ( 'NONE', *, *, #3752, .F. ) ;
#4881=( BOUNDED_CURVE ( )  B_SPLINE_CURVE ( 2, ( #14442, #13130, #11885, #15700, #6983, #10810, #7899, #4169, #560, #9238, #14291, #2913, #12038 ),
 .UNSPECIFIED., .F., .T. ) 
 B_SPLINE_CURVE_WITH_KNOTS ( ( 3, 2, 2, 2, 2, 2, 3 ),
 ( 0.8833333333333334147, 0.8866666666666667140, 0.8933333333333333126, 0.9000000000000000222, 0.9066666666666666208, 0.9133333333333333304, 0.9166666666666667407 ),
 .UNSPECIFIED. ) 
 CURVE ( )  GEOMETRIC_REPRESENTATION_ITEM ( )  RATIONAL_B_SPLINE_CURVE ( ( 0.9755282581475768211, 0.9755282581475771542, 1.000000000000000000, 0.9510565162951535312, 1.000000000000000000, 0.9510565162951535312, 1.000000000000000000, 0.9510565162951535312, 1.000000000000000000, 0.9510565162951535312, 1.000000000000000000, 0.9755282581475763770, 0.9755282581475768211 ) ) 
 REPRESENTATION_ITEM ( '' )  );
#4882=CARTESIAN_POINT ( 'NONE',  ( -15.45084971874736368, 34.39999999999999858, 47.55282581475768211 ) ) ;
#4885=CARTESIAN_POINT ( 'NONE',  ( -49.86468353125000164, 41.92187500034139447, 0.000000000000000000 ) ) ;
#4888=CARTESIAN_POINT ( 'NONE',  ( 30.90169943749474157, 27.08125000068280031, -42.53254041760200721 ) ) ;
#4889=CARTESIAN_POINT ( 'NONE',  ( 15.40903463028481113, 37.32187500034140015, -47.42413220539094709 ) ) ;
#4893=ORIENTED_EDGE ( 'NONE', *, *, #2451, .T. ) ;
#4896=VERTEX_POINT ( 'NONE', #3768 ) ;
#4901=CARTESIAN_POINT ( 'NONE',  ( 15.40903463028481113, 35.25937500034139305, -47.42413220539094709 ) ) ;
#4902=CARTESIAN_POINT ( 'NONE',  ( 40.34137639590981905, 40.65937500034139873, 29.30972558990010768 ) ) ;
#4904=DIRECTION ( 'NONE',  ( 0.000000000000000000, -1.000000000000000000, 0.000000000000000000 ) ) ;
#4905=EDGE_CURVE ( 'NONE', #12450, #4999, #13890, .T. ) ;
#4906=AXIS2_PLACEMENT_3D ( 'NONE', #6167, #5018, #8895 ) ;
#4927=CARTESIAN_POINT ( 'NONE',  ( -2.902026171381852926, 5.232512297988552774, 99.03650175003853917 ) ) ;
#4931=DIRECTION ( 'NONE',  ( -0.000000000000000000, 1.000000000000000000, -0.000000000000000000 ) ) ;
#4932=( NAMED_UNIT ( * ) PLANE_ANGLE_UNIT ( ) SI_UNIT ( $, .RADIAN. ) );
#4934=CARTESIAN_POINT ( 'NONE',  ( 40.45084971874737079, 48.98125000068279888, -29.38926261462366440 ) ) ;
#4938=CARTESIAN_POINT ( 'NONE',  ( -40.34137639590981195, 20.05937500034139731, 29.30972558990012189 ) ) ;
#4942=CARTESIAN_POINT ( 'NONE',  ( 0.000000000000000000, 22.50000000000000000, 102.0000000000000142 ) ) ;
#4951=CARTESIAN_POINT ( 'NONE',  ( -49.86468353124999453, 21.82187500034139305, -16.20201782572375393 ) ) ;
#4952=CARTESIAN_POINT ( 'NONE',  ( 30.81806926056962936, 29.15937500034139518, -42.41743335407646498 ) ) ;
#4954=CARTESIAN_POINT ( 'NONE',  ( -40.34137639590981195, 38.12187500034139731, 29.30972558990012189 ) ) ;
#4956=CARTESIAN_POINT ( 'NONE',  ( 50.00000000000000711, 36.89999999999999858, 16.24598481164530739 ) ) ;
#4957=CARTESIAN_POINT ( 'NONE',  ( -40.34137639590981905, 37.65937500034139873, -29.30972558990011478 ) ) ;
#4961=CARTESIAN_POINT ( 'NONE',  ( 15.45084971874736723, 45.40000000000000568, -47.55282581475768211 ) ) ;
#4973=CARTESIAN_POINT ( 'NONE',  ( -15.40903463028480580, 40.32187500034140015, 47.42413220539094709 ) ) ;
#4974=DIRECTION ( 'NONE',  ( 0.000000000000000000, 0.000000000000000000, 1.000000000000000000 ) ) ;
#4976=CARTESIAN_POINT ( 'NONE',  ( -40.45084971874737789, 27.58125000068280031, -29.38926261462365730 ) ) ;
#4977=CARTESIAN_POINT ( 'NONE',  ( -15.40903463028481646, 35.52187500034139589, -47.42413220539093999 ) ) ;
#4988=CARTESIAN_POINT ( 'NONE',  ( -7.919222016226934890, 24.22999571913595673, 49.99999999999996447 ) ) ;
#4991=CARTESIAN_POINT ( 'NONE',  ( -30.81806926056963292, 29.55937500034139376, -42.41743335407647209 ) ) ;
#4994=CARTESIAN_POINT ( 'NONE',  ( -49.86468353124999453, 48.02187500034139589, 16.20201782572377169 ) ) ;
#4998=CARTESIAN_POINT ( 'NONE',  ( -30.90169943749474513, 41.70000000000000284, -42.53254041760200721 ) ) ;
#4999=VERTEX_POINT ( 'NONE', #3694 ) ;
#5012=DIRECTION ( 'NONE',  ( 0.000000000000000000, 0.000000000000000000, 1.000000000000000000 ) ) ;
#5013=CARTESIAN_POINT ( 'NONE',  ( 40.34137639590981905, 48.65937500034139873, 29.30972558990010768 ) ) ;
#5018=DIRECTION ( 'NONE',  ( -0.000000000000000000, -1.000000000000000000, -0.000000000000000000 ) ) ;
#5019=CARTESIAN_POINT ( 'NONE',  ( 40.45084971874737789, 46.58125000068280031, 29.38926261462365375 ) ) ;
#5020=CARTESIAN_POINT ( 'NONE',  ( 40.45084971874737079, 21.19999999999999929, -29.38926261462366440 ) ) ;
#5029=VECTOR ( 'NONE', #8402, 1000.000000000000000 ) ;
#5033=EDGE_CURVE ( 'NONE', #11588, #16127, #820, .T. ) ;
#5038=CARTESIAN_POINT ( 'NONE',  ( 49.86468353125001585, 24.82187500034139305, 16.20201782572375038 ) ) ;
#5039=CARTESIAN_POINT ( 'NONE',  ( -40.34137639590981905, 23.65937500034139518, -29.30972558990011478 ) ) ;
#5040=CARTESIAN_POINT ( 'NONE',  ( 2.600676159226421000E-13, 31.28125000068279604, -49.99999999999999289 ) ) ;
#5041=CARTESIAN_POINT ( 'NONE',  ( -40.34137639590981905, 33.72187500034139873, -29.30972558990011478 ) ) ;
#5044=CARTESIAN_POINT ( 'NONE',  ( -15.45084971874736368, 32.39999999999999858, 47.55282581475768211 ) ) ;
#5045=CARTESIAN_POINT ( 'NONE',  ( 9.631387414534489405E-15, 38.35937500034139447, 52.43083105670540789 ) ) ;
#5047=CARTESIAN_POINT ( 'NONE',  ( 50.00000000000000000, 47.00000000000000000, -6.123233995736766085E-15 ) ) ;
#5060=CARTESIAN_POINT ( 'NONE',  ( -3.210462471511496205E-15, 41.42187500034140157, -52.43083105670540789 ) ) ;
#5063=CARTESIAN_POINT ( 'NONE',  ( 30.90169943749475578, 30.48125000068279533, 42.53254041760200010 ) ) ;
#5065=CARTESIAN_POINT ( 'NONE',  ( 49.86468353125000164, 36.92187500034140157, -6.106662507704105588E-15 ) ) ;
#5069=VERTEX_POINT ( 'NONE', #9083 ) ;
#5073=CARTESIAN_POINT ( 'NONE',  ( 2.600676159226420495E-13, 23.28125000068279604, -49.99999999999999289 ) ) ;
#5074=CARTESIAN_POINT ( 'NONE',  ( -40.34137639590981195, 30.05937500034139731, 29.30972558990012189 ) ) ;
#5076=CARTESIAN_POINT ( 'NONE',  ( 40.34137639590981195, 47.12187500034140442, -29.30972558990011834 ) ) ;
#5090=CARTESIAN_POINT ( 'NONE',  ( 7.919222016226940219, 33.22999571913595673, -49.99999999999996447 ) ) ;
#5094=( LENGTH_UNIT ( ) NAMED_UNIT ( * ) SI_UNIT ( .MILLI., .METRE. ) );
#5096=CARTESIAN_POINT ( 'NONE',  ( -30.90169943749474868, 47.48125000068279178, -42.53254041760200721 ) ) ;
#5097=CARTESIAN_POINT ( 'NONE',  ( -2.547328955960238000E-13, 20.49999999999999645, 49.99999999999999289 ) ) ;
#5099=CARTESIAN_POINT ( 'NONE',  ( -49.86468353125000164, 19.85937500034139447, 0.000000000000000000 ) ) ;
#5103=CARTESIAN_POINT ( 'NONE',  ( -50.00000000000000000, 49.78125000068280315, 0.000000000000000000 ) ) ;
#5110=CARTESIAN_POINT ( 'NONE',  ( -1.157256219580996337, 39.97118149501703499, 92.94656295785023303 ) ) ;
#5114=CARTESIAN_POINT ( 'NONE',  ( 40.34137639590981195, 25.05937500034139376, -29.30972558990011834 ) ) ;
#5116=CARTESIAN_POINT ( 'NONE',  ( -30.81806926056963292, 37.62187500034138310, -42.41743335407646498 ) ) ;
#5120=CARTESIAN_POINT ( 'NONE',  ( 49.99999999999999289, 29.10000000000000142, -16.24598481164532160 ) ) ;
#5121=CARTESIAN_POINT ( 'NONE',  ( 9.631387414534489405E-15, 36.35937500034140157, 52.43083105670540789 ) ) ;
#5123=EDGE_CURVE ( 'NONE', #12892, #4175, #2334, .T. ) ;
#5124=CARTESIAN_POINT ( 'NONE',  ( -15.45084971874737256, 45.60000000000000142, -47.55282581475767500 ) ) ;
#5125=ORIENTED_EDGE ( 'NONE', *, *, #7557, .T. ) ;
#5136=CARTESIAN_POINT ( 'NONE',  ( 9.631387414534489405E-15, 44.42187500034140157, 52.43083105670540789 ) ) ;
#5139=CARTESIAN_POINT ( 'NONE',  ( 30.90169943749475578, 26.48125000068279888, 42.53254041760200010 ) ) ;
#5141=CARTESIAN_POINT ( 'NONE',  ( 15.40903463028481113, 31.32187500034139305, -47.42413220539094709 ) ) ;
#5148=CARTESIAN_POINT ( 'NONE',  ( -30.90169943749474513, 23.69999999999999929, -42.53254041760200721 ) ) ;
#5150=CARTESIAN_POINT ( 'NONE',  ( 49.86468353125000164, 32.85937500034139447, -6.106662507704105588E-15 ) ) ;
#5151=CARTESIAN_POINT ( 'NONE',  ( 6.123233995736766085E-15, 20.00000000000000355, -50.00000000000000000 ) ) ;
#5152=CARTESIAN_POINT ( 'NONE',  ( -49.86468353125000164, 47.92187500034139447, 0.000000000000000000 ) ) ;
#5161=CARTESIAN_POINT ( 'NONE',  ( -50.00000000000000000, 45.78125000068279604, 0.000000000000000000 ) ) ;
#5169=CARTESIAN_POINT ( 'NONE',  ( 15.45084971874737789, 32.38125000068280457, 47.55282581475767500 ) ) ;
#5173=FILL_AREA_STYLE_COLOUR ( '', #9709 ) ;
#5174=CARTESIAN_POINT ( 'NONE',  ( 1.022488062601840571E-14, 49.50000000000000711, -50.00000000000000000 ) ) ;
#5175=CARTESIAN_POINT ( 'NONE',  ( 40.45084971874737079, 40.98125000068279888, -29.38926261462366440 ) ) ;
#5176=CARTESIAN_POINT ( 'NONE',  ( 2.600676159226420495E-13, 21.50000000000000000, -49.99999999999999289 ) ) ;
#5182=EDGE_LOOP ( 'NONE', ( #14496, #10965, #8865, #15210 ) ) ;
#5184=FACE_OUTER_BOUND ( 'NONE', #14025, .T. ) ;
#5193=CARTESIAN_POINT ( 'NONE',  ( -3.210462471511496205E-15, 23.35937500034139447, -52.43083105670540789 ) ) ;
#5194=DIRECTION ( 'NONE',  ( 0.000000000000000000, 1.000000000000000000, 0.000000000000000000 ) ) ;
#5195=CARTESIAN_POINT ( 'NONE',  ( 49.86468353124999453, 27.02187500034139944, -16.20201782572376104 ) ) ;
#5197=CARTESIAN_POINT ( 'NONE',  ( -50.00000000000000000, 32.00000000000000000, 0.000000000000000000 ) ) ;
#5198=CARTESIAN_POINT ( 'NONE',  ( -49.86468353124999453, 35.75937500034140015, -16.20201782572375393 ) ) ;
#5201=CARTESIAN_POINT ( 'NONE',  ( 50.00000000000000000, 41.00000000000000000, -6.123233995736766085E-15 ) ) ;
#5215=CARTESIAN_POINT ( 'NONE',  ( -15.40903463028481646, 43.52187500034139589, -47.42413220539093999 ) ) ;
#5216=CARTESIAN_POINT ( 'NONE',  ( -30.81806926056963292, 39.55937500034140442, -42.41743335407646498 ) ) ;
#5221=CARTESIAN_POINT ( 'NONE',  ( -50.00000000000000000, 27.78125000068279959, 0.000000000000000000 ) ) ;
#5225=CARTESIAN_POINT ( 'NONE',  ( 49.86468353124999453, 33.02187500034139589, -16.20201782572376459 ) ) ;
#5226=PLANE ( 'NONE',  #3836 ) ;
#5239=CARTESIAN_POINT ( 'NONE',  ( -49.86468353125000164, 33.85937500034139447, 0.000000000000000000 ) ) ;
#5241=CARTESIAN_POINT ( 'NONE',  ( -49.86468353124999453, 43.82187500034140015, -16.20201782572375393 ) ) ;
#5249=VERTEX_POINT ( 'NONE', #15966 ) ;
#5265=CYLINDRICAL_SURFACE ( 'NONE', #10991, 50.00000000000000000 ) ;
#5266=CARTESIAN_POINT ( 'NONE',  ( 15.45084971874737789, 38.38125000068279746, 47.55282581475767500 ) ) ;
#5267=CARTESIAN_POINT ( 'NONE',  ( 0.000000000000000000, 20.00000000000000355, 50.00000000000000000 ) ) ;
#5272=ORIENTED_EDGE ( 'NONE', *, *, #4314, .F. ) ;
#5273=CARTESIAN_POINT ( 'NONE',  ( 50.00000000000000000, 42.78125000068280315, -6.123233995736766085E-15 ) ) ;
#5278=FACE_OUTER_BOUND ( 'NONE', #13417, .T. ) ;
#5283=CARTESIAN_POINT ( 'NONE',  ( 30.81806926056964002, 22.55937500034139020, 42.41743335407646498 ) ) ;
#5285=CARTESIAN_POINT ( 'NONE',  ( 30.81806926056964002, 28.62187500034139731, 42.41743335407646498 ) ) ;
#5287=CARTESIAN_POINT ( 'NONE',  ( 9.657523855033129090E-15, 28.49999999999999645, 52.57311121191334990 ) ) ;
#5288=CARTESIAN_POINT ( 'NONE',  ( 9.631387414534489405E-15, 34.35937500034139447, 52.43083105670540789 ) ) ;
#5294=EDGE_CURVE ( 'NONE', #12450, #16417, #2220, .T. ) ;
#5302=CARTESIAN_POINT ( 'NONE',  ( -40.34137639590981195, 38.12187500034139731, 29.30972558990012189 ) ) ;
#5303=CARTESIAN_POINT ( 'NONE',  ( -30.81806926056962226, 40.15937500034139163, 42.41743335407647209 ) ) ;
#5306=CARTESIAN_POINT ( 'NONE',  ( -49.99999999999999289, 21.68125000068280173, -16.24598481164531449 ) ) ;
#5307=EDGE_CURVE ( 'NONE', #6137, #13242, #2964, .T. ) ;
#5309=CARTESIAN_POINT ( 'NONE',  ( 15.40903463028482356, 26.52187500034139589, 47.42413220539093999 ) ) ;
#5310=CARTESIAN_POINT ( 'NONE',  ( 8.446640517145639571E-15, 28.28125000068279959, 50.00000000000000000 ) ) ;
#5319=CARTESIAN_POINT ( 'NONE',  ( 15.40903463028482356, 26.45937500034139589, 47.42413220539093999 ) ) ;
#5322=CARTESIAN_POINT ( 'NONE',  ( -15.40903463028481646, 45.52187500034139589, -47.42413220539093999 ) ) ;
#5326=CYLINDRICAL_SURFACE ( 'NONE', #1441, 50.00000000000000000 ) ;
#5327=CARTESIAN_POINT ( 'NONE',  ( 30.81806926056962936, 47.22187500034139873, -42.41743335407647209 ) ) ;
#5339=CARTESIAN_POINT ( 'NONE',  ( -30.90169943749474868, 21.69999999999999574, -42.53254041760200721 ) ) ;
#5340=CARTESIAN_POINT ( 'NONE',  ( -15.40903463028481646, 49.45937500034140299, -47.42413220539093999 ) ) ;
#5341=CARTESIAN_POINT ( 'NONE',  ( -40.45084971874737079, 31.98125000068280244, 29.38926261462367151 ) ) ;
#5343=CARTESIAN_POINT ( 'NONE',  ( -30.81806926056962226, 24.22187500034139163, 42.41743335407647919 ) ) ;
#5345=CARTESIAN_POINT ( 'NONE',  ( 30.90169943749475578, 42.48125000068279888, 42.53254041760200010 ) ) ;
#5352=CARTESIAN_POINT ( 'NONE',  ( 30.90169943749475223, 42.69999999999999574, 42.53254041760199300 ) ) ;
#5363=CARTESIAN_POINT ( 'NONE',  ( -46.91068958262638944, 20.00000000000000355, 16.90862634959490407 ) ) ;
#5364=CARTESIAN_POINT ( 'NONE',  ( 49.86468353125001585, 26.82187500034139305, 16.20201782572375038 ) ) ;
#5366=CARTESIAN_POINT ( 'NONE',  ( -49.99999999999999289, 32.10000000000000142, 16.24598481164533226 ) ) ;
#5367=CARTESIAN_POINT ( 'NONE',  ( -40.34137639590981195, 34.05937500034139731, 29.30972558990012189 ) ) ;
#5379=CARTESIAN_POINT ( 'NONE',  ( -49.86468353124999453, 33.82187500034138594, -16.20201782572375393 ) ) ;
#5380=CARTESIAN_POINT ( 'NONE',  ( -49.86468353124999453, 43.75937500034140015, -16.20201782572375393 ) ) ;
#5383=CARTESIAN_POINT ( 'NONE',  ( -15.45084971874736368, 22.18125000068279817, 47.55282581475768211 ) ) ;
#5384=CARTESIAN_POINT ( 'NONE',  ( 40.34137639590981195, 29.12187500034139376, -29.30972558990011834 ) ) ;
#5392=CARTESIAN_POINT ( 'NONE',  ( -15.40903463028480580, 22.25937500034139660, 47.42413220539094709 ) ) ;
#5394=CARTESIAN_POINT ( 'NONE',  ( -30.81806926056962226, 40.22187500034139873, 42.41743335407647209 ) ) ;
#5397=CARTESIAN_POINT ( 'NONE',  ( 40.34137639590981195, 47.12187500034140442, -29.30972558990011834 ) ) ;
#5407=CARTESIAN_POINT ( 'NONE',  ( -3.111920190527341144E-15, 43.28125000068280315, -50.00000000000000000 ) ) ;
#5408=CARTESIAN_POINT ( 'NONE',  ( 15.45084971874736723, 39.18125000068280173, -47.55282581475768211 ) ) ;
#5410=EDGE_CURVE ( 'NONE', #7762, #15191, #9905, .T. ) ;
#5411=CARTESIAN_POINT ( 'NONE',  ( -15.45084971874737256, 27.60000000000000142, -47.55282581475767500 ) ) ;
#5412=CARTESIAN_POINT ( 'NONE',  ( -15.40903463028480580, 42.25937500034139305, 47.42413220539094709 ) ) ;
#5414=AXIS2_PLACEMENT_3D ( 'NONE', #7993, #13144, #15554 ) ;
#5415=CARTESIAN_POINT ( 'NONE',  ( -30.81806926056963292, 21.62187500034139376, -42.41743335407647209 ) ) ;
#5418=CARTESIAN_POINT ( 'NONE',  ( -30.90169943749474868, 41.48125000068278467, -42.53254041760200721 ) ) ;
#5438=CARTESIAN_POINT ( 'NONE',  ( -47.60088917010773457, 20.00000000000000355, 14.85495851097764231 ) ) ;
#5439=CARTESIAN_POINT ( 'NONE',  ( -49.86468353124999453, 26.02187500034139589, 16.20201782572377169 ) ) ;
#5443=CARTESIAN_POINT ( 'NONE',  ( 40.34137639590981195, 31.05937500034139731, -29.30972558990011834 ) ) ;
#5451=VECTOR ( 'NONE', #11154, 1000.000000000000000 ) ;
#5452=DIRECTION ( 'NONE',  ( 0.000000000000000000, 0.000000000000000000, 1.000000000000000000 ) ) ;
#5455=CARTESIAN_POINT ( 'NONE',  ( 40.34137639590981195, 33.12187500034139731, -29.30972558990011834 ) ) ;
#5456=CARTESIAN_POINT ( 'NONE',  ( 30.81806926056962936, 37.15937500034139163, -42.41743335407646498 ) ) ;
#5461=CARTESIAN_POINT ( 'NONE',  ( 9.657523855033129090E-15, 22.28125000068279959, 52.57311121191334990 ) ) ;
#5464=CARTESIAN_POINT ( 'NONE',  ( -49.86468353124999453, 27.82187500034139305, -16.20201782572375393 ) ) ;
#5474=CARTESIAN_POINT ( 'NONE',  ( -30.81806926056963292, 25.55937500034139376, -42.41743335407647209 ) ) ;
#5476=CARTESIAN_POINT ( 'NONE',  ( -49.86468353125000164, 39.92187500034139447, 0.000000000000000000 ) ) ;
#5479=CARTESIAN_POINT ( 'NONE',  ( 40.34137639590981195, 45.12187500034139731, -29.30972558990011834 ) ) ;
#5485=ORIENTED_EDGE ( 'NONE', *, *, #9175, .T. ) ;
#5486=CARTESIAN_POINT ( 'NONE',  ( -7.919222016226816763, 45.33250428222963535, -49.99999999999999289 ) ) ;
#5487=EDGE_LOOP ( 'NONE', ( #15628, #3760, #6506, #2705 ) ) ;
#5490=ADVANCED_FACE ( 'NONE', ( #3584 ), #217, .F. ) ;
#5492=DIRECTION ( 'NONE',  ( -0.000000000000000000, 1.000000000000000000, -0.000000000000000000 ) ) ;
#5494=CARTESIAN_POINT ( 'NONE',  ( -15.45084971874737256, 23.60000000000000142, -47.55282581475767500 ) ) ;
#5496=CARTESIAN_POINT ( 'NONE',  ( -49.86468353125000164, 43.85937500034140157, 0.000000000000000000 ) ) ;
#5505=CARTESIAN_POINT ( 'NONE',  ( -50.00000000000000000, 39.78125000068279604, 0.000000000000000000 ) ) ;
#5507=CARTESIAN_POINT ( 'NONE',  ( 15.45084971874737789, 46.38125000068279746, 47.55282581475767500 ) ) ;
#5514=AXIS2_PLACEMENT_3D ( 'NONE', #15634, #4259, #9325 ) ;
#5516=LINE ( 'NONE', #9246, #6842 ) ;
#5524=CARTESIAN_POINT ( 'NONE',  ( -49.99999999999999289, 37.88125000068279746, 16.24598481164533226 ) ) ;
#5526=DIRECTION ( 'NONE',  ( -0.000000000000000000, -1.000000000000000000, -0.000000000000000000 ) ) ;
#5527=CARTESIAN_POINT ( 'NONE',  ( -46.62157290631127893, 20.00000000000001066, 17.69020581817094850 ) ) ;
#5528=CARTESIAN_POINT ( 'NONE',  ( 40.34137639590981195, 29.12187500034139376, -29.30972558990011834 ) ) ;
#5530=CARTESIAN_POINT ( 'NONE',  ( -30.90169943749474513, 21.69999999999999574, -42.53254041760200721 ) ) ;
#5532=CARTESIAN_POINT ( 'NONE',  ( 30.81806926056964002, 30.55937500034139731, 42.41743335407647209 ) ) ;
#5542=CARTESIAN_POINT ( 'NONE',  ( -40.45084971874737079, 38.20000000000000284, 29.38926261462367151 ) ) ;
#5545=CARTESIAN_POINT ( 'NONE',  ( 49.86468353125000164, 38.92187500034139447, -6.106662507704105588E-15 ) ) ;
#5546=CARTESIAN_POINT ( 'NONE',  ( -49.86468353124999453, 35.95937500034139589, 16.20201782572377169 ) ) ;
#5549=CARTESIAN_POINT ( 'NONE',  ( 30.81806926056964002, 48.55937500034138310, 42.41743335407647209 ) ) ;
#5551=CARTESIAN_POINT ( 'NONE',  ( 49.86468353125000164, 24.92187500034139802, -6.106662507704105588E-15 ) ) ;
#5553=CARTESIAN_POINT ( 'NONE',  ( -3.111920190527341144E-15, 27.28125000068279604, -50.00000000000000000 ) ) ;
#5554=ORIENTED_EDGE ( 'NONE', *, *, #787, .T. ) ;
#5561=CARTESIAN_POINT ( 'NONE',  ( 50.00000000000000711, 30.68125000068279462, 16.24598481164530739 ) ) ;
#5563=CARTESIAN_POINT ( 'NONE',  ( 15.40903463028481113, 27.25937500034139660, -47.42413220539094709 ) ) ;
#5565=CARTESIAN_POINT ( 'NONE',  ( -15.40903463028481646, 41.52187500034139589, -47.42413220539093999 ) ) ;
#5568=CARTESIAN_POINT ( 'NONE',  ( -49.86468353125000164, 43.92187500034140157, 0.000000000000000000 ) ) ;
#5578=CARTESIAN_POINT ( 'NONE',  ( 30.90169943749474157, 23.29999999999999716, -42.53254041760200721 ) ) ;
#5579=CARTESIAN_POINT ( 'NONE',  ( 15.40903463028481113, 45.25937500034140015, -47.42413220539094709 ) ) ;
#5580=CARTESIAN_POINT ( 'NONE',  ( -15.45084971874736368, 32.18125000068279462, 47.55282581475768211 ) ) ;
#5583=CARTESIAN_POINT ( 'NONE',  ( 50.00000000000000000, 36.78125000068280315, -6.123233995736766085E-15 ) ) ;
#5585=CARTESIAN_POINT ( 'NONE',  ( 30.90169943749475223, 20.48125000068279178, 42.53254041760199300 ) ) ;
#5587=ORIENTED_EDGE ( 'NONE', *, *, #13322, .T. ) ;
#5590=ORIENTED_EDGE ( 'NONE', *, *, #16177, .F. ) ;
#5591=ORIENTED_EDGE ( 'NONE', *, *, #2216, .F. ) ;
#5595=EDGE_LOOP ( 'NONE', ( #5590, #6125, #9604, #9587 ) ) ;
#5597=CARTESIAN_POINT ( 'NONE',  ( 7.919222016226940219, 23.44874571845315359, -49.99999999999996447 ) ) ;
#5601=CARTESIAN_POINT ( 'NONE',  ( 8.446640517145639571E-15, 26.50000000000000000, 50.00000000000000000 ) ) ;
#5602=CARTESIAN_POINT ( 'NONE',  ( -49.86468353124999453, 22.02187500034139589, 16.20201782572377169 ) ) ;
#5605=CARTESIAN_POINT ( 'NONE',  ( 49.86468353125001585, 34.75937500034139305, 16.20201782572375038 ) ) ;
#5607=VERTEX_POINT ( 'NONE', #4305 ) ;
#5617=CARTESIAN_POINT ( 'NONE',  ( -30.81806926056963292, 37.62187500034139020, -42.41743335407647209 ) ) ;
#5618=CARTESIAN_POINT ( 'NONE',  ( 15.40903463028481113, 37.25937500034140015, -47.42413220539094709 ) ) ;
#5623=CARTESIAN_POINT ( 'NONE',  ( -40.45084971874737789, 21.58125000068279675, -29.38926261462365730 ) ) ;
#5625=CARTESIAN_POINT ( 'NONE',  ( -30.81806926056962226, 30.22187500034139518, 42.41743335407647919 ) ) ;
#5633=CARTESIAN_POINT ( 'NONE',  ( -15.40903463028481646, 25.45937500034139589, -47.42413220539093999 ) ) ;
#5635=CARTESIAN_POINT ( 'NONE',  ( -30.81806926056962226, 44.22187500034139163, 42.41743335407647919 ) ) ;
#5639=ORIENTED_EDGE ( 'NONE', *, *, #12767, .T. ) ;
#5644=CARTESIAN_POINT ( 'NONE',  ( 40.45084971874737079, 38.98125000068279888, -29.38926261462366440 ) ) ;
#5645=CARTESIAN_POINT ( 'NONE',  ( 6.123233995736766085E-15, 20.00000000000000355, -50.00000000000000000 ) ) ;
#5646=CARTESIAN_POINT ( 'NONE',  ( -30.90169943749473802, 24.29999999999999716, 42.53254041760200721 ) ) ;
#5647=CARTESIAN_POINT ( 'NONE',  ( -40.34137639590981195, 46.05937500034139731, 29.30972558990012189 ) ) ;
#5659=ORIENTED_EDGE ( 'NONE', *, *, #7269, .T. ) ;
#5662=CARTESIAN_POINT ( 'NONE',  ( 7.513064459987437071E-14, 42.50000000000000000, 50.00000000000000000 ) ) ;
#5672=CARTESIAN_POINT ( 'NONE',  ( 16.94295052416147840, 17.97534012751635402, 95.33699471030656980 ) ) ;
#5674=CARTESIAN_POINT ( 'NONE',  ( 40.34137639590981905, 20.72187500034139873, 29.30972558990010768 ) ) ;
#5677=CARTESIAN_POINT ( 'NONE',  ( 49.86468353124999453, 24.95937500034139234, -16.20201782572376459 ) ) ;
#5679=CARTESIAN_POINT ( 'NONE',  ( -2.547328955960238000E-13, 30.49999999999999645, 49.99999999999999289 ) ) ;
#5680=ORIENTED_EDGE ( 'NONE', *, *, #2226, .T. ) ;
#5690=CARTESIAN_POINT ( 'NONE',  ( 40.34137639590981195, 29.12187500034139376, -29.30972558990011834 ) ) ;
#5691=CARTESIAN_POINT ( 'NONE',  ( -15.40903463028480580, 38.25937500034140015, 47.42413220539094709 ) ) ;
#5695=CARTESIAN_POINT ( 'NONE',  ( 30.81806926056962936, 47.15937500034138452, -42.41743335407647209 ) ) ;
#5697=CARTESIAN_POINT ( 'NONE',  ( 50.00000000000000000, 49.00000000000000000, -6.123233995736766085E-15 ) ) ;
#5706=ORIENTED_EDGE ( 'NONE', *, *, #6252, .T. ) ;
#5709=CARTESIAN_POINT ( 'NONE',  ( 30.90169943749475223, 30.48125000068279533, 42.53254041760199300 ) ) ;
#5711=CARTESIAN_POINT ( 'NONE',  ( 9.631387414534489405E-15, 20.35937500034139092, 52.43083105670540789 ) ) ;
#5715=CARTESIAN_POINT ( 'NONE',  ( 15.45084971874737789, 36.60000000000000142, 47.55282581475767500 ) ) ;
#5716=CARTESIAN_POINT ( 'NONE',  ( -49.86468353124999453, 42.02187500034139589, 16.20201782572377525 ) ) ;
#5717=CARTESIAN_POINT ( 'NONE',  ( 40.45084971874737079, 31.20000000000000284, -29.38926261462366440 ) ) ;
#5718=ORIENTED_EDGE ( 'NONE', *, *, #3167, .T. ) ;
#5724=CARTESIAN_POINT ( 'NONE',  ( -30.90169943749474513, 39.48125000068278467, -42.53254041760200721 ) ) ;
#5727=CARTESIAN_POINT ( 'NONE',  ( 1.293669679204937499E-13, 37.28125000068280315, -50.00000000000000000 ) ) ;
#5728=CARTESIAN_POINT ( 'NONE',  ( 40.34137639590981195, 43.05937500034139731, -29.30972558990011834 ) ) ;
#5729=CARTESIAN_POINT ( 'NONE',  ( -49.86468353125000164, 47.85937500034139447, 0.000000000000000000 ) ) ;
#5731=ADVANCED_FACE ( 'NONE', ( #3631 ), #14913, .F. ) ;
#5732=DIRECTION ( 'NONE',  ( -0.8660254037844320463, 0.5000000000000113243, 0.000000000000000000 ) ) ;
#5734=LINE ( 'NONE', #15869, #9670 ) ;
#5737=ORIENTED_EDGE ( 'NONE', *, *, #13228, .T. ) ;
#5738=( BOUNDED_CURVE ( )  B_SPLINE_CURVE ( 2, ( #10799, #3393, #14846, #2206, #3475, #964, #14673, #7302, #13523, #5724, #13358, #8531, #15860 ),
 .UNSPECIFIED., .F., .F. ) 
 B_SPLINE_CURVE_WITH_KNOTS ( ( 3, 2, 2, 2, 2, 2, 3 ),
 ( 0.3166666666666667074, 0.3200000000000000067, 0.3266666666666666607, 0.3333333333333333148, 0.3400000000000000244, 0.3466666666666666785, 0.3500000000000000333 ),
 .UNSPECIFIED. ) 
 CURVE ( )  GEOMETRIC_REPRESENTATION_ITEM ( )  RATIONAL_B_SPLINE_CURVE ( ( 0.9755282581475768211, 0.9755282581475770431, 1.000000000000000000, 0.9510565162951535312, 1.000000000000000000, 0.9510565162951535312, 1.000000000000000000, 0.9510565162951535312, 1.000000000000000000, 0.9510565162951535312, 1.000000000000000000, 0.9755282581475765991, 0.9755282581475768211 ) ) 
 REPRESENTATION_ITEM ( '' )  );
#5740=ORIENTED_EDGE ( 'NONE', *, *, #3374, .F. ) ;
#5742=ORIENTED_EDGE ( 'NONE', *, *, #1414, .F. ) ;
#5751=ORIENTED_EDGE ( 'NONE', *, *, #5909, .F. ) ;
#5752=DIRECTION ( 'NONE',  ( -0.000000000000000000, 1.000000000000000000, -0.000000000000000000 ) ) ;
#5757=CARTESIAN_POINT ( 'NONE',  ( -15.45084971874736368, 48.40000000000000568, 47.55282581475768211 ) ) ;
#5760=CARTESIAN_POINT ( 'NONE',  ( -49.86468353125000164, 21.92187500034139802, 0.000000000000000000 ) ) ;
#5763=CARTESIAN_POINT ( 'NONE',  ( -49.86468353124999453, 25.95937500034139944, 16.20201782572377525 ) ) ;
#5774=CARTESIAN_POINT ( 'NONE',  ( 30.90169943749473802, 29.08125000068280031, -42.53254041760200721 ) ) ;
#5777=CARTESIAN_POINT ( 'NONE',  ( 40.34137639590981905, 26.72187500034139518, 29.30972558990010768 ) ) ;
#5778=CARTESIAN_POINT ( 'NONE',  ( -49.86468353125000164, 33.85937500034139447, 0.000000000000000000 ) ) ;
#5779=CARTESIAN_POINT ( 'NONE',  ( 7.919222016226822092, 26.33250428222964246, 49.99999999999999289 ) ) ;
#5781=CARTESIAN_POINT ( 'NONE',  ( -15.40903463028480580, 42.25937500034139305, 47.42413220539094709 ) ) ;
#5783=CARTESIAN_POINT ( 'NONE',  ( -40.34137639590981195, 22.12187500034139731, 29.30972558990012189 ) ) ;
#5784=ORIENTED_EDGE ( 'NONE', *, *, #1565, .F. ) ;
#5790=CARTESIAN_POINT ( 'NONE',  ( 30.90169943749473802, 41.08125000068280031, -42.53254041760200721 ) ) ;
#5792=CARTESIAN_POINT ( 'NONE',  ( -15.40903463028480580, 46.32187500034140015, 47.42413220539094709 ) ) ;
#5795=CARTESIAN_POINT ( 'NONE',  ( -49.99999999999999289, 39.90000000000001279, -16.24598481164531449 ) ) ;
#5796=CARTESIAN_POINT ( 'NONE',  ( -40.34137639590981195, 38.12187500034139731, 29.30972558990012189 ) ) ;
#5801=EDGE_LOOP ( 'NONE', ( #5706, #10303, #2939, #5740 ) ) ;
#5803=( BOUNDED_CURVE ( )  B_SPLINE_CURVE ( 2, ( #10954, #13526, #3395, #1045, #16019, #3304, #16193, #7142, #7218, #8611, #4647, #7389, #9877 ),
 .UNSPECIFIED., .F., .F. ) 
 B_SPLINE_CURVE_WITH_KNOTS ( ( 3, 2, 2, 2, 2, 2, 3 ),
 ( 0.7500000000000000000, 0.7533333333333332993, 0.7600000000000000089, 0.7666666666666667185, 0.7733333333333333171, 0.7800000000000000266, 0.7833333333333333259 ),
 .UNSPECIFIED. ) 
 CURVE ( )  GEOMETRIC_REPRESENTATION_ITEM ( )  RATIONAL_B_SPLINE_CURVE ( ( 0.9755282581475768211, 0.9755282581475768211, 1.000000000000000000, 0.9510565162951535312, 1.000000000000000000, 0.9510565162951535312, 1.000000000000000000, 0.9510565162951535312, 1.000000000000000000, 0.9510565162951535312, 1.000000000000000000, 0.9755282581475768211, 0.9755282581475768211 ) ) 
 REPRESENTATION_ITEM ( '' )  );
#5808=CARTESIAN_POINT ( 'NONE',  ( 7.919222016226758143, 36.33250428222963535, 50.00000000000000711 ) ) ;
#5809=EDGE_CURVE ( 'NONE', #15952, #12012, #7375, .T. ) ;
#5810=CARTESIAN_POINT ( 'NONE',  ( -40.34137639590981195, 38.05937500034139731, 29.30972558990012189 ) ) ;
#5821=EDGE_LOOP ( 'NONE', ( #14608, #3533, #535, #8328 ) ) ;
#5829=CARTESIAN_POINT ( 'NONE',  ( 30.90169943749473802, 29.30000000000000071, -42.53254041760200721 ) ) ;
#5833=CARTESIAN_POINT ( 'NONE',  ( -13.21840623068678866, 11.01752607032678455, 97.16300551537720764 ) ) ;
#5839=CARTESIAN_POINT ( 'NONE',  ( -41.19975849074612029, 20.00000000000000355, 28.55207485309411553 ) ) ;
#5840=EDGE_CURVE ( 'NONE', #5867, #16127, #8444, .T. ) ;
#5841=CARTESIAN_POINT ( 'NONE',  ( -48.35726954556750457, 20.00000000000000355, 12.16803787670978387 ) ) ;
#5844=AXIS2_PLACEMENT_3D ( 'NONE', #10225, #15277, #5012 ) ;
#5846=CARTESIAN_POINT ( 'NONE',  ( 15.40903463028482356, 26.45937500034139589, 47.42413220539093999 ) ) ;
#5848=CARTESIAN_POINT ( 'NONE',  ( -15.45084971874737256, 29.60000000000000142, -47.55282581475767500 ) ) ;
#5854=CARTESIAN_POINT ( 'NONE',  ( 7.919222016226822092, 48.33250428222964246, 49.99999999999999289 ) ) ;
#5857=CARTESIAN_POINT ( 'NONE',  ( 49.86468353124999453, 31.02187500034139234, -16.20201782572376459 ) ) ;
#5858=CARTESIAN_POINT ( 'NONE',  ( 49.86468353125001585, 26.75937500034139660, 16.20201782572375038 ) ) ;
#5862=CARTESIAN_POINT ( 'NONE',  ( -49.86468353125000164, 45.85937500034140157, 0.000000000000000000 ) ) ;
#5865=CARTESIAN_POINT ( 'NONE',  ( 49.86468353124999453, 23.02187500034139944, -16.20201782572376459 ) ) ;
#5867=VERTEX_POINT ( 'NONE', #6535 ) ;
#5873=CARTESIAN_POINT ( 'NONE',  ( 2.600676159226420495E-13, 33.28125000068279604, -49.99999999999999289 ) ) ;
#5875=CARTESIAN_POINT ( 'NONE',  ( -40.34137639590981905, 47.72187500034139873, -29.30972558990011478 ) ) ;
#5879=CARTESIAN_POINT ( 'NONE',  ( 40.45084971874737789, 32.58125000068280031, 29.38926261462365375 ) ) ;
#5880=CARTESIAN_POINT ( 'NONE',  ( -49.99999999999999289, 35.90000000000000568, -16.24598481164531449 ) ) ;
#5881=CARTESIAN_POINT ( 'NONE',  ( -40.34137639590981195, 42.12187500034139731, 29.30972558990012189 ) ) ;
#5891=CARTESIAN_POINT ( 'NONE',  ( -15.45084971874737256, 21.38125000068279746, -47.55282581475767500 ) ) ;
#5893=CARTESIAN_POINT ( 'NONE',  ( 15.40903463028481113, 39.25937500034140015, -47.42413220539094709 ) ) ;
#5895=CARTESIAN_POINT ( 'NONE',  ( 15.45084971874736723, 25.40000000000000213, -47.55282581475768211 ) ) ;
#5898=CARTESIAN_POINT ( 'NONE',  ( 0.000000000000000000, 20.00000000000000355, 50.00000000000000000 ) ) ;
#5909=EDGE_CURVE ( 'NONE', #8741, #12025, #11601, .T. ) ;
#5917=CARTESIAN_POINT ( 'NONE',  ( -4.611208113858000779, 5.578466101304616842, 98.91552298129929000 ) ) ;
#5923=LINE ( 'NONE', #14624, #11510 ) ;
#5925=CARTESIAN_POINT ( 'NONE',  ( 49.86468353125000164, 22.92187500034139802, -6.106662507704105588E-15 ) ) ;
#5929=CARTESIAN_POINT ( 'NONE',  ( -49.86468353124999453, 27.75937500034139660, -16.20201782572375393 ) ) ;
#5930=CARTESIAN_POINT ( 'NONE',  ( -40.45084971874737079, 30.20000000000000284, 29.38926261462367151 ) ) ;
#5934=ORIENTED_EDGE ( 'NONE', *, *, #3167, .F. ) ;
#5935=DIRECTION ( 'NONE',  ( -0.000000000000000000, 1.000000000000000000, -0.000000000000000000 ) ) ;
#5939=( BOUNDED_CURVE ( )  B_SPLINE_CURVE ( 2, ( #2414, #4684, #3432, #7419, #11081, #16390, #4855, #16054, #14883, #8566, #7256, #13636, #12488 ),
 .UNSPECIFIED., .F., .F. ) 
 B_SPLINE_CURVE_WITH_KNOTS ( ( 3, 2, 2, 2, 2, 2, 3 ),
 ( 0.2500000000000000000, 0.2533333333333333548, 0.2600000000000000089, 0.2666666666666666630, 0.2733333333333333171, 0.2800000000000000266, 0.2833333333333333814 ),
 .UNSPECIFIED. ) 
 CURVE ( )  GEOMETRIC_REPRESENTATION_ITEM ( )  RATIONAL_B_SPLINE_CURVE ( ( 0.9755282581475765991, 0.9755282581475765991, 1.000000000000000000, 0.9510565162951535312, 1.000000000000000000, 0.9510565162951535312, 1.000000000000000000, 0.9510565162951535312, 1.000000000000000000, 0.9510565162951535312, 1.000000000000000000, 0.9755282581475765991, 0.9755282581475768211 ) ) 
 REPRESENTATION_ITEM ( '' )  );
#5941=CARTESIAN_POINT ( 'NONE',  ( -15.40903463028480580, 30.32187500034140015, 47.42413220539094709 ) ) ;
#5942=CARTESIAN_POINT ( 'NONE',  ( -40.34137639590981195, 32.05937500034139731, 29.30972558990012189 ) ) ;
#5948=CARTESIAN_POINT ( 'NONE',  ( 49.86468353125001585, 44.75937500034138594, 16.20201782572375038 ) ) ;
#5950=CARTESIAN_POINT ( 'NONE',  ( -49.86468353125000164, 23.92187500034139447, 0.000000000000000000 ) ) ;
#5957=CARTESIAN_POINT ( 'NONE',  ( 50.00000000000000000, 40.78125000068279604, -6.123233995736766085E-15 ) ) ;
#5960=CARTESIAN_POINT ( 'NONE',  ( -30.81806926056963292, 49.62187500034139020, -42.41743335407647209 ) ) ;
#5963=CARTESIAN_POINT ( 'NONE',  ( -50.00000000000000000, 31.78125000068279959, 0.000000000000000000 ) ) ;
#5965=CARTESIAN_POINT ( 'NONE',  ( -40.34137639590981195, 40.12187500034139731, 29.30972558990012189 ) ) ;
#5975=CARTESIAN_POINT ( 'NONE',  ( 15.45084971874736723, 21.40000000000000213, -47.55282581475768211 ) ) ;
#5976=CARTESIAN_POINT ( 'NONE',  ( -40.34137639590981905, 35.65937500034139873, -29.30972558990011478 ) ) ;
#5977=CARTESIAN_POINT ( 'NONE',  ( 15.40903463028481113, 49.25937500034139305, -47.42413220539094709 ) ) ;
#5984=CARTESIAN_POINT ( 'NONE',  ( -40.45084971874737079, 42.20000000000000284, 29.38926261462367151 ) ) ;
#5985=ORIENTED_EDGE ( 'NONE', *, *, #8173, .F. ) ;
#5996=CARTESIAN_POINT ( 'NONE',  ( -50.00000000000000000, 47.78125000068279604, 0.000000000000000000 ) ) ;
#5998=CARTESIAN_POINT ( 'NONE',  ( -2.319115541017227944, 5.144547910235605315, 99.06743674540427946 ) ) ;
#6003=CARTESIAN_POINT ( 'NONE',  ( 2.978552182361884590E-14, 47.50000000000000711, -50.00000000000000000 ) ) ;
#6007=CARTESIAN_POINT ( 'NONE',  ( 50.00000000000000711, 48.68125000068279462, 16.24598481164530739 ) ) ;
#6010=CARTESIAN_POINT ( 'NONE',  ( -15.40903463028481646, 25.45937500034139589, -47.42413220539093999 ) ) ;
#6026=CARTESIAN_POINT ( 'NONE',  ( -40.34137639590981905, 27.72187500034139873, -29.30972558990011478 ) ) ;
#6027=CARTESIAN_POINT ( 'NONE',  ( -49.86468353124999453, 27.75937500034139660, -16.20201782572375393 ) ) ;
#6031=CYLINDRICAL_SURFACE ( 'NONE', #6546, 50.00000000000000000 ) ;
#6032=CARTESIAN_POINT ( 'NONE',  ( -3.210462471511496205E-15, 45.35937500034139447, -52.43083105670540789 ) ) ;
#6034=EDGE_CURVE ( 'NONE', #7298, #11268, #14323, .T. ) ;
#6035=CARTESIAN_POINT ( 'NONE',  ( -40.34137639590981195, 24.12187500034139731, 29.30972558990012189 ) ) ;
#6043=CARTESIAN_POINT ( 'NONE',  ( -40.45084971874737789, 33.58125000068280031, -29.38926261462365730 ) ) ;
#6045=CARTESIAN_POINT ( 'NONE',  ( -3.210462471511496205E-15, 21.35937500034139092, -52.43083105670540789 ) ) ;
#6049=CARTESIAN_POINT ( 'NONE',  ( -15.45084971874737256, 31.38125000068280102, -47.55282581475767500 ) ) ;
#6052=CARTESIAN_POINT ( 'NONE',  ( 49.86468353125001585, 38.82187500034140015, 16.20201782572375038 ) ) ;
#6060=ORIENTED_EDGE ( 'NONE', *, *, #10406, .F. ) ;
#6063=CARTESIAN_POINT ( 'NONE',  ( -49.99999999999999289, 21.68125000068280528, -16.24598481164531449 ) ) ;
#6064=CARTESIAN_POINT ( 'NONE',  ( 30.90169943749474157, 21.30000000000000426, -42.53254041760200721 ) ) ;
#6065=CARTESIAN_POINT ( 'NONE',  ( 49.86468353125000164, 38.85937500034139447, -6.106662507704105588E-15 ) ) ;
#6066=CARTESIAN_POINT ( 'NONE',  ( 40.34137639590981905, 42.65937500034139873, 29.30972558990010768 ) ) ;
#6069=CARTESIAN_POINT ( 'NONE',  ( -30.81806926056963292, 49.62187500034139020, -42.41743335407646498 ) ) ;
#6073=AXIS2_PLACEMENT_3D ( 'NONE', #11531, #10299, #12537 ) ;
#6074=CARTESIAN_POINT ( 'NONE',  ( 30.90169943749473802, 41.30000000000000426, -42.53254041760200721 ) ) ;
#6083=CARTESIAN_POINT ( 'NONE',  ( -40.45084971874737079, 40.20000000000000284, 29.38926261462367151 ) ) ;
#6084=SURFACE_SIDE_STYLE ('',( #2320 ) ) ;
#6088=CARTESIAN_POINT ( 'NONE',  ( -5.711110298752863024, 5.918106549715473008, 98.79732775862568417 ) ) ;
#6090=DIRECTION ( 'NONE',  ( -0.000000000000000000, 1.000000000000000000, -0.000000000000000000 ) ) ;
#6096=CARTESIAN_POINT ( 'NONE',  ( -40.45084971874737789, 45.58125000068280031, -29.38926261462365730 ) ) ;
#6101=VERTEX_POINT ( 'NONE', #1694 ) ;
#6102=CARTESIAN_POINT ( 'NONE',  ( 50.00000000000000711, 44.90000000000000568, 16.24598481164530739 ) ) ;
#6106=CARTESIAN_POINT ( 'NONE',  ( -2.547328955960238000E-13, 20.28125000068279959, 49.99999999999999289 ) ) ;
#6110=CARTESIAN_POINT ( 'NONE',  ( 40.34137639590981905, 20.72187500034139873, 29.30972558990010768 ) ) ;
#6111=CARTESIAN_POINT ( 'NONE',  ( 40.34137639590981195, 27.05937500034139731, -29.30972558990011834 ) ) ;
#6112=CARTESIAN_POINT ( 'NONE',  ( 50.00000000000000000, 26.78125000068279959, -6.123233995736766085E-15 ) ) ;
#6113=CARTESIAN_POINT ( 'NONE',  ( 49.86468353125001585, 36.82187500034140015, 16.20201782572375038 ) ) ;
#6115=CARTESIAN_POINT ( 'NONE',  ( -15.40903463028480580, 40.25937500034139305, 47.42413220539094709 ) ) ;
#6118=CARTESIAN_POINT ( 'NONE',  ( 40.45084971874737079, 43.20000000000000284, -29.38926261462366440 ) ) ;
#6119=ORIENTED_EDGE ( 'NONE', *, *, #1740, .F. ) ;
#6125=ORIENTED_EDGE ( 'NONE', *, *, #3967, .T. ) ;
#6126=CARTESIAN_POINT ( 'NONE',  ( 15.45084971874736723, 41.18125000068280173, -47.55282581475768211 ) ) ;
#6128=CARTESIAN_POINT ( 'NONE',  ( 49.86468353125001585, 44.82187500034138594, 16.20201782572375038 ) ) ;
#6131=CARTESIAN_POINT ( 'NONE',  ( 49.99999999999999289, 34.88125000068279746, -16.24598481164532160 ) ) ;
#6132=CARTESIAN_POINT ( 'NONE',  ( -40.34137639590981905, 35.72187500034139163, -29.30972558990011478 ) ) ;
#6137=VERTEX_POINT ( 'NONE', #10760 ) ;
#6138=ORIENTED_EDGE ( 'NONE', *, *, #1732, .T. ) ;
#6141=CARTESIAN_POINT ( 'NONE',  ( -49.99999999999999289, 21.88125000068279746, 16.24598481164533226 ) ) ;
#6143=CARTESIAN_POINT ( 'NONE',  ( 49.86468353125001585, 36.75937500034138594, 16.20201782572375038 ) ) ;
#6144=CARTESIAN_POINT ( 'NONE',  ( 15.40903463028481113, 41.25937500034139305, -47.42413220539094709 ) ) ;
#6160=FACE_OUTER_BOUND ( 'NONE', #5182, .T. ) ;
#6167=CARTESIAN_POINT ( 'NONE',  ( 0.000000000000000000, 45.07596123493892293, 0.000000000000000000 ) ) ;
#6168=CARTESIAN_POINT ( 'NONE',  ( -40.45084971874737789, 47.58125000068280031, -29.38926261462365730 ) ) ;
#6169=CARTESIAN_POINT ( 'NONE',  ( 7.919222016226809657, 45.22999571913594963, -50.00000000000000000 ) ) ;
#6171=CARTESIAN_POINT ( 'NONE',  ( -30.90169943749474513, 25.69999999999999574, -42.53254041760200721 ) ) ;
#6184=CARTESIAN_POINT ( 'NONE',  ( -30.81806926056962226, 22.22187500034139163, 42.41743335407647919 ) ) ;
#6185=CARTESIAN_POINT ( 'NONE',  ( -49.86468353124999453, 29.75937500034139305, -16.20201782572375393 ) ) ;
#6187=CARTESIAN_POINT ( 'NONE',  ( 40.34137639590981195, 35.12187500034139731, -29.30972558990011834 ) ) ;
#6189=CARTESIAN_POINT ( 'NONE',  ( -3.219174618344376363E-15, 39.49999999999999289, -52.57311121191334990 ) ) ;
#6190=CARTESIAN_POINT ( 'NONE',  ( 9.631387414534489405E-15, 40.35937500034139447, 52.43083105670540789 ) ) ;
#6193=CARTESIAN_POINT ( 'NONE',  ( -49.99999999999999289, 42.09999999999999432, 16.24598481164533226 ) ) ;
#6194=ORIENTED_EDGE ( 'NONE', *, *, #1205, .F. ) ;
#6200=CARTESIAN_POINT ( 'NONE',  ( -40.45084971874737079, 34.20000000000000284, 29.38926261462367151 ) ) ;
#6204=CARTESIAN_POINT ( 'NONE',  ( 15.40903463028481113, 45.32187500034140015, -47.42413220539094709 ) ) ;
#6207=CARTESIAN_POINT ( 'NONE',  ( -49.99999999999999289, 25.88125000068280102, 16.24598481164533226 ) ) ;
#6209=CARTESIAN_POINT ( 'NONE',  ( -30.81806926056963292, 33.62187500034139731, -42.41743335407647209 ) ) ;
#6219=CARTESIAN_POINT ( 'NONE',  ( -7.919222016226809657, 49.33250428222964246, -49.99999999999999289 ) ) ;
#6221=CARTESIAN_POINT ( 'NONE',  ( 30.81806926056964002, 32.55937500034139731, 42.41743335407647209 ) ) ;
#6222=DIRECTION ( 'NONE',  ( 0.000000000000000000, 0.000000000000000000, -1.000000000000000000 ) ) ;
#6224=CARTESIAN_POINT ( 'NONE',  ( 15.40903463028482356, 48.52187500034140299, 47.42413220539093999 ) ) ;
#6235=CARTESIAN_POINT ( 'NONE',  ( 15.45084971874737789, 34.38125000068280457, 47.55282581475767500 ) ) ;
#6240=CARTESIAN_POINT ( 'NONE',  ( 30.90169943749475223, 32.48125000068280599, 42.53254041760199300 ) ) ;
#6245=( NAMED_UNIT ( * ) SI_UNIT ( $, .STERADIAN. ) SOLID_ANGLE_UNIT ( ) );
#6247=CARTESIAN_POINT ( 'NONE',  ( 40.45084971874737789, 48.58125000068280031, 29.38926261462365375 ) ) ;
#6251=CARTESIAN_POINT ( 'NONE',  ( 49.86468353124999453, 20.95937500034138878, -16.20201782572376459 ) ) ;
#6252=EDGE_CURVE ( 'NONE', #9264, #5867, #4037, .T. ) ;
#6257=VERTEX_POINT ( 'NONE', #3610 ) ;
#6258=AXIS2_PLACEMENT_3D ( 'NONE', #7201, #8596, #4974 ) ;
#6260=B_SPLINE_CURVE_WITH_KNOTS ( 'NONE', 3,
 ( #12462, #9884, #11141, #14937 ),
 .UNSPECIFIED., .F., .F.,
 ( 4, 4 ),
 ( 0.000000000000000000, 0.01231015999390909152 ),
 .UNSPECIFIED. ) ;
#6267=CARTESIAN_POINT ( 'NONE',  ( -40.34137639590981905, 25.72187500034139518, -29.30972558990011478 ) ) ;
#6268=CARTESIAN_POINT ( 'NONE',  ( 40.34137639590981195, 23.05937500034139731, -29.30972558990011834 ) ) ;
#6270=CARTESIAN_POINT ( 'NONE',  ( -3.210462471511496205E-15, 35.42187500034140157, -52.43083105670540789 ) ) ;
#6272=CARTESIAN_POINT ( 'NONE',  ( 40.45084971874737789, 32.80000000000000426, 29.38926261462365375 ) ) ;
#6273=CARTESIAN_POINT ( 'NONE',  ( 49.86468353125001585, 38.75937500034139305, 16.20201782572375038 ) ) ;
#6276=CIRCLE ( 'NONE', #12681, 17.50000000000000000 ) ;
#6277=CARTESIAN_POINT ( 'NONE',  ( 30.90169943749475578, 42.69999999999999574, 42.53254041760200010 ) ) ;
#6285=CARTESIAN_POINT ( 'NONE',  ( -40.45084971874737789, 33.80000000000000426, -29.38926261462365730 ) ) ;
#6290=CARTESIAN_POINT ( 'NONE',  ( -3.210462471511496205E-15, 45.42187500034139447, -52.43083105670540789 ) ) ;
#6293=CARTESIAN_POINT ( 'NONE',  ( -50.00000000000000000, 29.78125000068279959, 0.000000000000000000 ) ) ;
#6294=CARTESIAN_POINT ( 'NONE',  ( 13.19280092631089829, 34.01215678592156877, 93.07304329697090850 ) ) ;
#6295=CARTESIAN_POINT ( 'NONE',  ( 40.34137639590981195, 37.12187500034139731, -29.30972558990011834 ) ) ;
#6300=CARTESIAN_POINT ( 'NONE',  ( 0.000000000000000000, 28.00000000000000355, 0.000000000000000000 ) ) ;
#6301=VERTEX_POINT ( 'NONE', #9674 ) ;
#6308=CARTESIAN_POINT ( 'NONE',  ( -3.210462471511496205E-15, 31.35937500034139092, -52.43083105670540789 ) ) ;
#6312=CARTESIAN_POINT ( 'NONE',  ( -15.40903463028481646, 43.52187500034139589, -47.42413220539093999 ) ) ;
#6317=ORIENTED_EDGE ( 'NONE', *, *, #12767, .F. ) ;
#6323=ORIENTED_EDGE ( 'NONE', *, *, #10226, .F. ) ;
#6330=CARTESIAN_POINT ( 'NONE',  ( -15.40903463028481646, 47.45937500034139589, -47.42413220539093999 ) ) ;
#6339=CARTESIAN_POINT ( 'NONE',  ( 40.34137639590981905, 20.65937500034139873, 29.30972558990010768 ) ) ;
#6340=ORIENTED_EDGE ( 'NONE', *, *, #14552, .T. ) ;
#6342=VERTEX_POINT ( 'NONE', #8507 ) ;
#6349=EDGE_CURVE ( 'NONE', #102, #15191, #15290, .T. ) ;
#6353=CARTESIAN_POINT ( 'NONE',  ( -40.34137639590981195, 26.05937500034139731, 29.30972558990012189 ) ) ;
#6355=ADVANCED_FACE ( 'NONE', ( #8341 ), #10845, .F. ) ;
#6356=CARTESIAN_POINT ( 'NONE',  ( -40.34137639590981905, 35.72187500034139163, -29.30972558990011478 ) ) ;
#6359=CARTESIAN_POINT ( 'NONE',  ( -40.45084971874737789, 31.80000000000000071, -29.38926261462365730 ) ) ;
#6360=CARTESIAN_POINT ( 'NONE',  ( 30.81806926056964002, 36.55937500034139731, 42.41743335407647209 ) ) ;
#6362=CARTESIAN_POINT ( 'NONE',  ( -15.45084971874736368, 46.40000000000000568, 47.55282581475768211 ) ) ;
#6372=CARTESIAN_POINT ( 'NONE',  ( -40.34137639590981195, 40.12187500034139731, 29.30972558990012189 ) ) ;
#6377=CARTESIAN_POINT ( 'NONE',  ( 15.45084971874736723, 27.18125000068279817, -47.55282581475768211 ) ) ;
#6378=CARTESIAN_POINT ( 'NONE',  ( 2.291013771646459141, 39.88729579110228229, 92.94536576005377526 ) ) ;
#6379=( BOUNDED_CURVE ( )  B_SPLINE_CURVE ( 2, ( #6918, #14209, #7986, #4414, #408, #12981, #8156, #6845, #12893, #5352, #4083, #1823, #5662 ),
 .UNSPECIFIED., .F., .F. ) 
 B_SPLINE_CURVE_WITH_KNOTS ( ( 3, 2, 2, 2, 2, 2, 3 ),
 ( 0.2166666666666666741, 0.2200000000000000011, 0.2266666666666666552, 0.2333333333333333370, 0.2399999999999999911, 0.2466666666666666730, 0.2500000000000000000 ),
 .UNSPECIFIED. ) 
 CURVE ( )  GEOMETRIC_REPRESENTATION_ITEM ( )  RATIONAL_B_SPLINE_CURVE ( ( 0.9755282581475768211, 0.9755282581475768211, 1.000000000000000000, 0.9510565162951535312, 1.000000000000000000, 0.9510565162951535312, 1.000000000000000000, 0.9510565162951535312, 1.000000000000000000, 0.9510565162951535312, 1.000000000000000000, 0.9755282581475768211, 0.9755282581475765991 ) ) 
 REPRESENTATION_ITEM ( '' )  );
#6380=AXIS2_PLACEMENT_3D ( 'NONE', #14518, #552, #15690 ) ;
#6381=CARTESIAN_POINT ( 'NONE',  ( -49.86468353124999453, 34.02187500034140299, 16.20201782572377525 ) ) ;
#6382=CARTESIAN_POINT ( 'NONE',  ( 1.293669679204937499E-13, 39.28125000068280315, -50.00000000000000000 ) ) ;
#6389=CARTESIAN_POINT ( 'NONE',  ( -40.34137639590981195, 34.05937500034139731, 29.30972558990012189 ) ) ;
#6391=CARTESIAN_POINT ( 'NONE',  ( 40.34137639590981905, 46.72187500034139873, 29.30972558990010768 ) ) ;
#6399=CARTESIAN_POINT ( 'NONE',  ( -40.45084971874737079, 45.98125000068279888, 29.38926261462367151 ) ) ;
#6400=VERTEX_POINT ( 'NONE', #5040 ) ;
#6401=ORIENTED_EDGE ( 'NONE', *, *, #3975, .T. ) ;
#6411=CARTESIAN_POINT ( 'NONE',  ( -49.99999999999999289, 49.89999999999999147, -16.24598481164531449 ) ) ;
#6412=CARTESIAN_POINT ( 'NONE',  ( -15.45084971874737256, 43.38125000068279746, -47.55282581475767500 ) ) ;
#6423=CYLINDRICAL_SURFACE ( 'NONE', #10015, 50.00000000000000000 ) ;
#6426=CARTESIAN_POINT ( 'NONE',  ( 50.00000000000000711, 32.89999999999999858, 16.24598481164530739 ) ) ;
#6427=CARTESIAN_POINT ( 'NONE',  ( 0.000000000000000000, 20.00000000000000355, 0.000000000000000000 ) ) ;
#6430=ADVANCED_FACE ( 'NONE', ( #9085, #2678 ), #14141, .T. ) ;
#6432=CARTESIAN_POINT ( 'NONE',  ( 49.86468353124999453, 20.95937500034139234, -16.20201782572376104 ) ) ;
#6434=CARTESIAN_POINT ( 'NONE',  ( -15.40903463028480580, 26.32187500034140015, 47.42413220539094709 ) ) ;
#6436=CARTESIAN_POINT ( 'NONE',  ( -40.45084971874737079, 32.20000000000000284, 29.38926261462367151 ) ) ;
#6437=CARTESIAN_POINT ( 'NONE',  ( -15.40903463028480580, 36.25937500034140015, 47.42413220539094709 ) ) ;
#6439=CARTESIAN_POINT ( 'NONE',  ( -30.90169943749473802, 46.30000000000000426, 42.53254041760200721 ) ) ;
#6443=UNCERTAINTY_MEASURE_WITH_UNIT (LENGTH_MEASURE( 1.000000000000000082E-05 ), #5094, 'distance_accuracy_value', 'NONE');
#6449=LINE ( 'NONE', #13829, #7293 ) ;
#6451=EDGE_CURVE ( 'NONE', #15954, #3182, #1342, .T. ) ;
#6453=CARTESIAN_POINT ( 'NONE',  ( -30.81806926056962226, 44.22187500034139163, 42.41743335407647919 ) ) ;
#6454=CARTESIAN_POINT ( 'NONE',  ( -40.34137639590981905, 39.65937500034139873, -29.30972558990011478 ) ) ;
#6458=CARTESIAN_POINT ( 'NONE',  ( -40.45084971874737079, 29.98125000068279888, 29.38926261462367151 ) ) ;
#6460=CARTESIAN_POINT ( 'NONE',  ( 9.631387414534489405E-15, 34.42187500034138736, 52.43083105670540789 ) ) ;
#6469=CARTESIAN_POINT ( 'NONE',  ( 40.34137639590981195, 33.05937500034139731, -29.30972558990011834 ) ) ;
#6471=( BOUNDED_CURVE ( )  B_SPLINE_CURVE ( 2, ( #4746, #635, #5895, #11136, #14932, #13531, #12033, #884, #16023, #4826, #15867, #2133, #7222 ),
 .UNSPECIFIED., .F., .T. ) 
 B_SPLINE_CURVE_WITH_KNOTS ( ( 3, 2, 2, 2, 2, 2, 3 ),
 ( 0.8166666666666666519, 0.8199999999999999512, 0.8266666666666666607, 0.8333333333333333703, 0.8399999999999999689, 0.8466666666666666785, 0.8500000000000000888 ),
 .UNSPECIFIED. ) 
 CURVE ( )  GEOMETRIC_REPRESENTATION_ITEM ( )  RATIONAL_B_SPLINE_CURVE ( ( 0.9755282581475768211, 0.9755282581475768211, 1.000000000000000000, 0.9510565162951535312, 1.000000000000000000, 0.9510565162951535312, 1.000000000000000000, 0.9510565162951535312, 1.000000000000000000, 0.9510565162951535312, 1.000000000000000000, 0.9755282581475763770, 0.9755282581475768211 ) ) 
 REPRESENTATION_ITEM ( '' )  );
#6472=CARTESIAN_POINT ( 'NONE',  ( -30.81806926056962226, 46.22187500034139163, 42.41743335407647209 ) ) ;
#6473=DIRECTION ( 'NONE',  ( 0.000000000000000000, 0.000000000000000000, 1.000000000000000000 ) ) ;
#6480=ORIENTED_EDGE ( 'NONE', *, *, #1427, .F. ) ;
#6485=VECTOR ( 'NONE', #14603, 1000.000000000000000 ) ;
#6488=CARTESIAN_POINT ( 'NONE',  ( 15.40903463028482356, 48.45937500034140299, 47.42413220539093999 ) ) ;
#6494=CARTESIAN_POINT ( 'NONE',  ( 40.45084971874737789, 38.58125000068280031, 29.38926261462365375 ) ) ;
#6506=ORIENTED_EDGE ( 'NONE', *, *, #5809, .T. ) ;
#6507=FACE_OUTER_BOUND ( 'NONE', #15832, .T. ) ;
#6513=CARTESIAN_POINT ( 'NONE',  ( 0.000000000000000000, 20.00000000000000355, 50.00000000000000000 ) ) ;
#6514=CARTESIAN_POINT ( 'NONE',  ( 49.86468353125001585, 20.75937500034140015, 16.20201782572375038 ) ) ;
#6516=CARTESIAN_POINT ( 'NONE',  ( -15.40903463028480580, 30.32187500034140015, 47.42413220539094709 ) ) ;
#6518=CARTESIAN_POINT ( 'NONE',  ( 40.45084971874737789, 28.80000000000000426, 29.38926261462365375 ) ) ;
#6519=CARTESIAN_POINT ( 'NONE',  ( 40.34137639590981195, 35.05937500034139731, -29.30972558990011834 ) ) ;
#6530=CARTESIAN_POINT ( 'NONE',  ( -2.547328955960238000E-13, 34.50000000000000000, 49.99999999999999289 ) ) ;
#6533=CARTESIAN_POINT ( 'NONE',  ( 9.631387414534489405E-15, 36.42187500034139447, 52.43083105670540789 ) ) ;
#6534=CARTESIAN_POINT ( 'NONE',  ( 40.34137639590981195, 45.05937500034139731, -29.30972558990011834 ) ) ;
#6535=CARTESIAN_POINT ( 'NONE',  ( -3.111920190527341144E-15, 35.50000000000000000, -50.00000000000000000 ) ) ;
#6540=CARTESIAN_POINT ( 'NONE',  ( -30.90169943749474868, 29.48125000068279888, -42.53254041760200721 ) ) ;
#6541=APPLICATION_CONTEXT ( 'automotive_design' ) ;
#6542=CARTESIAN_POINT ( 'NONE',  ( 1.152251941144751379, 40.00000000000000711, 92.94692077166136812 ) ) ;
#6544=CARTESIAN_POINT ( 'NONE',  ( -15.40903463028480580, 28.32187500034139660, 47.42413220539094709 ) ) ;
#6546=AXIS2_PLACEMENT_3D ( 'NONE', #1017, #8676, #11102 ) ;
#6548=AXIS2_PLACEMENT_3D ( 'NONE', #9799, #11132, #9957 ) ;
#6554=CARTESIAN_POINT ( 'NONE',  ( 30.90169943749473802, 49.08125000068280031, -42.53254041760200721 ) ) ;
#6558=CARTESIAN_POINT ( 'NONE',  ( 30.81806926056962936, 31.15937500034139518, -42.41743335407647209 ) ) ;
#6562=EDGE_CURVE ( 'NONE', #4835, #10619, #12907, .T. ) ;
#6563=CARTESIAN_POINT ( 'NONE',  ( 49.86468353124999453, 49.02187500034140299, -16.20201782572376104 ) ) ;
#6567=CARTESIAN_POINT ( 'NONE',  ( 40.34137639590981905, 48.72187500034139873, 29.30972558990010768 ) ) ;
#6574=ORIENTED_EDGE ( 'NONE', *, *, #1781, .T. ) ;
#6575=VECTOR ( 'NONE', #2138, 1000.000000000000000 ) ;
#6577=CARTESIAN_POINT ( 'NONE',  ( 7.919222016226758143, 38.33250428222964246, 50.00000000000000711 ) ) ;
#6581=CARTESIAN_POINT ( 'NONE',  ( -15.45084971874736368, 24.40000000000000213, 47.55282581475768211 ) ) ;
#6585=CARTESIAN_POINT ( 'NONE',  ( 15.40903463028481113, 23.32187500034139660, -47.42413220539094709 ) ) ;
#6588=CARTESIAN_POINT ( 'NONE',  ( -49.99999999999999289, 37.88125000068279746, 16.24598481164533226 ) ) ;
#6593=B_SPLINE_CURVE_WITH_KNOTS ( 'NONE', 3,
 ( #11982, #7916, #14385, #9412, #11817, #10588, #14222, #339, #6689, #3006, #423, #15801, #9500, #8167, #1517, #9166, #14547, #10418, #504, #5438, #8075, #6858, #3174, #11661, #11906, #10666, #15717, #14459, #6607, #3089, #10501, #1834, #5363, #15473, #2848, #12991, #1595, #5527, #4189, #9255, #14310, #2930, #7997, #13071, #7333, #8406, #2081, #14878, #9828, #14704, #3335, #7090, #14961, #4677, #13475, #1909, #834, #7003, #16048, #2159, #4589 ),
 .UNSPECIFIED., .F., .F.,
 ( 4, 3, 3, 3, 3, 3, 3, 3, 3, 3, 3, 3, 3, 3, 3, 3, 3, 3, 3, 3, 4 ),
 ( 0.000000000000000000, 0.0001250000981872742046, 0.0006250122739946097549, 0.001125024449802050283, 0.001625036625609320266, 0.002125048801416672649, 0.002625060977223844620, 0.003125073153031289810, 0.003625085328838455277, 0.004125097504645746510, 0.004625109680452854297, 0.005125121856260252649, 0.005625134032067359569, 0.006125146207874817769, 0.006625158383682326277, 0.007125170559489365542, 0.007625182735296597361, 0.008125194911103646167, 0.008625207086911106102, 0.009137502482429510006, 0.009649851960369987616 ),
 .UNSPECIFIED. ) ;
#6602=CARTESIAN_POINT ( 'NONE',  ( -17.28056337048291269, 25.32136411938365583, 93.95934175966624480 ) ) ;
#6606=CARTESIAN_POINT ( 'NONE',  ( -15.40903463028481646, 21.45937500034139589, -47.42413220539093999 ) ) ;
#6607=CARTESIAN_POINT ( 'NONE',  ( -47.13255506291579877, 20.00000000000000355, 16.27994764699678854 ) ) ;
#6608=CARTESIAN_POINT ( 'NONE',  ( -40.34137639590981905, 27.72187500034139873, -29.30972558990011478 ) ) ;
#6610=CARTESIAN_POINT ( 'NONE',  ( 15.45084971874736723, 31.39999999999999858, -47.55282581475768211 ) ) ;
#6611=CARTESIAN_POINT ( 'NONE',  ( -30.81806926056963292, 29.55937500034139376, -42.41743335407647209 ) ) ;
#6613=AXIS2_PLACEMENT_3D ( 'NONE', #13685, #12777, #1378 ) ;
#6624=CARTESIAN_POINT ( 'NONE',  ( -40.34137639590981195, 34.12187500034139731, 29.30972558990012189 ) ) ;
#6625=CARTESIAN_POINT ( 'NONE',  ( 49.86468353124999453, 44.95937500034139589, -16.20201782572376104 ) ) ;
#6630=CARTESIAN_POINT ( 'NONE',  ( -15.45084971874736368, 24.18125000068279817, 47.55282581475768211 ) ) ;
#6631=CARTESIAN_POINT ( 'NONE',  ( 16.40338228813142507, 28.62403330670708002, 93.52543394180021608 ) ) ;
#6632=CARTESIAN_POINT ( 'NONE',  ( -49.86468353125000164, 27.92187500034139447, 0.000000000000000000 ) ) ;
#6635=VECTOR ( 'NONE', #11715, 1000.000000000000000 ) ;
#6639=VERTEX_POINT ( 'NONE', #5601 ) ;
#6640=EDGE_CURVE ( 'NONE', #2321, #15727, #6593, .T. ) ;
#6645=CARTESIAN_POINT ( 'NONE',  ( 15.40903463028482356, 22.45937500034139589, 47.42413220539093999 ) ) ;
#6648=CARTESIAN_POINT ( 'NONE',  ( -3.210462471511496205E-15, 41.42187500034139447, -52.43083105670540789 ) ) ;
#6651=CARTESIAN_POINT ( 'NONE',  ( 49.86468353125000164, 48.92187500034139447, -6.106662507704105588E-15 ) ) ;
#6655=EDGE_LOOP ( 'NONE', ( #12711, #2859, #11060, #133 ) ) ;
#6659=DIRECTION ( 'NONE',  ( 1.000000000000000000, 0.000000000000000000, 0.000000000000000000 ) ) ;
#6662=CARTESIAN_POINT ( 'NONE',  ( 9.657523855033129090E-15, 26.50000000000000355, 52.57311121191334990 ) ) ;
#6663=CARTESIAN_POINT ( 'NONE',  ( 30.81806926056962936, 43.15937500034140584, -42.41743335407647209 ) ) ;
#6666=CARTESIAN_POINT ( 'NONE',  ( -3.210462471511496205E-15, 21.42187500034139802, -52.43083105670540789 ) ) ;
#6668=APPLICATION_CONTEXT ( 'automotive_design' ) ;
#6670=CARTESIAN_POINT ( 'NONE',  ( 50.00000000000000711, 42.68125000068280173, 16.24598481164530739 ) ) ;
#6671=LINE ( 'NONE', #5267, #14502 ) ;
#6672=CARTESIAN_POINT ( 'NONE',  ( 15.45084971874736723, 21.18125000068279817, -47.55282581475768211 ) ) ;
#6687=CARTESIAN_POINT ( 'NONE',  ( -7.919222016226870942, 38.22999571913595673, 49.99999999999997158 ) ) ;
#6688=CARTESIAN_POINT ( 'NONE',  ( 17.35865297518751049, 20.20728047528196925, 94.86179832180087601 ) ) ;
#6689=CARTESIAN_POINT ( 'NONE',  ( -48.11476475577501333, 20.00000000000000355, 13.09518440665035754 ) ) ;
#6690=CARTESIAN_POINT ( 'NONE',  ( -3.210462471511496205E-15, 27.42187500034139092, -52.43083105670540789 ) ) ;
#6693=CARTESIAN_POINT ( 'NONE',  ( -30.81806926056963292, 31.55937500034139731, -42.41743335407647209 ) ) ;
#6701=CARTESIAN_POINT ( 'NONE',  ( -49.99999999999999289, 37.90000000000000568, -16.24598481164531449 ) ) ;
#6704=CARTESIAN_POINT ( 'NONE',  ( -49.86468353125000164, 33.92187500034139447, 0.000000000000000000 ) ) ;
#6705=CARTESIAN_POINT ( 'NONE',  ( -3.210462471511496205E-15, 37.35937500034140157, -52.43083105670540789 ) ) ;
#6708=CARTESIAN_POINT ( 'NONE',  ( 40.34137639590981195, 49.05937500034139731, -29.30972558990011834 ) ) ;
#6711=CARTESIAN_POINT ( 'NONE',  ( 40.34137639590981905, 28.72187500034139873, 29.30972558990010768 ) ) ;
#6722=CARTESIAN_POINT ( 'NONE',  ( -40.34137639590981905, 25.65937500034139518, -29.30972558990011478 ) ) ;
#6726=CARTESIAN_POINT ( 'NONE',  ( 49.86468353125001585, 40.82187500034140726, 16.20201782572375038 ) ) ;
#6729=CARTESIAN_POINT ( 'NONE',  ( 30.81806926056962936, 45.22187500034139873, -42.41743335407647209 ) ) ;
#6740=CARTESIAN_POINT ( 'NONE',  ( -30.90169943749474513, 43.48125000068279178, -42.53254041760200721 ) ) ;
#6741=CARTESIAN_POINT ( 'NONE',  ( 50.00000000000000000, 38.78125000068279604, -6.123233995736766085E-15 ) ) ;
#6743=CARTESIAN_POINT ( 'NONE',  ( 30.90169943749475578, 24.69999999999999929, 42.53254041760200010 ) ) ;
#6744=CARTESIAN_POINT ( 'NONE',  ( -3.210462471511496205E-15, 41.35937500034138736, -52.43083105670540789 ) ) ;
#6745=CARTESIAN_POINT ( 'NONE',  ( -30.90169943749474513, 25.48125000068279888, -42.53254041760200721 ) ) ;
#6749=EDGE_CURVE ( 'NONE', #15727, #12890, #1994, .T. ) ;
#6752=CARTESIAN_POINT ( 'NONE',  ( 50.00000000000000711, 40.68125000068280173, 16.24598481164530739 ) ) ;
#6761=VECTOR ( 'NONE', #6090, 1000.000000000000000 ) ;
#6771=CARTESIAN_POINT ( 'NONE',  ( 0.000000000000000000, 28.00000000000000355, 0.000000000000000000 ) ) ;
#6773=ADVANCED_FACE ( 'NONE', ( #1320 ), #10230, .F. ) ;
#6774=CARTESIAN_POINT ( 'NONE',  ( -30.81806926056962226, 30.22187500034139518, 42.41743335407647209 ) ) ;
#6778=CARTESIAN_POINT ( 'NONE',  ( 30.81806926056964002, 32.55937500034139731, 42.41743335407647209 ) ) ;
#6789=CARTESIAN_POINT ( 'NONE',  ( -15.40903463028481646, 35.52187500034139589, -47.42413220539093999 ) ) ;
#6790=CARTESIAN_POINT ( 'NONE',  ( -49.86468353124999453, 37.75937500034140015, -16.20201782572375393 ) ) ;
#6793=CARTESIAN_POINT ( 'NONE',  ( 15.45084971874737789, 22.38125000068280102, 47.55282581475767500 ) ) ;
#6796=CARTESIAN_POINT ( 'NONE',  ( -15.40903463028481646, 27.52187500034139944, -47.42413220539093999 ) ) ;
#6797=CARTESIAN_POINT ( 'NONE',  ( -40.45084971874737079, 27.98125000068279888, 29.38926261462367151 ) ) ;
#6804=CARTESIAN_POINT ( 'NONE',  ( 49.99999999999999289, 30.88125000068279746, -16.24598481164532160 ) ) ;
#6806=CARTESIAN_POINT ( 'NONE',  ( 30.81806926056964002, 24.55937500034139376, 42.41743335407647209 ) ) ;
#6808=CARTESIAN_POINT ( 'NONE',  ( 49.86468353125001585, 38.82187500034140015, 16.20201782572375038 ) ) ;
#6810=CARTESIAN_POINT ( 'NONE',  ( 9.631387414534489405E-15, 48.42187500034140157, 52.43083105670540789 ) ) ;
#6811=CARTESIAN_POINT ( 'NONE',  ( 49.99999999999999289, 31.09999999999999787, -16.24598481164532160 ) ) ;
#6824=CARTESIAN_POINT ( 'NONE',  ( -50.00000000000000000, 26.00000000000000355, 0.000000000000000000 ) ) ;
#6826=CARTESIAN_POINT ( 'NONE',  ( 30.81806926056964002, 46.55937500034139020, 42.41743335407647209 ) ) ;
#6833=CARTESIAN_POINT ( 'NONE',  ( 40.45084971874737079, 32.98125000068279888, -29.38926261462366440 ) ) ;
#6836=CARTESIAN_POINT ( 'NONE',  ( 2.600676159226420495E-13, 21.28125000068279604, -49.99999999999999289 ) ) ;
#6842=VECTOR ( 'NONE', #13061, 1000.000000000000000 ) ;
#6844=EDGE_CURVE ( 'NONE', #1788, #6342, #528, .T. ) ;
#6845=CARTESIAN_POINT ( 'NONE',  ( 50.00000000000000711, 42.89999999999999147, 16.24598481164530739 ) ) ;
#6850=CARTESIAN_POINT ( 'NONE',  ( -50.00000000000000000, 20.00000000000000000, 0.000000000000000000 ) ) ;
#6858=CARTESIAN_POINT ( 'NONE',  ( -47.50025713571316999, 20.00000000000001066, 15.17274647889583861 ) ) ;
#6859=CARTESIAN_POINT ( 'NONE',  ( -49.86468353125000164, 23.92187500034139447, 0.000000000000000000 ) ) ;
#6860=AXIS2_PLACEMENT_3D ( 'NONE', #6898, #11952, #9381 ) ;
#6863=CARTESIAN_POINT ( 'NONE',  ( -49.86468353125000164, 33.85937500034139447, 0.000000000000000000 ) ) ;
#6864=CARTESIAN_POINT ( 'NONE',  ( 15.45084971874736723, 39.40000000000000568, -47.55282581475768211 ) ) ;
#6871=CARTESIAN_POINT ( 'NONE',  ( -15.40903463028480580, 38.32187500034140015, 47.42413220539094709 ) ) ;
#6872=CARTESIAN_POINT ( 'NONE',  ( 49.86468353125001585, 38.75937500034139305, 16.20201782572375038 ) ) ;
#6875=CARTESIAN_POINT ( 'NONE',  ( -15.45084971874737256, 23.38125000068280102, -47.55282581475767500 ) ) ;
#6877=CARTESIAN_POINT ( 'NONE',  ( -15.40903463028480580, 30.32187500034140015, 47.42413220539094709 ) ) ;
#6887=CARTESIAN_POINT ( 'NONE',  ( 15.40903463028481113, 23.25937500034139660, -47.42413220539094709 ) ) ;
#6889=CARTESIAN_POINT ( 'NONE',  ( -40.34137639590981905, 39.72187500034139873, -29.30972558990011478 ) ) ;
#6892=CARTESIAN_POINT ( 'NONE',  ( 9.631387414534489405E-15, 44.42187500034140157, 52.43083105670540789 ) ) ;
#6898=CARTESIAN_POINT ( 'NONE',  ( 0.000000000000000000, 22.50000000000000000, 80.00000000000000000 ) ) ;
#6901=CARTESIAN_POINT ( 'NONE',  ( 15.45084971874737789, 22.60000000000000142, 47.55282581475767500 ) ) ;
#6903=CARTESIAN_POINT ( 'NONE',  ( 40.34137639590981195, 41.05937500034139731, -29.30972558990011834 ) ) ;
#6908=CARTESIAN_POINT ( 'NONE',  ( 50.00000000000000711, 32.68125000068279462, 16.24598481164530739 ) ) ;
#6909=DIRECTION ( 'NONE',  ( 0.000000000000000000, 1.000000000000000000, 0.000000000000000000 ) ) ;
#6910=CARTESIAN_POINT ( 'NONE',  ( 7.919222016226875382, 37.44874571845315359, -49.99999999999997158 ) ) ;
#6917=ORIENTED_EDGE ( 'NONE', *, *, #11253, .T. ) ;
#6918=CARTESIAN_POINT ( 'NONE',  ( -3.111920190527341144E-15, 43.50000000000000711, -50.00000000000000000 ) ) ;
#6926=CARTESIAN_POINT ( 'NONE',  ( -15.45084971874736368, 30.18125000068280173, 47.55282581475768211 ) ) ;
#6927=CARTESIAN_POINT ( 'NONE',  ( 50.00000000000000711, 46.90000000000000568, 16.24598481164530739 ) ) ;
#6931=CARTESIAN_POINT ( 'NONE',  ( 30.81806926056964002, 22.62187500034139731, 42.41743335407646498 ) ) ;
#6934=CARTESIAN_POINT ( 'NONE',  ( -3.210462471511496205E-15, 27.35937500034139802, -52.43083105670540789 ) ) ;
#6942=EDGE_CURVE ( 'NONE', #15954, #14909, #12047, .T. ) ;
#6945=CARTESIAN_POINT ( 'NONE',  ( -40.34137639590981195, 32.12187500034140442, 29.30972558990012189 ) ) ;
#6946=CARTESIAN_POINT ( 'NONE',  ( -15.40903463028480580, 34.25937500034139305, 47.42413220539094709 ) ) ;
#6950=CARTESIAN_POINT ( 'NONE',  ( 49.86468353125001585, 42.75937500034138594, 16.20201782572375038 ) ) ;
#6953=CARTESIAN_POINT ( 'NONE',  ( 15.45084971874736723, 49.39999999999999858, -47.55282581475768211 ) ) ;
#6961=CARTESIAN_POINT ( 'NONE',  ( -50.00000000000000000, 33.78125000068280315, 0.000000000000000000 ) ) ;
#6963=CARTESIAN_POINT ( 'NONE',  ( 49.86468353125000164, 22.85937500034139802, -6.106662507704105588E-15 ) ) ;
#6966=CARTESIAN_POINT ( 'NONE',  ( 30.90169943749475578, 34.70000000000000995, 42.53254041760200010 ) ) ;
#6968=CARTESIAN_POINT ( 'NONE',  ( -49.86468353124999453, 43.82187500034140015, -16.20201782572375393 ) ) ;
#6977=CARTESIAN_POINT ( 'NONE',  ( -15.40903463028480580, 44.25937500034140015, 47.42413220539094709 ) ) ;
#6981=CARTESIAN_POINT ( 'NONE',  ( -1.240322475938754499E-13, 36.28125000068280315, 50.00000000000000000 ) ) ;
#6983=CARTESIAN_POINT ( 'NONE',  ( 40.45084971874737079, 22.98125000068279888, -29.38926261462366440 ) ) ;
#6987=ADVANCED_FACE ( 'NONE', ( #15045 ), #5265, .F. ) ;
#6999=CARTESIAN_POINT ( 'NONE',  ( 6.123233995736766085E-15, 20.00000000000000355, -50.00000000000000000 ) ) ;
#7001=CARTESIAN_POINT ( 'NONE',  ( -7.919222016226804328, 48.44874571845315359, 50.00000000000000000 ) ) ;
#7003=CARTESIAN_POINT ( 'NONE',  ( -45.33038492356476468, 20.00000000000001776, 20.77601661419166845 ) ) ;
#7004=CARTESIAN_POINT ( 'NONE',  ( -49.86468353124999453, 24.02187500034139589, 16.20201782572377169 ) ) ;
#7008=CARTESIAN_POINT ( 'NONE',  ( -40.34137639590981905, 23.65937500034139518, -29.30972558990011478 ) ) ;
#7013=ORIENTED_EDGE ( 'NONE', *, *, #8927, .F. ) ;
#7017=CARTESIAN_POINT ( 'NONE',  ( 50.00000000000000711, 34.89999999999999858, 16.24598481164530739 ) ) ;
#7020=CARTESIAN_POINT ( 'NONE',  ( 49.86468353124999453, 27.02187500034139589, -16.20201782572376459 ) ) ;
#7021=CARTESIAN_POINT ( 'NONE',  ( 40.34137639590981905, 34.65937500034139873, 29.30972558990010768 ) ) ;
#7022=CARTESIAN_POINT ( 'NONE',  ( -3.111920190527341144E-15, 43.50000000000000711, -50.00000000000000000 ) ) ;
#7025=CARTESIAN_POINT ( 'NONE',  ( -3.210462471511496205E-15, 43.35937500034138736, -52.43083105670540789 ) ) ;
#7028=CARTESIAN_POINT ( 'NONE',  ( -40.34137639590981905, 23.72187500034139873, -29.30972558990011478 ) ) ;
#7031=EDGE_CURVE ( 'NONE', #7298, #15854, #482, .T. ) ;
#7040=CARTESIAN_POINT ( 'NONE',  ( 15.40903463028482356, 46.52187500034139589, 47.42413220539093999 ) ) ;
#7042=CARTESIAN_POINT ( 'NONE',  ( -50.00000000000000000, 38.00000000000000711, 0.000000000000000000 ) ) ;
#7043=CARTESIAN_POINT ( 'NONE',  ( -15.40903463028480580, 38.32187500034140015, 47.42413220539094709 ) ) ;
#7055=CARTESIAN_POINT ( 'NONE',  ( 50.00000000000000000, 36.78125000068280315, -6.123233995736766085E-15 ) ) ;
#7056=CARTESIAN_POINT ( 'NONE',  ( 15.40903463028481113, 37.25937500034140015, -47.42413220539094709 ) ) ;
#7057=CARTESIAN_POINT ( 'NONE',  ( -49.86468353124999453, 49.75937500034137884, -16.20201782572375393 ) ) ;
#7067=ORIENTED_EDGE ( 'NONE', *, *, #1371, .F. ) ;
#7090=CARTESIAN_POINT ( 'NONE',  ( -45.74278786629260907, 19.99999999999998934, 19.85154960931437174 ) ) ;
#7091=CARTESIAN_POINT ( 'NONE',  ( 30.81806926056962936, 21.22187500034139518, -42.41743335407646498 ) ) ;
#7095=CARTESIAN_POINT ( 'NONE',  ( 49.86468353124999453, 22.95937500034139589, -16.20201782572376459 ) ) ;
#7099=ORIENTED_EDGE ( 'NONE', *, *, #11253, .F. ) ;
#7102=ORIENTED_EDGE ( 'NONE', *, *, #12301, .T. ) ;
#7103=CYLINDRICAL_SURFACE ( 'NONE', #14769, 50.00000000000000000 ) ;
#7105=AXIS2_PLACEMENT_3D ( 'NONE', #3311, #11050, #14858 ) ;
#7107=CARTESIAN_POINT ( 'NONE',  ( 15.45084971874737789, 34.60000000000000853, 47.55282581475767500 ) ) ;
#7110=CARTESIAN_POINT ( 'NONE',  ( -49.86468353124999453, 31.82187500034139305, -16.20201782572375393 ) ) ;
#7111=CARTESIAN_POINT ( 'NONE',  ( -40.34137639590981195, 28.05937500034139731, 29.30972558990012189 ) ) ;
#7112=DIRECTION ( 'NONE',  ( -0.000000000000000000, -0.000000000000000000, -1.000000000000000000 ) ) ;
#7115=CARTESIAN_POINT ( 'NONE',  ( -30.81806926056962226, 46.15937500034139873, 42.41743335407647919 ) ) ;
#7117=CARTESIAN_POINT ( 'NONE',  ( 15.40903463028481113, 23.32187500034139660, -47.42413220539094709 ) ) ;
#7126=CARTESIAN_POINT ( 'NONE',  ( 15.40903463028481113, 49.32187500034139305, -47.42413220539094709 ) ) ;
#7129=CARTESIAN_POINT ( 'NONE',  ( 40.45084971874737079, 39.19999999999999574, -29.38926261462366440 ) ) ;
#7131=CARTESIAN_POINT ( 'NONE',  ( -49.86468353125000164, 37.92187500034140157, 0.000000000000000000 ) ) ;
#7132=CARTESIAN_POINT ( 'NONE',  ( 6.123233995736766085E-15, 20.00000000000000355, -50.00000000000000000 ) ) ;
#7139=CYLINDRICAL_SURFACE ( 'NONE', #4450, 50.00000000000000000 ) ;
#7141=EDGE_CURVE ( 'NONE', #2703, #4062, #885, .T. ) ;
#7142=CARTESIAN_POINT ( 'NONE',  ( 50.00000000000000711, 26.89999999999999858, 16.24598481164530739 ) ) ;
#7144=CARTESIAN_POINT ( 'NONE',  ( 49.86468353124999453, 34.95937500034138878, -16.20201782572376459 ) ) ;
#7145=CARTESIAN_POINT ( 'NONE',  ( -49.86468353124999453, 45.75937500034140015, -16.20201782572375393 ) ) ;
#7148=AXIS2_PLACEMENT_3D ( 'NONE', #15694, #9311, #1730 ) ;
#7151=CARTESIAN_POINT ( 'NONE',  ( -50.00000000000000000, 46.00000000000000000, 0.000000000000000000 ) ) ;
#7157=ORIENTED_EDGE ( 'NONE', *, *, #13518, .T. ) ;
#7165=CARTESIAN_POINT ( 'NONE',  ( -17.50000000000000000, 22.50000000000000000, 94.42467108177066848 ) ) ;
#7168=FACE_OUTER_BOUND ( 'NONE', #228, .T. ) ;
#7171=CARTESIAN_POINT ( 'NONE',  ( -40.34137639590981905, 25.72187500034139518, -29.30972558990011478 ) ) ;
#7174=CARTESIAN_POINT ( 'NONE',  ( -30.81806926056962226, 28.15937500034139518, 42.41743335407647919 ) ) ;
#7175=CARTESIAN_POINT ( 'NONE',  ( -50.00000000000000000, 30.00000000000000355, 0.000000000000000000 ) ) ;
#7180=CARTESIAN_POINT ( 'NONE',  ( 0.000000000000000000, 20.00000000000000355, 0.000000000000000000 ) ) ;
#7185=CARTESIAN_POINT ( 'NONE',  ( -30.81806926056962226, 32.22187500034139163, 42.41743335407647919 ) ) ;
#7186=CARTESIAN_POINT ( 'NONE',  ( -30.81806926056962226, 28.15937500034139518, 42.41743335407647209 ) ) ;
#7190=CARTESIAN_POINT ( 'NONE',  ( -49.86468353125000164, 47.85937500034139447, 0.000000000000000000 ) ) ;
#7192=CARTESIAN_POINT ( 'NONE',  ( 30.81806926056962936, 23.22187500034139163, -42.41743335407647209 ) ) ;
#7195=ORIENTED_EDGE ( 'NONE', *, *, #9559, .F. ) ;
#7200=CARTESIAN_POINT ( 'NONE',  ( 15.40903463028481113, 21.25937500034139660, -47.42413220539094709 ) ) ;
#7201=CARTESIAN_POINT ( 'NONE',  ( 0.000000000000000000, 20.00000000000000355, 0.000000000000000000 ) ) ;
#7205=CARTESIAN_POINT ( 'NONE',  ( 30.90169943749474157, 33.08125000068279320, -42.53254041760200721 ) ) ;
#7206=CARTESIAN_POINT ( 'NONE',  ( -3.210462471511496205E-15, 41.42187500034140157, -52.43083105670540789 ) ) ;
#7213=ORIENTED_EDGE ( 'NONE', *, *, #13545, .F. ) ;
#7218=CARTESIAN_POINT ( 'NONE',  ( 40.45084971874737789, 26.80000000000000071, 29.38926261462365375 ) ) ;
#7220=CARTESIAN_POINT ( 'NONE',  ( 40.34137639590981905, 36.65937500034139873, 29.30972558990010768 ) ) ;
#7222=CARTESIAN_POINT ( 'NONE',  ( -2.547328955960238000E-13, 24.49999999999999289, 49.99999999999999289 ) ) ;
#7227=CARTESIAN_POINT ( 'NONE',  ( 30.90169943749475223, 36.70000000000000284, 42.53254041760199300 ) ) ;
#7242=CARTESIAN_POINT ( 'NONE',  ( -17.27575688642330221, 19.64968859734266715, 94.97692319343484257 ) ) ;
#7251=CARTESIAN_POINT ( 'NONE',  ( -40.45084971874737789, 49.58125000068280031, -29.38926261462365730 ) ) ;
#7255=CARTESIAN_POINT ( 'NONE',  ( 49.86468353125000164, 26.85937500034139802, -6.106662507704105588E-15 ) ) ;
#7256=CARTESIAN_POINT ( 'NONE',  ( -15.45084971874737256, 41.38125000068279746, -47.55282581475767500 ) ) ;
#7262=CARTESIAN_POINT ( 'NONE',  ( -3.111920190527341144E-15, 43.50000000000000711, -50.00000000000000000 ) ) ;
#7269=EDGE_CURVE ( 'NONE', #6137, #7369, #8379, .T. ) ;
#7270=CARTESIAN_POINT ( 'NONE',  ( -40.34137639590981195, 28.12187500034139731, 29.30972558990012189 ) ) ;
#7271=CARTESIAN_POINT ( 'NONE',  ( 15.40903463028482356, 28.45937500034139589, 47.42413220539093999 ) ) ;
#7272=CARTESIAN_POINT ( 'NONE',  ( 15.45084971874736723, 27.18125000068279817, -47.55282581475768211 ) ) ;
#7276=CARTESIAN_POINT ( 'NONE',  ( 15.40903463028481113, 43.25937500034139305, -47.42413220539094709 ) ) ;
#7278=CARTESIAN_POINT ( 'NONE',  ( -15.40903463028480580, 22.32187500034139660, 47.42413220539094709 ) ) ;
#7289=CARTESIAN_POINT ( 'NONE',  ( 40.34137639590981905, 20.65937500034139873, 29.30972558990010768 ) ) ;
#7292=CARTESIAN_POINT ( 'NONE',  ( -15.45084971874736368, 36.18125000068280173, 47.55282581475768211 ) ) ;
#7293=VECTOR ( 'NONE', #1442, 1000.000000000000000 ) ;
#7294=CARTESIAN_POINT ( 'NONE',  ( -30.81806926056963292, 43.62187500034139020, -42.41743335407647209 ) ) ;
#7298=VERTEX_POINT ( 'NONE', #4653 ) ;
#7299=ORIENTED_EDGE ( 'NONE', *, *, #4180, .F. ) ;
#7302=CARTESIAN_POINT ( 'NONE',  ( -49.99999999999999289, 39.68125000068280173, -16.24598481164531449 ) ) ;
#7307=CARTESIAN_POINT ( 'NONE',  ( 49.86468353124999453, 40.95937500034140299, -16.20201782572376459 ) ) ;
#7308=CARTESIAN_POINT ( 'NONE',  ( 49.86468353124999453, 42.95937500034139589, -16.20201782572376104 ) ) ;
#7315=CIRCLE ( 'NONE', #8907, 92.05189185291139609 ) ;
#7322=DIRECTION ( 'NONE',  ( -0.000000000000000000, 1.000000000000000000, -0.000000000000000000 ) ) ;
#7324=CARTESIAN_POINT ( 'NONE',  ( 8.446640517145639571E-15, 48.28125000068279604, 50.00000000000000000 ) ) ;
#7326=CARTESIAN_POINT ( 'NONE',  ( -17.50000000000000355, 21.92963385674405785, 94.52695465929356544 ) ) ;
#7331=CARTESIAN_POINT ( 'NONE',  ( -2.547328955960238000E-13, 32.50000000000000000, 49.99999999999999289 ) ) ;
#7333=CARTESIAN_POINT ( 'NONE',  ( -46.19495089481165451, 20.00000000000000355, 18.77607397657153143 ) ) ;
#7334=FACE_OUTER_BOUND ( 'NONE', #4603, .T. ) ;
#7337=CARTESIAN_POINT ( 'NONE',  ( -49.99999999999999289, 26.10000000000000142, 16.24598481164533226 ) ) ;
#7340=EDGE_CURVE ( 'NONE', #6342, #9634, #5734, .T. ) ;
#7355=CARTESIAN_POINT ( 'NONE',  ( -3.210462471511496205E-15, 25.42187500034139092, -52.43083105670540789 ) ) ;
#7356=CARTESIAN_POINT ( 'NONE',  ( 30.81806926056964002, 28.55937500034139376, 42.41743335407646498 ) ) ;
#7360=CARTESIAN_POINT ( 'NONE',  ( 30.81806926056964002, 38.62187500034139020, 42.41743335407646498 ) ) ;
#7363=CARTESIAN_POINT ( 'NONE',  ( -30.81806926056963292, 35.55937500034139020, -42.41743335407647209 ) ) ;
#7365=CARTESIAN_POINT ( 'NONE',  ( 40.45084971874737789, 44.79999999999999716, 29.38926261462365375 ) ) ;
#7366=ORIENTED_EDGE ( 'NONE', *, *, #12974, .T. ) ;
#7369=VERTEX_POINT ( 'NONE', #3310 ) ;
#7374=CARTESIAN_POINT ( 'NONE',  ( 40.34137639590981195, 49.12187500034139731, -29.30972558990011834 ) ) ;
#7375=LINE ( 'NONE', #2036, #8105 ) ;
#7377=CARTESIAN_POINT ( 'NONE',  ( 50.00000000000000000, 34.78125000068280315, -6.123233995736766085E-15 ) ) ;
#7378=CARTESIAN_POINT ( 'NONE',  ( 15.40903463028482356, 36.52187500034139589, 47.42413220539093999 ) ) ;
#7389=CARTESIAN_POINT ( 'NONE',  ( 7.919222016226822092, 26.55125428154684641, 49.99999999999999289 ) ) ;
#7391=CARTESIAN_POINT ( 'NONE',  ( 49.86468353125001585, 38.75937500034139305, 16.20201782572375038 ) ) ;
#7392=CARTESIAN_POINT ( 'NONE',  ( -15.40903463028481646, 41.45937500034140299, -47.42413220539093999 ) ) ;
#7393=CARTESIAN_POINT ( 'NONE',  ( -1.224646799147353217E-14, 0.000000000000000000, -100.0000000000000000 ) ) ;
#7395=CARTESIAN_POINT ( 'NONE',  ( 15.45084971874736723, 41.40000000000000568, -47.55282581475768211 ) ) ;
#7396=CARTESIAN_POINT ( 'NONE',  ( 1.293669679204937499E-13, 41.50000000000000000, -50.00000000000000000 ) ) ;
#7401=ORIENTED_EDGE ( 'NONE', *, *, #12294, .F. ) ;
#7403=CARTESIAN_POINT ( 'NONE',  ( -7.919222016226870942, 40.44874571845315359, 49.99999999999997158 ) ) ;
#7404=CARTESIAN_POINT ( 'NONE',  ( -3.111920190527341144E-15, 29.50000000000000000, -50.00000000000000000 ) ) ;
#7407=DIRECTION ( 'NONE',  ( -0.000000000000000000, 1.000000000000000000, -0.000000000000000000 ) ) ;
#7408=CARTESIAN_POINT ( 'NONE',  ( -0.5790451294426995910, 4.999999999999993783, 99.11836509645767990 ) ) ;
#7414=CARTESIAN_POINT ( 'NONE',  ( 40.45084971874737079, 46.98125000068280599, -29.38926261462366440 ) ) ;
#7418=CARTESIAN_POINT ( 'NONE',  ( 40.34137639590981905, 22.65937500034139518, 29.30972558990010768 ) ) ;
#7419=CARTESIAN_POINT ( 'NONE',  ( -30.90169943749473447, 42.08125000068279320, 42.53254041760200721 ) ) ;
#7424=CARTESIAN_POINT ( 'NONE',  ( 40.45084971874737079, 49.20000000000000284, -29.38926261462366440 ) ) ;
#7432=CARTESIAN_POINT ( 'NONE',  ( -15.40903463028480580, 22.32187500034139660, 47.42413220539094709 ) ) ;
#7433=CARTESIAN_POINT ( 'NONE',  ( 49.86468353125000164, 30.85937500034139802, -6.106662507704105588E-15 ) ) ;
#7434=CARTESIAN_POINT ( 'NONE',  ( 15.45084971874737789, 26.38125000068280102, 47.55282581475767500 ) ) ;
#7435=CARTESIAN_POINT ( 'NONE',  ( -49.86468353124999453, 36.02187500034139589, 16.20201782572377169 ) ) ;
#7437=ADVANCED_FACE ( 'NONE', ( #10130 ), #11454, .T. ) ;
#7438=CARTESIAN_POINT ( 'NONE',  ( -15.45084971874737256, 37.60000000000000142, -47.55282581475767500 ) ) ;
#7439=CARTESIAN_POINT ( 'NONE',  ( 30.81806926056964002, 40.55937500034139731, 42.41743335407647209 ) ) ;
#7441=CARTESIAN_POINT ( 'NONE',  ( 15.45084971874736723, 43.39999999999999858, -47.55282581475768211 ) ) ;
#7448=DIRECTION ( 'NONE',  ( 0.000000000000000000, -0.000000000000000000, 1.000000000000000000 ) ) ;
#7450=CARTESIAN_POINT ( 'NONE',  ( 40.34137639590981905, 40.72187500034139873, 29.30972558990010768 ) ) ;
#7453=EDGE_CURVE ( 'NONE', #13275, #2321, #6260, .T. ) ;
#7454=CARTESIAN_POINT ( 'NONE',  ( -40.45084971874737079, 27.98125000068279888, 29.38926261462367151 ) ) ;
#7455=CARTESIAN_POINT ( 'NONE',  ( -40.34137639590981195, 36.12187500034139731, 29.30972558990012189 ) ) ;
#7464=CARTESIAN_POINT ( 'NONE',  ( -40.45084971874737789, 21.58125000068279675, -29.38926261462365730 ) ) ;
#7466=CARTESIAN_POINT ( 'NONE',  ( 15.40903463028482356, 30.45937500034139589, 47.42413220539093999 ) ) ;
#7472=ORIENTED_EDGE ( 'NONE', *, *, #12231, .F. ) ;
#7480=DIRECTION ( 'NONE',  ( -0.000000000000000000, 1.000000000000000000, -0.000000000000000000 ) ) ;
#7482=CARTESIAN_POINT ( 'NONE',  ( 40.45084971874737079, 32.98125000068279888, -29.38926261462366440 ) ) ;
#7486=( NAMED_UNIT ( * ) PLANE_ANGLE_UNIT ( ) SI_UNIT ( $, .RADIAN. ) );
#7488=CARTESIAN_POINT ( 'NONE',  ( -30.90169943749473802, 48.08125000068278609, 42.53254041760200721 ) ) ;
#7491=CARTESIAN_POINT ( 'NONE',  ( -15.40903463028480580, 20.25937500034139660, 47.42413220539094709 ) ) ;
#7495=CARTESIAN_POINT ( 'NONE',  ( 7.513064459987437071E-14, 42.28125000068280315, 50.00000000000000000 ) ) ;
#7499=( BOUNDED_CURVE ( )  B_SPLINE_CURVE ( 2, ( #7657, #1498, #3753, #12727, #11475, #10233, #15292, #10720, #12975, #7980, #5507, #400, #9146 ),
 .UNSPECIFIED., .F., .T. ) 
 B_SPLINE_CURVE_WITH_KNOTS ( ( 3, 2, 2, 2, 2, 2, 3 ),
 ( 0.08333333333333334259, 0.08666666666666666963, 0.09333333333333333759, 0.1000000000000000056, 0.1066666666666666735, 0.1133333333333333276, 0.1166666666666666685 ),
 .UNSPECIFIED. ) 
 CURVE ( )  GEOMETRIC_REPRESENTATION_ITEM ( )  RATIONAL_B_SPLINE_CURVE ( ( 0.9755282581475768211, 0.9755282581475768211, 1.000000000000000000, 0.9510565162951535312, 1.000000000000000000, 0.9510565162951535312, 1.000000000000000000, 0.9510565162951535312, 1.000000000000000000, 0.9510565162951535312, 1.000000000000000000, 0.9755282581475767101, 0.9755282581475768211 ) ) 
 REPRESENTATION_ITEM ( '' )  );
#7503=CARTESIAN_POINT ( 'NONE',  ( -40.34137639590981905, 21.72187500034139518, -29.30972558990011478 ) ) ;
#7504=CARTESIAN_POINT ( 'NONE',  ( -49.86468353125000164, 23.85937500034139447, 0.000000000000000000 ) ) ;
#7506=CARTESIAN_POINT ( 'NONE',  ( 15.40903463028481113, 35.32187500034139305, -47.42413220539094709 ) ) ;
#7508=CARTESIAN_POINT ( 'NONE',  ( 50.00000000000000711, 38.89999999999999858, 16.24598481164530739 ) ) ;
#7509=CARTESIAN_POINT ( 'NONE',  ( -30.81806926056963292, 39.55937500034139731, -42.41743335407647209 ) ) ;
#7513=CARTESIAN_POINT ( 'NONE',  ( -49.99999999999999289, 47.89999999999999858, -16.24598481164531449 ) ) ;
#7523=CARTESIAN_POINT ( 'NONE',  ( 40.34137639590981905, 42.72187500034139873, 29.30972558990010768 ) ) ;
#7525=EDGE_CURVE ( 'NONE', #14047, #15954, #14020, .T. ) ;
#7527=CARTESIAN_POINT ( 'NONE',  ( 50.00000000000000711, 30.68125000068279462, 16.24598481164530739 ) ) ;
#7528=CARTESIAN_POINT ( 'NONE',  ( 5.648665123217551098, 39.07342515812086248, 92.94044983197015597 ) ) ;
#7531=CARTESIAN_POINT ( 'NONE',  ( -15.40903463028480580, 36.32187500034140015, 47.42413220539094709 ) ) ;
#7544=CARTESIAN_POINT ( 'NONE',  ( 49.86468353124999453, 28.95937500034139944, -16.20201782572376459 ) ) ;
#7547=CARTESIAN_POINT ( 'NONE',  ( -49.86468353124999453, 46.02187500034139589, 16.20201782572377169 ) ) ;
#7550=CARTESIAN_POINT ( 'NONE',  ( -7.919222016226752814, 41.55125428154683931, -50.00000000000000711 ) ) ;
#7554=EDGE_LOOP ( 'NONE', ( #780, #876 ) ) ;
#7557=EDGE_CURVE ( 'NONE', #3318, #6257, #9963, .T. ) ;
#7563=CARTESIAN_POINT ( 'NONE',  ( 40.45084971874737789, 32.58125000068280031, 29.38926261462365375 ) ) ;
#7565=CARTESIAN_POINT ( 'NONE',  ( 15.45084971874736723, 25.18125000068279817, -47.55282581475768211 ) ) ;
#7568=CARTESIAN_POINT ( 'NONE',  ( -49.99999999999999289, 45.88125000068279746, 16.24598481164533226 ) ) ;
#7569=CARTESIAN_POINT ( 'NONE',  ( 30.90169943749473802, 21.30000000000000426, -42.53254041760200721 ) ) ;
#7571=CARTESIAN_POINT ( 'NONE',  ( -3.111920190527341144E-15, 25.50000000000000355, -50.00000000000000000 ) ) ;
#7580=ADVANCED_FACE ( 'NONE', ( #7793 ), #5326, .F. ) ;
#7581=CARTESIAN_POINT ( 'NONE',  ( 30.90169943749473802, 33.30000000000000426, -42.53254041760200721 ) ) ;
#7583=STYLED_ITEM ( 'NONE', ( #1074 ), #3231 ) ;
#7587=CARTESIAN_POINT ( 'NONE',  ( -30.81806926056962226, 20.15937500034140228, 42.41743335407647209 ) ) ;
#7589=CARTESIAN_POINT ( 'NONE',  ( 49.86468353125000164, 32.92187500034139447, -6.106662507704105588E-15 ) ) ;
#7591=CARTESIAN_POINT ( 'NONE',  ( 49.99999999999999289, 33.10000000000000853, -16.24598481164532160 ) ) ;
#7592=CARTESIAN_POINT ( 'NONE',  ( 49.86468353124999453, 36.95937500034139589, -16.20201782572376459 ) ) ;
#7596=AXIS2_PLACEMENT_3D ( 'NONE', #8665, #16312, #13810 ) ;
#7597=CARTESIAN_POINT ( 'NONE',  ( -40.45084971874737079, 42.20000000000000284, 29.38926261462367151 ) ) ;
#7599=CARTESIAN_POINT ( 'NONE',  ( -7.919222016226804328, 26.44874571845315359, 50.00000000000000000 ) ) ;
#7612=CARTESIAN_POINT ( 'NONE',  ( -15.40903463028481646, 45.52187500034139589, -47.42413220539093999 ) ) ;
#7615=CARTESIAN_POINT ( 'NONE',  ( 49.99999999999999289, 26.88125000068280102, -16.24598481164532160 ) ) ;
#7617=CARTESIAN_POINT ( 'NONE',  ( 15.40903463028481113, 33.32187500034139305, -47.42413220539094709 ) ) ;
#7620=AXIS2_PLACEMENT_3D ( 'NONE', #9816, #11151, #14867 ) ;
#7627=CYLINDRICAL_SURFACE ( 'NONE', #6613, 50.00000000000000000 ) ;
#7629=CARTESIAN_POINT ( 'NONE',  ( 40.34137639590981905, 28.65937500034139873, 29.30972558990010768 ) ) ;
#7634=CARTESIAN_POINT ( 'NONE',  ( -40.34137639590981905, 43.72187500034139873, -29.30972558990011478 ) ) ;
#7644=ORIENTED_EDGE ( 'NONE', *, *, #3672, .T. ) ;
#7647=CARTESIAN_POINT ( 'NONE',  ( 50.00000000000000000, 34.78125000068280315, -6.123233995736766085E-15 ) ) ;
#7655=CARTESIAN_POINT ( 'NONE',  ( -49.99999999999999289, 41.68125000068280173, -16.24598481164531449 ) ) ;
#7657=CARTESIAN_POINT ( 'NONE',  ( 2.978552182361884590E-14, 47.28125000068279604, -50.00000000000000000 ) ) ;
#7658=CARTESIAN_POINT ( 'NONE',  ( 8.446640517145639571E-15, 26.50000000000000000, 50.00000000000000000 ) ) ;
#7663=CARTESIAN_POINT ( 'NONE',  ( 30.90169943749473802, 43.08125000068280031, -42.53254041760200721 ) ) ;
#7667=ORIENTED_EDGE ( 'NONE', *, *, #7031, .T. ) ;
#7668=CARTESIAN_POINT ( 'NONE',  ( 49.99999999999999289, 33.10000000000000142, -16.24598481164532160 ) ) ;
#7669=CYLINDRICAL_SURFACE ( 'NONE', #943, 50.00000000000000000 ) ;
#7673=CARTESIAN_POINT ( 'NONE',  ( -49.86468353124999453, 25.95937500034139589, 16.20201782572377169 ) ) ;
#7675=CARTESIAN_POINT ( 'NONE',  ( -30.81806926056963292, 35.62187500034140442, -42.41743335407646498 ) ) ;
#7678=CARTESIAN_POINT ( 'NONE',  ( 40.45084971874737079, 31.20000000000000284, -29.38926261462366440 ) ) ;
#7679=CARTESIAN_POINT ( 'NONE',  ( -3.210462471511496205E-15, 37.35937500034139447, -52.43083105670540789 ) ) ;
#7681=CARTESIAN_POINT ( 'NONE',  ( 30.90169943749474157, 43.30000000000000426, -42.53254041760200721 ) ) ;
#7693=CARTESIAN_POINT ( 'NONE',  ( 40.34137639590981905, 44.72187500034139163, 29.30972558990010768 ) ) ;
#7694=CARTESIAN_POINT ( 'NONE',  ( 49.86468353124999453, 40.95937500034140299, -16.20201782572376104 ) ) ;
#7697=CARTESIAN_POINT ( 'NONE',  ( 15.45084971874737789, 26.38125000068280102, 47.55282581475767500 ) ) ;
#7698=CARTESIAN_POINT ( 'NONE',  ( 10.22617902976740822, 36.71297534007683794, 92.96698611470405638 ) ) ;
#7699=CONICAL_SURFACE ( 'NONE', #6380, 85.01963570546854498, 0.9599310885968793672 ) ;
#7700=CARTESIAN_POINT ( 'NONE',  ( 30.81806926056964002, 34.62187500034139731, 42.41743335407647209 ) ) ;
#7702=ORIENTED_EDGE ( 'NONE', *, *, #3975, .F. ) ;
#7703=ORIENTED_EDGE ( 'NONE', *, *, #4905, .T. ) ;
#7707=CARTESIAN_POINT ( 'NONE',  ( -30.90169943749474513, 23.48125000068279888, -42.53254041760200721 ) ) ;
#7709=CARTESIAN_POINT ( 'NONE',  ( -15.40903463028480580, 34.25937500034139305, 47.42413220539094709 ) ) ;
#7711=CARTESIAN_POINT ( 'NONE',  ( 49.86468353125000164, 48.92187500034139447, -6.106662507704105588E-15 ) ) ;
#7712=DIRECTION ( 'NONE',  ( 0.000000000000000000, -0.5735764363510476027, -0.8191520442889907994 ) ) ;
#7719=CARTESIAN_POINT ( 'NONE',  ( -3.111920190527341144E-15, 27.28125000068279604, -50.00000000000000000 ) ) ;
#7721=ORIENTED_EDGE ( 'NONE', *, *, #2441, .F. ) ;
#7733=CARTESIAN_POINT ( 'NONE',  ( 50.00000000000000000, 38.78125000068279604, -6.123233995736766085E-15 ) ) ;
#7741=CARTESIAN_POINT ( 'NONE',  ( -3.111920190527341144E-15, 43.28125000068280315, -50.00000000000000000 ) ) ;
#7746=CARTESIAN_POINT ( 'NONE',  ( 40.45084971874737079, 33.20000000000000284, -29.38926261462366440 ) ) ;
#7747=CARTESIAN_POINT ( 'NONE',  ( -16.62039348561838281, 28.09550434916130257, 93.58242969371653430 ) ) ;
#7751=CARTESIAN_POINT ( 'NONE',  ( 49.86468353125000164, 22.85937500034139802, -6.106662507704105588E-15 ) ) ;
#7753=CARTESIAN_POINT ( 'NONE',  ( -15.40903463028481646, 31.52187500034139944, -47.42413220539093999 ) ) ;
#7755=CARTESIAN_POINT ( 'NONE',  ( -30.90169943749474868, 29.70000000000000284, -42.53254041760200721 ) ) ;
#7756=CARTESIAN_POINT ( 'NONE',  ( -30.81806926056962226, 34.15937500034139163, 42.41743335407647919 ) ) ;
#7758=CARTESIAN_POINT ( 'NONE',  ( 15.45084971874736723, 41.40000000000000568, -47.55282581475768211 ) ) ;
#7762=VERTEX_POINT ( 'NONE', #8686 ) ;
#7770=CARTESIAN_POINT ( 'NONE',  ( 49.86468353125000164, 34.92187500034140157, -6.106662507704105588E-15 ) ) ;
#7771=CARTESIAN_POINT ( 'NONE',  ( -40.34137639590981195, 40.05937500034140442, 29.30972558990012189 ) ) ;
#7775=CARTESIAN_POINT ( 'NONE',  ( 15.45084971874736723, 25.18125000068279817, -47.55282581475768211 ) ) ;
#7776=CARTESIAN_POINT ( 'NONE',  ( 12.80943516814229532, 34.43714179323908553, 93.05110628388169403 ) ) ;
#7777=CARTESIAN_POINT ( 'NONE',  ( 49.86468353125001585, 28.82187500034139305, 16.20201782572375038 ) ) ;
#7780=ADVANCED_FACE ( 'NONE', ( #8936 ), #10269, .F. ) ;
#7790=CARTESIAN_POINT ( 'NONE',  ( -40.34137639590981905, 31.65937500034139873, -29.30972558990011478 ) ) ;
#7791=CARTESIAN_POINT ( 'NONE',  ( -49.86468353125000164, 43.92187500034140157, 0.000000000000000000 ) ) ;
#7793=FACE_OUTER_BOUND ( 'NONE', #9222, .T. ) ;
#7802=EDGE_LOOP ( 'NONE', ( #15975, #14946, #13498, #11708 ) ) ;
#7806=CARTESIAN_POINT ( 'NONE',  ( -30.90169943749473802, 22.30000000000000071, 42.53254041760200721 ) ) ;
#7809=CARTESIAN_POINT ( 'NONE',  ( -30.90169943749474513, 31.48125000068279533, -42.53254041760200721 ) ) ;
#7810=CARTESIAN_POINT ( 'NONE',  ( 15.45084971874737789, 24.38125000068279746, 47.55282581475767500 ) ) ;
#7811=CARTESIAN_POINT ( 'NONE',  ( 15.40903463028481113, 25.32187500034139660, -47.42413220539094709 ) ) ;
#7813=CARTESIAN_POINT ( 'NONE',  ( -40.45084971874737079, 37.98125000068279888, 29.38926261462367151 ) ) ;
#7831=CARTESIAN_POINT ( 'NONE',  ( -30.81806926056963292, 25.55937500034139376, -42.41743335407646498 ) ) ;
#7833=CARTESIAN_POINT ( 'NONE',  ( -3.210462471511496205E-15, 31.42187500034139447, -52.43083105670540789 ) ) ;
#7834=EDGE_CURVE ( 'NONE', #384, #6400, #6449, .T. ) ;
#7835=CARTESIAN_POINT ( 'NONE',  ( -49.99999999999999289, 22.09999999999999787, 16.24598481164533226 ) ) ;
#7836=EDGE_CURVE ( 'NONE', #4422, #4896, #9666, .T. ) ;
#7837=CARTESIAN_POINT ( 'NONE',  ( 30.90169943749475578, 32.70000000000000284, 42.53254041760200010 ) ) ;
#7838=CARTESIAN_POINT ( 'NONE',  ( 9.631387414534489405E-15, 30.35937500034139447, 52.43083105670540789 ) ) ;
#7850=CARTESIAN_POINT ( 'NONE',  ( 9.631387414534489405E-15, 34.42187500034138736, 52.43083105670540789 ) ) ;
#7851=CARTESIAN_POINT ( 'NONE',  ( 40.34137639590981905, 44.65937500034139163, 29.30972558990010768 ) ) ;
#7856=CARTESIAN_POINT ( 'NONE',  ( -30.90169943749473802, 22.08125000068279320, 42.53254041760200721 ) ) ;
#7858=CARTESIAN_POINT ( 'NONE',  ( -30.81806926056962226, 28.22187500034139873, 42.41743335407647919 ) ) ;
#7866=CARTESIAN_POINT ( 'NONE',  ( 40.45084971874737789, 48.58125000068280031, 29.38926261462365375 ) ) ;
#7870=CARTESIAN_POINT ( 'NONE',  ( 40.34137639590981905, 22.65937500034139518, 29.30972558990010768 ) ) ;
#7872=CARTESIAN_POINT ( 'NONE',  ( -30.81806926056963292, 45.62187500034139020, -42.41743335407646498 ) ) ;
#7876=CARTESIAN_POINT ( 'NONE',  ( -3.210462471511496205E-15, 45.42187500034139447, -52.43083105670540789 ) ) ;
#7887=CARTESIAN_POINT ( 'NONE',  ( 0.000000000000000000, 20.00000000000000355, 0.000000000000000000 ) ) ;
#7890=CARTESIAN_POINT ( 'NONE',  ( 40.45084971874737789, 24.80000000000000426, 29.38926261462365375 ) ) ;
#7891=CARTESIAN_POINT ( 'NONE',  ( 40.34137639590981905, 46.65937500034139873, 29.30972558990010768 ) ) ;
#7894=CARTESIAN_POINT ( 'NONE',  ( 15.40903463028481113, 21.32187500034139660, -47.42413220539094709 ) ) ;
#7897=CARTESIAN_POINT ( 'NONE',  ( 50.00000000000000000, 40.78125000068279604, -6.123233995736766085E-15 ) ) ;
#7899=CARTESIAN_POINT ( 'NONE',  ( 50.00000000000000000, 22.78125000068279959, -6.123233995736766085E-15 ) ) ;
#7901=ORIENTED_EDGE ( 'NONE', *, *, #5909, .T. ) ;
#7903=ORIENTED_EDGE ( 'NONE', *, *, #14133, .F. ) ;
#7909=CARTESIAN_POINT ( 'NONE',  ( -12.00394982932901655, 35.24696676550272656, 93.01447361572049033 ) ) ;
#7912=EDGE_CURVE ( 'NONE', #15952, #2027, #10738, .T. ) ;
#7914=EDGE_CURVE ( 'NONE', #10580, #3182, #4371, .T. ) ;
#7915=CARTESIAN_POINT ( 'NONE',  ( 7.919222016226827421, 47.44874571845315359, -50.00000000000000000 ) ) ;
#7916=CARTESIAN_POINT ( 'NONE',  ( -48.34710198928235059, 20.00000000000000355, 12.20844498793695365 ) ) ;
#7917=CARTESIAN_POINT ( 'NONE',  ( 30.81806926056964002, 30.62187500034139376, 42.41743335407646498 ) ) ;
#7919=CARTESIAN_POINT ( 'NONE',  ( -40.45084971874737789, 29.80000000000000071, -29.38926261462365730 ) ) ;
#7920=CARTESIAN_POINT ( 'NONE',  ( -49.86468353124999453, 33.95937500034139589, 16.20201782572377525 ) ) ;
#7922=CARTESIAN_POINT ( 'NONE',  ( 50.00000000000000000, 39.00000000000000000, -6.123233995736766085E-15 ) ) ;
#7925=PRODUCT_DEFINITION_CONTEXT ( 'detailed design', #6668, 'design' ) ;
#7928=ADVANCED_FACE ( 'NONE', ( #14698 ), #2863, .F. ) ;
#7935=CARTESIAN_POINT ( 'NONE',  ( -3.210462471511496205E-15, 33.42187500034140157, -52.43083105670540789 ) ) ;
#7936=CARTESIAN_POINT ( 'NONE',  ( 49.86468353125000164, 38.85937500034139447, -6.106662507704105588E-15 ) ) ;
#7939=CARTESIAN_POINT ( 'NONE',  ( 15.40903463028481113, 49.25937500034139305, -47.42413220539094709 ) ) ;
#7942=CARTESIAN_POINT ( 'NONE',  ( -30.81806926056962226, 26.22187500034139518, 42.41743335407647919 ) ) ;
#7944=CARTESIAN_POINT ( 'NONE',  ( -50.00000000000000000, 27.78125000068279959, 0.000000000000000000 ) ) ;
#7949=CARTESIAN_POINT ( 'NONE',  ( 7.919222016226818539, 49.22999571913594252, -50.00000000000000000 ) ) ;
#7954=CARTESIAN_POINT ( 'NONE',  ( 30.81806926056962936, 23.15937500034139873, -42.41743335407647209 ) ) ;
#7956=CARTESIAN_POINT ( 'NONE',  ( 49.86468353125000164, 42.92187500034140157, -6.106662507704105588E-15 ) ) ;
#7959=CARTESIAN_POINT ( 'NONE',  ( 15.40903463028482356, 48.52187500034140299, 47.42413220539093999 ) ) ;
#7961=ORIENTED_EDGE ( 'NONE', *, *, #12301, .F. ) ;
#7971=LINE ( 'NONE', #13043, #15657 ) ;
#7972=CARTESIAN_POINT ( 'NONE',  ( 49.99999999999999289, 25.10000000000000142, -16.24598481164532160 ) ) ;
#7973=CARTESIAN_POINT ( 'NONE',  ( -40.34137639590981905, 41.65937500034139873, -29.30972558990011478 ) ) ;
#7978=CARTESIAN_POINT ( 'NONE',  ( -40.45084971874737789, 43.58125000068280031, -29.38926261462365730 ) ) ;
#7980=CARTESIAN_POINT ( 'NONE',  ( 30.90169943749475223, 46.48125000068280599, 42.53254041760199300 ) ) ;
#7982=ORIENTED_EDGE ( 'NONE', *, *, #496, .F. ) ;
#7986=CARTESIAN_POINT ( 'NONE',  ( 15.45084971874736723, 43.39999999999999858, -47.55282581475768211 ) ) ;
#7991=DIRECTION ( 'NONE',  ( -0.000000000000000000, -0.000000000000000000, -1.000000000000000000 ) ) ;
#7993=CARTESIAN_POINT ( 'NONE',  ( 0.000000000000000000, 20.00000000000000355, 0.000000000000000000 ) ) ;
#7997=CARTESIAN_POINT ( 'NONE',  ( -46.31917516190693362, 20.00000000000000355, 18.46674513801226425 ) ) ;
#7998=CARTESIAN_POINT ( 'NONE',  ( -49.86468353125000164, 27.92187500034139447, 0.000000000000000000 ) ) ;
#8001=CARTESIAN_POINT ( 'NONE',  ( -3.210462471511496205E-15, 31.35937500034139092, -52.43083105670540789 ) ) ;
#8009=DIRECTION ( 'NONE',  ( 0.000000000000000000, 1.000000000000000000, 0.000000000000000000 ) ) ;
#8012=CARTESIAN_POINT ( 'NONE',  ( -49.86468353124999453, 36.02187500034139589, 16.20201782572377525 ) ) ;
#8013=CARTESIAN_POINT ( 'NONE',  ( 49.86468353125000164, 34.85937500034140157, -6.106662507704105588E-15 ) ) ;
#8016=CARTESIAN_POINT ( 'NONE',  ( -40.45084971874737789, 23.58125000068280031, -29.38926261462365730 ) ) ;
#8018=CARTESIAN_POINT ( 'NONE',  ( 49.86468353124999453, 25.02187500034139589, -16.20201782572376459 ) ) ;
#8021=ORIENTED_EDGE ( 'NONE', *, *, #5809, .F. ) ;
#8023=ORIENTED_EDGE ( 'NONE', *, *, #3983, .T. ) ;
#8030=CARTESIAN_POINT ( 'NONE',  ( -49.86468353125000164, 27.85937500034139447, 0.000000000000000000 ) ) ;
#8032=CARTESIAN_POINT ( 'NONE',  ( 30.81806926056964002, 40.62187500034139731, 42.41743335407646498 ) ) ;
#8034=EDGE_CURVE ( 'NONE', #1788, #4999, #2772, .T. ) ;
#8036=CARTESIAN_POINT ( 'NONE',  ( -30.81806926056963292, 45.62187500034139020, -42.41743335407647209 ) ) ;
#8047=FACE_OUTER_BOUND ( 'NONE', #13198, .T. ) ;
#8048=CARTESIAN_POINT ( 'NONE',  ( 50.00000000000000000, 25.00000000000000000, -6.123233995736766085E-15 ) ) ;
#8049=CARTESIAN_POINT ( 'NONE',  ( -49.86468353124999453, 45.95937500034138878, 16.20201782572377525 ) ) ;
#8050=CARTESIAN_POINT ( 'NONE',  ( -40.45084971874737789, 25.58125000068279675, -29.38926261462365730 ) ) ;
#8055=CARTESIAN_POINT ( 'NONE',  ( 15.45084971874736723, 33.18125000068279462, -47.55282581475768211 ) ) ;
#8070=CARTESIAN_POINT ( 'NONE',  ( 50.00000000000000000, 23.00000000000000355, -6.123233995736766085E-15 ) ) ;
#8074=CARTESIAN_POINT ( 'NONE',  ( 17.50000000000000000, 22.50000000000000355, 94.42467108177066848 ) ) ;
#8075=CARTESIAN_POINT ( 'NONE',  ( -47.55097084096128413, 20.00000000000001066, 15.01398062573002612 ) ) ;
#8077=CARTESIAN_POINT ( 'NONE',  ( 9.631387414534489405E-15, 26.42187500034139447, 52.43083105670540789 ) ) ;
#8078=CARTESIAN_POINT ( 'NONE',  ( -50.00000000000000000, 22.00000000000000355, 0.000000000000000000 ) ) ;
#8081=CARTESIAN_POINT ( 'NONE',  ( -30.81806926056962226, 32.15937500034139873, 42.41743335407647919 ) ) ;
#8093=CARTESIAN_POINT ( 'NONE',  ( 49.86468353125000164, 36.92187500034140157, -6.106662507704105588E-15 ) ) ;
#8094=CARTESIAN_POINT ( 'NONE',  ( 15.40903463028482356, 38.45937500034139589, 47.42413220539093999 ) ) ;
#8097=CARTESIAN_POINT ( 'NONE',  ( 40.45084971874737789, 22.58125000068279675, 29.38926261462365375 ) ) ;
#8100=CARTESIAN_POINT ( 'NONE',  ( 15.40903463028481113, 25.32187500034139660, -47.42413220539094709 ) ) ;
#8105=VECTOR ( 'NONE', #9692, 1000.000000000000000 ) ;
#8108=CARTESIAN_POINT ( 'NONE',  ( 40.45084971874737789, 30.58125000068279675, 29.38926261462365375 ) ) ;
#8110=CARTESIAN_POINT ( 'NONE',  ( 30.81806926056962936, 27.15937500034139163, -42.41743335407647209 ) ) ;
#8113=CARTESIAN_POINT ( 'NONE',  ( 40.34137639590981905, 40.72187500034139873, 29.30972558990010768 ) ) ;
#8116=CARTESIAN_POINT ( 'NONE',  ( -49.86468353124999453, 46.02187500034140299, 16.20201782572377525 ) ) ;
#8118=CARTESIAN_POINT ( 'NONE',  ( 50.00000000000000000, 31.00000000000000355, -6.123233995736766085E-15 ) ) ;
#8127=ORIENTED_EDGE ( 'NONE', *, *, #9559, .T. ) ;
#8129=EDGE_CURVE ( 'NONE', #2703, #14669, #11065, .T. ) ;
#8132=EDGE_CURVE ( 'NONE', #11630, #8883, #1698, .T. ) ;
#8134=CARTESIAN_POINT ( 'NONE',  ( 40.45084971874737079, 27.20000000000000284, -29.38926261462366440 ) ) ;
#8136=CARTESIAN_POINT ( 'NONE',  ( 49.86468353125000164, 44.85937500034140157, -6.106662507704105588E-15 ) ) ;
#8141=AXIS2_PLACEMENT_3D ( 'NONE', #591, #3262, #11749 ) ;
#8144=CARTESIAN_POINT ( 'NONE',  ( 0.000000000000000000, 20.00000000000000355, 50.00000000000000000 ) ) ;
#8145=CARTESIAN_POINT ( 'NONE',  ( -50.00000000000000000, 33.78125000068280315, 0.000000000000000000 ) ) ;
#8147=CARTESIAN_POINT ( 'NONE',  ( 40.45084971874737789, 20.58125000068280031, 29.38926261462365375 ) ) ;
#8152=VECTOR ( 'NONE', #13741, 1000.000000000000000 ) ;
#8156=CARTESIAN_POINT ( 'NONE',  ( 50.00000000000000000, 43.00000000000000000, -6.123233995736766085E-15 ) ) ;
#8157=DIRECTION ( 'NONE',  ( 0.000000000000000000, 0.000000000000000000, 1.000000000000000000 ) ) ;
#8161=CARTESIAN_POINT ( 'NONE',  ( 40.45084971874737789, 22.80000000000000071, 29.38926261462365375 ) ) ;
#8166=CARTESIAN_POINT ( 'NONE',  ( 40.45084971874737079, 47.20000000000000284, -29.38926261462366440 ) ) ;
#8167=CARTESIAN_POINT ( 'NONE',  ( -47.88920767661647204, 19.99999999999999645, 13.89741811465869503 ) ) ;
#8168=CARTESIAN_POINT ( 'NONE',  ( -3.210462471511496205E-15, 23.42187500034139447, -52.43083105670540789 ) ) ;
#8170=CARTESIAN_POINT ( 'NONE',  ( -30.90169943749473447, 22.29999999999999716, 42.53254041760200721 ) ) ;
#8172=CARTESIAN_POINT ( 'NONE',  ( -40.34137639590981905, 25.65937500034139518, -29.30972558990011478 ) ) ;
#8173=EDGE_CURVE ( 'NONE', #4002, #9078, #825, .T. ) ;
#8183=CARTESIAN_POINT ( 'NONE',  ( 9.631387414534489405E-15, 32.42187500034139447, 52.43083105670540789 ) ) ;
#8184=CARTESIAN_POINT ( 'NONE',  ( -30.81806926056963292, 35.55937500034139020, -42.41743335407646498 ) ) ;
#8189=CARTESIAN_POINT ( 'NONE',  ( 40.45084971874737079, 20.98125000068279888, -29.38926261462366440 ) ) ;
#8191=CARTESIAN_POINT ( 'NONE',  ( 49.86468353125001585, 20.82187500034140015, 16.20201782572375038 ) ) ;
#8194=ORIENTED_EDGE ( 'NONE', *, *, #8034, .F. ) ;
#8198=CYLINDRICAL_SURFACE ( 'NONE', #7596, 50.00000000000000000 ) ;
#8201=CARTESIAN_POINT ( 'NONE',  ( 49.86468353124999453, 22.95937500034139589, -16.20201782572376459 ) ) ;
#8204=CARTESIAN_POINT ( 'NONE',  ( 40.45084971874737079, 35.20000000000000284, -29.38926261462366440 ) ) ;
#8205=CARTESIAN_POINT ( 'NONE',  ( -49.86468353125000164, 49.92187500034140157, 0.000000000000000000 ) ) ;
#8215=CARTESIAN_POINT ( 'NONE',  ( 49.99999999999999289, 21.09999999999999787, -16.24598481164532160 ) ) ;
#8217=CARTESIAN_POINT ( 'NONE',  ( -40.34137639590981195, 44.05937500034139731, 29.30972558990012189 ) ) ;
#8218=CARTESIAN_POINT ( 'NONE',  ( -49.86468353125000164, 49.85937500034139447, 0.000000000000000000 ) ) ;
#8237=FACE_OUTER_BOUND ( 'NONE', #11064, .T. ) ;
#8242=CARTESIAN_POINT ( 'NONE',  ( -49.99999999999999289, 48.09999999999999432, 16.24598481164533226 ) ) ;
#8249=CARTESIAN_POINT ( 'NONE',  ( -49.86468353125000164, 23.85937500034139447, 0.000000000000000000 ) ) ;
#8252=ADVANCED_FACE ( 'NONE', ( #10119 ), #5226, .T. ) ;
#8261=CARTESIAN_POINT ( 'NONE',  ( 40.34137639590981195, 27.12187500034139731, -29.30972558990011834 ) ) ;
#8262=CARTESIAN_POINT ( 'NONE',  ( 30.81806926056964002, 34.55937500034139731, 42.41743335407646498 ) ) ;
#8263=CARTESIAN_POINT ( 'NONE',  ( -49.99999999999999289, 44.09999999999999432, 16.24598481164533226 ) ) ;
#8266=CARTESIAN_POINT ( 'NONE',  ( 30.81806926056964002, 44.55937500034139020, 42.41743335407647209 ) ) ;
#8268=CARTESIAN_POINT ( 'NONE',  ( 15.45084971874737789, 48.60000000000000142, 47.55282581475767500 ) ) ;
#8273=ORIENTED_EDGE ( 'NONE', *, *, #6942, .F. ) ;
#8278=CARTESIAN_POINT ( 'NONE',  ( 49.86468353125001585, 46.82187500034139305, 16.20201782572375038 ) ) ;
#8281=CARTESIAN_POINT ( 'NONE',  ( 40.45084971874737789, 40.80000000000000426, 29.38926261462365375 ) ) ;
#8282=CARTESIAN_POINT ( 'NONE',  ( 15.40903463028482356, 38.52187500034139589, 47.42413220539093999 ) ) ;
#8283=CARTESIAN_POINT ( 'NONE',  ( 15.45084971874737789, 30.60000000000000142, 47.55282581475767500 ) ) ;
#8288=EDGE_CURVE ( 'NONE', #10597, #15517, #11372, .T. ) ;
#8291=DIRECTION ( 'NONE',  ( 1.000000000000000000, -0.000000000000000000, -0.000000000000000000 ) ) ;
#8293=CARTESIAN_POINT ( 'NONE',  ( -30.90169943749473802, 20.30000000000000426, 42.53254041760200721 ) ) ;
#8294=CARTESIAN_POINT ( 'NONE',  ( -40.34137639590981195, 40.05937500034140442, 29.30972558990012189 ) ) ;
#8301=CARTESIAN_POINT ( 'NONE',  ( -49.99999999999999289, 46.09999999999999432, 16.24598481164533226 ) ) ;
#8303=CARTESIAN_POINT ( 'NONE',  ( 40.45084971874737079, 41.20000000000000284, -29.38926261462366440 ) ) ;
#8311=CARTESIAN_POINT ( 'NONE',  ( 0.000000000000000000, 20.00000000000000355, 0.000000000000000000 ) ) ;
#8319=CARTESIAN_POINT ( 'NONE',  ( -49.99999999999999289, 31.89999999999999858, -16.24598481164531449 ) ) ;
#8322=CARTESIAN_POINT ( 'NONE',  ( -30.81806926056962226, 22.22187500034139163, 42.41743335407647209 ) ) ;
#8325=CARTESIAN_POINT ( 'NONE',  ( 30.81806926056962936, 25.15937500034139518, -42.41743335407647209 ) ) ;
#8328=ORIENTED_EDGE ( 'NONE', *, *, #12849, .F. ) ;
#8331=ORIENTED_EDGE ( 'NONE', *, *, #16259, .F. ) ;
#8339=CARTESIAN_POINT ( 'NONE',  ( 40.34137639590981905, 30.72187500034139518, 29.30972558990010768 ) ) ;
#8340=CARTESIAN_POINT ( 'NONE',  ( -15.40903463028481646, 31.45937500034139944, -47.42413220539093999 ) ) ;
#8341=FACE_OUTER_BOUND ( 'NONE', #567, .T. ) ;
#8344=CARTESIAN_POINT ( 'NONE',  ( -15.40903463028480580, 46.25937500034140015, 47.42413220539094709 ) ) ;
#8346=CARTESIAN_POINT ( 'NONE',  ( 49.86468353125000164, 20.92187500034139802, -6.106662507704105588E-15 ) ) ;
#8351=ORIENTED_EDGE ( 'NONE', *, *, #7340, .T. ) ;
#8356=CARTESIAN_POINT ( 'NONE',  ( -40.34137639590981905, 49.72187500034139873, -29.30972558990011478 ) ) ;
#8360=CARTESIAN_POINT ( 'NONE',  ( -49.99999999999999289, 36.10000000000000853, 16.24598481164533226 ) ) ;
#8361=CARTESIAN_POINT ( 'NONE',  ( -49.86468353124999453, 40.02187500034140299, 16.20201782572377525 ) ) ;
#8370=CARTESIAN_POINT ( 'NONE',  ( 8.446640517145639571E-15, 48.49999999999999289, 50.00000000000000000 ) ) ;
#8372=CARTESIAN_POINT ( 'NONE',  ( 50.00000000000000711, 36.68125000068280173, 16.24598481164530739 ) ) ;
#8373=CARTESIAN_POINT ( 'NONE',  ( 30.81806926056964002, 40.55937500034139731, 42.41743335407647209 ) ) ;
#8374=CARTESIAN_POINT ( 'NONE',  ( 30.81806926056962936, 47.15937500034139163, -42.41743335407646498 ) ) ;
#8379=LINE ( 'NONE', #5898, #6485 ) ;
#8380=CARTESIAN_POINT ( 'NONE',  ( -30.90169943749473447, 36.08125000068279320, 42.53254041760200721 ) ) ;
#8384=CARTESIAN_POINT ( 'NONE',  ( 0.000000000000000000, 28.00000000000000355, 0.000000000000000000 ) ) ;
#8385=PRODUCT_DEFINITION_FORMATION_WITH_SPECIFIED_SOURCE ( 'ANY', '', #1877, .NOT_KNOWN. ) ;
#8390=ORIENTED_EDGE ( 'NONE', *, *, #1427, .T. ) ;
#8399=CARTESIAN_POINT ( 'NONE',  ( -3.111920190527341144E-15, 45.28125000068279604, -50.00000000000000000 ) ) ;
#8402=DIRECTION ( 'NONE',  ( 1.000000000000000000, -0.000000000000000000, -0.000000000000000000 ) ) ;
#8404=CARTESIAN_POINT ( 'NONE',  ( -40.45084971874737789, 31.80000000000000071, -29.38926261462365730 ) ) ;
#8406=CARTESIAN_POINT ( 'NONE',  ( -46.13167797950591620, 20.00000000000000355, 18.93026546213454608 ) ) ;
#8407=CARTESIAN_POINT ( 'NONE',  ( -30.81806926056963292, 23.62187500034139731, -42.41743335407646498 ) ) ;
#8409=AXIS2_PLACEMENT_3D ( 'NONE', #10251, #2430, #2511 ) ;
#8411=CARTESIAN_POINT ( 'NONE',  ( 49.86468353125001585, 24.75937500034140015, 16.20201782572375038 ) ) ;
#8418=CARTESIAN_POINT ( 'NONE',  ( 30.90169943749475223, 48.69999999999999574, 42.53254041760199300 ) ) ;
#8420=EDGE_CURVE ( 'NONE', #13132, #102, #9241, .T. ) ;
#8424=CARTESIAN_POINT ( 'NONE',  ( 30.90169943749475223, 34.70000000000000284, 42.53254041760199300 ) ) ;
#8427=CARTESIAN_POINT ( 'NONE',  ( -30.81806926056962226, 30.22187500034139518, 42.41743335407647919 ) ) ;
#8428=CARTESIAN_POINT ( 'NONE',  ( -30.81806926056962226, 30.15937500034139163, 42.41743335407647209 ) ) ;
#8431=CARTESIAN_POINT ( 'NONE',  ( 30.81806926056962936, 43.15937500034140584, -42.41743335407647209 ) ) ;
#8433=CARTESIAN_POINT ( 'NONE',  ( -50.00000000000000000, 50.00000000000000000, 0.000000000000000000 ) ) ;
#8443=CARTESIAN_POINT ( 'NONE',  ( 49.86468353125001585, 20.75937500034140015, 16.20201782572375038 ) ) ;
#8444=LINE ( 'NONE', #12264, #10765 ) ;
#8447=CARTESIAN_POINT ( 'NONE',  ( 40.45084971874737789, 36.58125000068280031, 29.38926261462365375 ) ) ;
#8448=CARTESIAN_POINT ( 'NONE',  ( 30.90169943749475578, 38.70000000000000284, 42.53254041760200010 ) ) ;
#8449=CARTESIAN_POINT ( 'NONE',  ( -15.40903463028481646, 39.52187500034139589, -47.42413220539093999 ) ) ;
#8457=EDGE_CURVE ( 'NONE', #12470, #7298, #14745, .T. ) ;
#8461=CARTESIAN_POINT ( 'NONE',  ( 1.022488062601840571E-14, 49.28125000068280315, -50.00000000000000000 ) ) ;
#8462=CARTESIAN_POINT ( 'NONE',  ( 0.000000000000000000, 20.00000000000000355, 0.000000000000000000 ) ) ;
#8463=CARTESIAN_POINT ( 'NONE',  ( 40.34137639590981905, 40.65937500034139873, 29.30972558990010768 ) ) ;
#8464=CARTESIAN_POINT ( 'NONE',  ( 40.34137639590981905, 46.65937500034139873, 29.30972558990010768 ) ) ;
#8469=CARTESIAN_POINT ( 'NONE',  ( 7.919222016226758143, 40.55125428154685352, 50.00000000000000711 ) ) ;
#8481=CARTESIAN_POINT ( 'NONE',  ( 0.000000000000000000, 20.00000000000000355, 50.00000000000000000 ) ) ;
#8482=CARTESIAN_POINT ( 'NONE',  ( -15.45084971874736368, 20.40000000000000213, 47.55282581475768211 ) ) ;
#8492=CARTESIAN_POINT ( 'NONE',  ( -30.81806926056963292, 27.55937500034139376, -42.41743335407647209 ) ) ;
#8494=CARTESIAN_POINT ( 'NONE',  ( -49.99999999999999289, 30.10000000000000497, 16.24598481164533226 ) ) ;
#8496=CARTESIAN_POINT ( 'NONE',  ( 40.45084971874737789, 44.79999999999999716, 29.38926261462365375 ) ) ;
#8503=CARTESIAN_POINT ( 'NONE',  ( 7.919222016226822092, 28.33250428222963890, 49.99999999999999289 ) ) ;
#8505=CARTESIAN_POINT ( 'NONE',  ( -40.34137639590981195, 30.12187500034139731, 29.30972558990012189 ) ) ;
#8506=CARTESIAN_POINT ( 'NONE',  ( -49.86468353124999453, 31.95937500034139944, 16.20201782572377169 ) ) ;
#8507=CARTESIAN_POINT ( 'NONE',  ( 1.022488062601840571E-14, 49.50000000000000711, -50.00000000000000000 ) ) ;
#8509=CARTESIAN_POINT ( 'NONE',  ( 0.000000000000000000, 0.000000000000000000, 0.000000000000000000 ) ) ;
#8510=CARTESIAN_POINT ( 'NONE',  ( -15.40903463028480580, 44.25937500034140015, 47.42413220539094709 ) ) ;
#8512=CARTESIAN_POINT ( 'NONE',  ( 40.34137639590981195, 21.12187500034139376, -29.30972558990011834 ) ) ;
#8520=CARTESIAN_POINT ( 'NONE',  ( -15.40903463028481646, 49.52187500034140299, -47.42413220539093999 ) ) ;
#8522=CARTESIAN_POINT ( 'NONE',  ( -30.90169943749473802, 36.08125000068280031, 42.53254041760200721 ) ) ;
#8523=CARTESIAN_POINT ( 'NONE',  ( -15.40903463028480580, 42.32187500034139305, 47.42413220539094709 ) ) ;
#8531=CARTESIAN_POINT ( 'NONE',  ( -7.919222016226752814, 39.33250428222963535, -50.00000000000000711 ) ) ;
#8535=CARTESIAN_POINT ( 'NONE',  ( -15.40903463028481646, 35.45937500034139589, -47.42413220539093999 ) ) ;
#8542=CARTESIAN_POINT ( 'NONE',  ( 40.45084971874737079, 37.20000000000000284, -29.38926261462366440 ) ) ;
#8543=CARTESIAN_POINT ( 'NONE',  ( -49.99999999999999289, 41.90000000000000568, -16.24598481164531449 ) ) ;
#8544=EDGE_LOOP ( 'NONE', ( #6340, #5718, #11012, #2720 ) ) ;
#8548=ORIENTED_EDGE ( 'NONE', *, *, #7525, .T. ) ;
#8550=CYLINDRICAL_SURFACE ( 'NONE', #1504, 50.00000000000000000 ) ;
#8554=CARTESIAN_POINT ( 'NONE',  ( -11.62776035141319397, 9.371681691055611552, 97.66124091237762173 ) ) ;
#8555=CARTESIAN_POINT ( 'NONE',  ( 0.000000000000000000, 0.000000000000000000, 100.0000000000000000 ) ) ;
#8560=DIRECTION ( 'NONE',  ( 1.000000000000000000, 0.000000000000000000, 0.000000000000000000 ) ) ;
#8562=CARTESIAN_POINT ( 'NONE',  ( -3.219174618344376363E-15, 49.28125000068278894, -52.57311121191334990 ) ) ;
#8565=CARTESIAN_POINT ( 'NONE',  ( 40.34137639590981195, 21.05937500034139376, -29.30972558990011834 ) ) ;
#8566=CARTESIAN_POINT ( 'NONE',  ( -30.90169943749474513, 41.48125000068279178, -42.53254041760200721 ) ) ;
#8568=ORIENTED_EDGE ( 'NONE', *, *, #16259, .T. ) ;
#8571=CARTESIAN_POINT ( 'NONE',  ( 50.00000000000000711, 48.90000000000000568, 16.24598481164530739 ) ) ;
#8575=CARTESIAN_POINT ( 'NONE',  ( 30.90169943749473802, 35.29999999999999716, -42.53254041760200721 ) ) ;
#8576=CARTESIAN_POINT ( 'NONE',  ( -15.40903463028480580, 26.32187500034140015, 47.42413220539094709 ) ) ;
#8577=CARTESIAN_POINT ( 'NONE',  ( 15.40903463028482356, 30.45937500034139589, 47.42413220539093999 ) ) ;
#8578=CARTESIAN_POINT ( 'NONE',  ( 49.99999999999999289, 26.88125000068280102, -16.24598481164532160 ) ) ;
#8579=CARTESIAN_POINT ( 'NONE',  ( 49.86468353125000164, 34.92187500034140157, -6.106662507704105588E-15 ) ) ;
#8581=AXIS2_PLACEMENT_3D ( 'NONE', #13305, #14620, #2155 ) ;
#8582=CARTESIAN_POINT ( 'NONE',  ( -49.86468353124999453, 43.95937500034138878, 16.20201782572377525 ) ) ;
#8584=CARTESIAN_POINT ( 'NONE',  ( -49.99999999999999289, 46.09999999999999432, 16.24598481164533226 ) ) ;
#8587=ORIENTED_EDGE ( 'NONE', *, *, #5123, .T. ) ;
#8595=CARTESIAN_POINT ( 'NONE',  ( 49.86468353125000164, 48.92187500034139447, -6.106662507704105588E-15 ) ) ;
#8596=DIRECTION ( 'NONE',  ( -0.000000000000000000, 1.000000000000000000, -0.000000000000000000 ) ) ;
#8598=CARTESIAN_POINT ( 'NONE',  ( 30.90169943749475578, 34.48125000068279888, 42.53254041760200010 ) ) ;
#8599=CARTESIAN_POINT ( 'NONE',  ( -30.81806926056962226, 40.22187500034139873, 42.41743335407647919 ) ) ;
#8611=CARTESIAN_POINT ( 'NONE',  ( 30.90169943749475223, 26.70000000000000284, 42.53254041760199300 ) ) ;
#8613=CARTESIAN_POINT ( 'NONE',  ( -15.40903463028481646, 39.45937500034139589, -47.42413220539093999 ) ) ;
#8614=CARTESIAN_POINT ( 'NONE',  ( -40.34137639590981195, 44.05937500034139731, 29.30972558990012189 ) ) ;
#8634=EDGE_LOOP ( 'NONE', ( #2204, #4413, #11059, #2764, #1956, #3921 ) ) ;
#8635=CARTESIAN_POINT ( 'NONE',  ( -49.99999999999999289, 47.88125000068281167, 16.24598481164533226 ) ) ;
#8646=CARTESIAN_POINT ( 'NONE',  ( 49.99999999999999289, 48.88125000068279746, -16.24598481164532160 ) ) ;
#8650=CARTESIAN_POINT ( 'NONE',  ( 30.81806926056962936, 21.15937500034140228, -42.41743335407647209 ) ) ;
#8663=ADVANCED_FACE ( 'NONE', ( #11480 ), #15300, .F. ) ;
#8665=CARTESIAN_POINT ( 'NONE',  ( 0.000000000000000000, 20.00000000000000355, 0.000000000000000000 ) ) ;
#8668=CARTESIAN_POINT ( 'NONE',  ( 40.34137639590981195, 23.12187500034139731, -29.30972558990011834 ) ) ;
#8669=CARTESIAN_POINT ( 'NONE',  ( -15.40903463028480580, 32.25937500034140015, 47.42413220539094709 ) ) ;
#8673=CARTESIAN_POINT ( 'NONE',  ( 30.81806926056962936, 37.22187500034139163, -42.41743335407646498 ) ) ;
#8676=DIRECTION ( 'NONE',  ( -0.000000000000000000, 1.000000000000000000, -0.000000000000000000 ) ) ;
#8677=CARTESIAN_POINT ( 'NONE',  ( 40.34137639590981905, 40.65937500034139873, 29.30972558990010768 ) ) ;
#8679=CARTESIAN_POINT ( 'NONE',  ( 30.90169943749474157, 45.29999999999999005, -42.53254041760200721 ) ) ;
#8686=CARTESIAN_POINT ( 'NONE',  ( -2.547328955960238000E-13, 24.49999999999999289, 49.99999999999999289 ) ) ;
#8688=CARTESIAN_POINT ( 'NONE',  ( 30.81806926056962936, 45.22187500034139873, -42.41743335407647209 ) ) ;
#8691=CARTESIAN_POINT ( 'NONE',  ( 40.45084971874737079, 24.98125000068279888, -29.38926261462366440 ) ) ;
#8693=CARTESIAN_POINT ( 'NONE',  ( 40.34137639590981195, 33.12187500034139731, -29.30972558990011834 ) ) ;
#8697=ORIENTED_EDGE ( 'NONE', *, *, #16177, .T. ) ;
#8703=CARTESIAN_POINT ( 'NONE',  ( -40.45084971874737789, 49.58125000068280031, -29.38926261462365730 ) ) ;
#8705=EDGE_CURVE ( 'NONE', #13696, #4877, #617, .T. ) ;
#8706=CARTESIAN_POINT ( 'NONE',  ( 15.40903463028481113, 33.25937500034140015, -47.42413220539094709 ) ) ;
#8707=CARTESIAN_POINT ( 'NONE',  ( 30.81806926056962936, 45.15937500034139873, -42.41743335407646498 ) ) ;
#8711=DIRECTION ( 'NONE',  ( -0.000000000000000000, -0.000000000000000000, -1.000000000000000000 ) ) ;
#8721=VERTEX_POINT ( 'NONE', #12656 ) ;
#8725=CARTESIAN_POINT ( 'NONE',  ( -40.45084971874737079, 20.20000000000000284, 29.38926261462367151 ) ) ;
#8732=CARTESIAN_POINT ( 'NONE',  ( 15.45084971874736723, 49.18125000068279462, -47.55282581475768211 ) ) ;
#8733=CARTESIAN_POINT ( 'NONE',  ( 49.99999999999999289, 44.88125000068279036, -16.24598481164532160 ) ) ;
#8741=VERTEX_POINT ( 'NONE', #5103 ) ;
#8745=CARTESIAN_POINT ( 'NONE',  ( -15.45084971874736368, 20.18125000068279817, 47.55282581475768211 ) ) ;
#8749=ADVANCED_FACE ( 'NONE', ( #2995 ), #11971, .F. ) ;
#8751=CARTESIAN_POINT ( 'NONE',  ( -40.34137639590981905, 23.72187500034139873, -29.30972558990011478 ) ) ;
#8752=CARTESIAN_POINT ( 'NONE',  ( 9.631387414534489405E-15, 26.35937500034139802, 52.43083105670540789 ) ) ;
#8754=CARTESIAN_POINT ( 'NONE',  ( -40.34137639590981195, 34.12187500034139731, 29.30972558990012189 ) ) ;
#8755=EDGE_CURVE ( 'NONE', #14669, #4716, #3042, .T. ) ;
#8756=LINE ( 'NONE', #10096, #8152 ) ;
#8757=CARTESIAN_POINT ( 'NONE',  ( -30.90169943749474868, 35.69999999999999574, -42.53254041760200721 ) ) ;
#8758=CARTESIAN_POINT ( 'NONE',  ( 15.40903463028482356, 40.45937500034139589, 47.42413220539093999 ) ) ;
#8761=CARTESIAN_POINT ( 'NONE',  ( -40.45084971874737079, 44.20000000000000284, 29.38926261462367151 ) ) ;
#8770=CARTESIAN_POINT ( 'NONE',  ( 9.631387414534489405E-15, 40.42187500034138736, 52.43083105670540789 ) ) ;
#8773=CARTESIAN_POINT ( 'NONE',  ( -49.99999999999999289, 27.88125000068279746, 16.24598481164533226 ) ) ;
#8776=CARTESIAN_POINT ( 'NONE',  ( 49.86468353124999453, 37.02187500034138878, -16.20201782572376459 ) ) ;
#8778=EDGE_CURVE ( 'NONE', #11268, #11668, #6379, .T. ) ;
#8787=CARTESIAN_POINT ( 'NONE',  ( 30.81806926056964002, 30.55937500034139731, 42.41743335407647209 ) ) ;
#8789=CARTESIAN_POINT ( 'NONE',  ( -40.34137639590981905, 45.72187500034139873, -29.30972558990011478 ) ) ;
#8797=ORIENTED_EDGE ( 'NONE', *, *, #16383, .F. ) ;
#8811=CARTESIAN_POINT ( 'NONE',  ( -3.219174618344376363E-15, 47.28125000068278894, -52.57311121191334990 ) ) ;
#8812=CARTESIAN_POINT ( 'NONE',  ( 30.90169943749473802, 45.08125000068280031, -42.53254041760200721 ) ) ;
#8814=CARTESIAN_POINT ( 'NONE',  ( -15.40903463028481646, 21.45937500034139589, -47.42413220539093999 ) ) ;
#8818=CARTESIAN_POINT ( 'NONE',  ( 40.45084971874737789, 42.58125000068280031, 29.38926261462365375 ) ) ;
#8823=CARTESIAN_POINT ( 'NONE',  ( 2.600676159226420495E-13, 33.49999999999999289, -49.99999999999999289 ) ) ;
#8824=CARTESIAN_POINT ( 'NONE',  ( -10.22384026579626060, 36.71443566863956676, 92.96696093445143561 ) ) ;
#8828=CARTESIAN_POINT ( 'NONE',  ( -40.34137639590981195, 24.12187500034139731, 29.30972558990012189 ) ) ;
#8829=CARTESIAN_POINT ( 'NONE',  ( 15.40903463028482356, 20.45937500034139589, 47.42413220539093999 ) ) ;
#8831=CARTESIAN_POINT ( 'NONE',  ( 15.40903463028482356, 32.52187500034139589, 47.42413220539093999 ) ) ;
#8833=CARTESIAN_POINT ( 'NONE',  ( -40.45084971874737789, 33.80000000000000426, -29.38926261462365730 ) ) ;
#8834=CARTESIAN_POINT ( 'NONE',  ( 15.40903463028481113, 39.25937500034140015, -47.42413220539094709 ) ) ;
#8840=CARTESIAN_POINT ( 'NONE',  ( -15.45084971874736368, 48.40000000000000568, 47.55282581475768211 ) ) ;
#8844=ORIENTED_EDGE ( 'NONE', *, *, #787, .F. ) ;
#8845=LINE ( 'NONE', #1439, #13184 ) ;
#8848=MANIFOLD_SOLID_BREP ( 'Boss-Extrude2', #12910 ) ;
#8851=AXIS2_PLACEMENT_3D ( 'NONE', #9576, #3170, #15964 ) ;
#8854=CARTESIAN_POINT ( 'NONE',  ( -40.34137639590981905, 43.72187500034139873, -29.30972558990011478 ) ) ;
#8857=CARTESIAN_POINT ( 'NONE',  ( 50.00000000000000000, 30.78125000068279959, -6.123233995736766085E-15 ) ) ;
#8860=CARTESIAN_POINT ( 'NONE',  ( 30.81806926056962936, 35.22187500034138452, -42.41743335407647209 ) ) ;
#8863=B_SPLINE_CURVE_WITH_KNOTS ( 'NONE', 3,
 ( #4089, #16401, #5110, #8910, #12661, #13974, #15137, #10330, #12900, #9159, #3928, #8824, #14216, #2841, #7909, #1590, #253, #2502, #1510, #1257, #4010, #7747, #15388, #6602, #12986, #83, #1337, #3764 ),
 .UNSPECIFIED., .F., .F.,
 ( 4, 2, 2, 2, 2, 2, 2, 2, 2, 2, 2, 2, 2, 4 ),
 ( 0.06961014663733354479, 0.07132520376916648419, 0.07304026090099940971, 0.07475531803283234911, 0.07647037516466527463, 0.07990048942833113954, 0.08161554656016407894, 0.08333060369199700446, 0.08676071795566286937, 0.08847577508749582265, 0.09019083221932876204, 0.09362094648299464084, 0.09533600361482758023, 0.09705106074666051963 ),
 .UNSPECIFIED. ) ;
#8865=ORIENTED_EDGE ( 'NONE', *, *, #8420, .F. ) ;
#8869=CARTESIAN_POINT ( 'NONE',  ( -7.919222016226688865, 23.33250428222964246, -50.00000000000003553 ) ) ;
#8870=CARTESIAN_POINT ( 'NONE',  ( 49.86468353125001585, 30.75937500034139305, 16.20201782572375038 ) ) ;
#8874=CARTESIAN_POINT ( 'NONE',  ( -30.81806926056962226, 44.22187500034139163, 42.41743335407647209 ) ) ;
#8878=CARTESIAN_POINT ( 'NONE',  ( -7.919222016226773242, 42.44874571845315359, 50.00000000000000711 ) ) ;
#8883=VERTEX_POINT ( 'NONE', #2149 ) ;
#8893=CARTESIAN_POINT ( 'NONE',  ( 30.90169943749473802, 25.08125000068279675, -42.53254041760200721 ) ) ;
#8894=EDGE_CURVE ( 'NONE', #384, #10597, #10929, .T. ) ;
#8895=DIRECTION ( 'NONE',  ( 0.000000000000000000, 0.000000000000000000, -1.000000000000000000 ) ) ;
#8896=CARTESIAN_POINT ( 'NONE',  ( -3.219174618344376363E-15, 39.28125000068279604, -52.57311121191334990 ) ) ;
#8897=CARTESIAN_POINT ( 'NONE',  ( -5.823736356558307894E-14, 44.28125000068280315, 50.00000000000000000 ) ) ;
#8900=CARTESIAN_POINT ( 'NONE',  ( -40.45084971874737789, 25.80000000000000071, -29.38926261462365730 ) ) ;
#8907=AXIS2_PLACEMENT_3D ( 'NONE', #3054, #2814, #10637 ) ;
#8910=CARTESIAN_POINT ( 'NONE',  ( -2.303005534166477464, 39.85734974871404290, 92.94531063127084280 ) ) ;
#8914=CARTESIAN_POINT ( 'NONE',  ( 15.40903463028481113, 23.25937500034139660, -47.42413220539094709 ) ) ;
#8916=CARTESIAN_POINT ( 'NONE',  ( 9.631387414534489405E-15, 34.42187500034139447, 52.43083105670540789 ) ) ;
#8918=CARTESIAN_POINT ( 'NONE',  ( 9.657523855033129090E-15, 32.50000000000000000, 52.57311121191334990 ) ) ;
#8919=CARTESIAN_POINT ( 'NONE',  ( -3.210462471511496205E-15, 41.35937500034138736, -52.43083105670540789 ) ) ;
#8924=CARTESIAN_POINT ( 'NONE',  ( 40.45084971874737079, 47.20000000000000284, -29.38926261462366440 ) ) ;
#8927=EDGE_CURVE ( 'NONE', #11268, #13562, #13621, .T. ) ;
#8931=ORIENTED_EDGE ( 'NONE', *, *, #7914, .T. ) ;
#8936=FACE_OUTER_BOUND ( 'NONE', #7554, .T. ) ;
#8941=DIRECTION ( 'NONE',  ( -0.000000000000000000, 1.000000000000000000, -0.000000000000000000 ) ) ;
#8942=CARTESIAN_POINT ( 'NONE',  ( -40.34137639590981905, 41.72187500034139873, -29.30972558990011478 ) ) ;
#8945=CARTESIAN_POINT ( 'NONE',  ( 30.90169943749475578, 28.48125000068280244, 42.53254041760200010 ) ) ;
#8949=CARTESIAN_POINT ( 'NONE',  ( 40.34137639590981905, 32.72187500034139873, 29.30972558990010768 ) ) ;
#8960=CARTESIAN_POINT ( 'NONE',  ( 9.631387414534489405E-15, 32.35937500034139447, 52.43083105670540789 ) ) ;
#8962=CARTESIAN_POINT ( 'NONE',  ( -49.86468353124999453, 45.82187500034140015, -16.20201782572375393 ) ) ;
#8972=CARTESIAN_POINT ( 'NONE',  ( -15.45084971874737256, 45.38125000068279746, -47.55282581475767500 ) ) ;
#8974=ORIENTED_EDGE ( 'NONE', *, *, #8457, .F. ) ;
#8978=FACE_OUTER_BOUND ( 'NONE', #16243, .T. ) ;
#8980=CARTESIAN_POINT ( 'NONE',  ( -1.240322475938754499E-13, 38.50000000000000711, 50.00000000000000000 ) ) ;
#8983=DIRECTION ( 'NONE',  ( -0.000000000000000000, 1.000000000000000000, -0.000000000000000000 ) ) ;
#8984=CARTESIAN_POINT ( 'NONE',  ( 30.90169943749474157, 39.08125000068280031, -42.53254041760200721 ) ) ;
#8989=EDGE_LOOP ( 'NONE', ( #14132, #8351, #1953 ) ) ;
#8999=DIRECTION ( 'NONE',  ( 0.000000000000000000, 0.000000000000000000, 1.000000000000000000 ) ) ;
#9003=CARTESIAN_POINT ( 'NONE',  ( -49.86468353124999453, 25.75937500034139660, -16.20201782572375393 ) ) ;
#9006=CARTESIAN_POINT ( 'NONE',  ( -49.86468353124999453, 31.82187500034139305, -16.20201782572375393 ) ) ;
#9008=CARTESIAN_POINT ( 'NONE',  ( 40.45084971874737789, 30.80000000000000071, 29.38926261462365375 ) ) ;
#9010=CARTESIAN_POINT ( 'NONE',  ( 30.81806926056964002, 38.55937500034140442, 42.41743335407647209 ) ) ;
#9012=CARTESIAN_POINT ( 'NONE',  ( -40.45084971874737789, 41.80000000000000426, -29.38926261462365730 ) ) ;
#9020=AXIS2_PLACEMENT_3D ( 'NONE', #1299, #4904, #6222 ) ;
#9024=CARTESIAN_POINT ( 'NONE',  ( 49.86468353125001585, 40.82187500034140726, 16.20201782572375038 ) ) ;
#9025=CARTESIAN_POINT ( 'NONE',  ( 9.631387414534489405E-15, 42.35937500034140157, 52.43083105670540789 ) ) ;
#9028=CARTESIAN_POINT ( 'NONE',  ( -30.90169943749474868, 25.48125000068279888, -42.53254041760200721 ) ) ;
#9029=CARTESIAN_POINT ( 'NONE',  ( 17.06320572571393157, 26.42681735030989998, 93.80094291277063689 ) ) ;
#9031=CARTESIAN_POINT ( 'NONE',  ( -49.86468353124999453, 29.82187500034139660, -16.20201782572375393 ) ) ;
#9039=CARTESIAN_POINT ( 'NONE',  ( -7.919222016226688865, 23.55125428154684641, -50.00000000000003553 ) ) ;
#9041=CARTESIAN_POINT ( 'NONE',  ( 15.40903463028482356, 34.45937500034139589, 47.42413220539093999 ) ) ;
#9043=CARTESIAN_POINT ( 'NONE',  ( 40.34137639590981195, 45.12187500034139731, -29.30972558990011834 ) ) ;
#9055=CARTESIAN_POINT ( 'NONE',  ( 49.99999999999999289, 34.88125000068280457, -16.24598481164532160 ) ) ;
#9060=CARTESIAN_POINT ( 'NONE',  ( -50.00000000000000000, 22.00000000000000355, 0.000000000000000000 ) ) ;
#9061=CARTESIAN_POINT ( 'NONE',  ( -49.86468353124999453, 47.75937500034139305, -16.20201782572375393 ) ) ;
#9066=SURFACE_STYLE_FILL_AREA ( #13874 ) ;
#9068=CARTESIAN_POINT ( 'NONE',  ( -30.90169943749473802, 38.08125000068280031, 42.53254041760200721 ) ) ;
#9075=CARTESIAN_POINT ( 'NONE',  ( 30.90169943749475223, 42.48125000068279888, 42.53254041760199300 ) ) ;
#9078=VERTEX_POINT ( 'NONE', #1314 ) ;
#9079=DIRECTION ( 'NONE',  ( 0.000000000000000000, 0.000000000000000000, 1.000000000000000000 ) ) ;
#9083=CARTESIAN_POINT ( 'NONE',  ( 2.600676159226421000E-13, 21.50000000000000000, -49.99999999999999289 ) ) ;
#9084=CARTESIAN_POINT ( 'NONE',  ( 49.86468353125001585, 22.75937500034139660, 16.20201782572375038 ) ) ;
#9085=FACE_BOUND ( 'NONE', #14754, .T. ) ;
#9086=CARTESIAN_POINT ( 'NONE',  ( -30.81806926056963292, 27.62187500034139731, -42.41743335407646498 ) ) ;
#9088=CARTESIAN_POINT ( 'NONE',  ( -15.45084971874737256, 29.60000000000000142, -47.55282581475767500 ) ) ;
#9089=CARTESIAN_POINT ( 'NONE',  ( 15.40903463028482356, 34.45937500034139589, 47.42413220539093999 ) ) ;
#9101=CARTESIAN_POINT ( 'NONE',  ( 30.81806926056964002, 34.62187500034139731, 42.41743335407647209 ) ) ;
#9102=CARTESIAN_POINT ( 'NONE',  ( 40.34137639590981195, 41.05937500034139731, -29.30972558990011834 ) ) ;
#9106=CARTESIAN_POINT ( 'NONE',  ( 30.90169943749475578, 24.48125000068280244, 42.53254041760200010 ) ) ;
#9107=CARTESIAN_POINT ( 'NONE',  ( 7.778087436843963864, 38.21832046643818614, 92.94215756931615147 ) ) ;
#9108=CARTESIAN_POINT ( 'NONE',  ( -49.86468353124999453, 30.02187500034139234, 16.20201782572377525 ) ) ;
#9109=CARTESIAN_POINT ( 'NONE',  ( -40.45084971874737789, 27.80000000000000071, -29.38926261462365730 ) ) ;
#9116=CARTESIAN_POINT ( 'NONE',  ( 2.600676159226420495E-13, 23.50000000000000000, -49.99999999999999289 ) ) ;
#9118=CARTESIAN_POINT ( 'NONE',  ( 49.86468353125001585, 24.75937500034140015, 16.20201782572375038 ) ) ;
#9120=CARTESIAN_POINT ( 'NONE',  ( -15.40903463028480580, 48.32187500034140015, 47.42413220539094709 ) ) ;
#9124=CARTESIAN_POINT ( 'NONE',  ( 49.86468353124999453, 49.02187500034140299, -16.20201782572376459 ) ) ;
#9134=CARTESIAN_POINT ( 'NONE',  ( -30.90169943749473447, 44.08125000068279320, 42.53254041760200721 ) ) ;
#9137=CARTESIAN_POINT ( 'NONE',  ( 49.99999999999999289, 27.10000000000000497, -16.24598481164532160 ) ) ;
#9138=CARTESIAN_POINT ( 'NONE',  ( 49.86468353124999453, 48.95937500034140299, -16.20201782572376459 ) ) ;
#9139=CARTESIAN_POINT ( 'NONE',  ( -49.99999999999999289, 31.88125000068280102, 16.24598481164533226 ) ) ;
#9141=EDGE_CURVE ( 'NONE', #15007, #11588, #12629, .T. ) ;
#9142=CARTESIAN_POINT ( 'NONE',  ( 30.81806926056964002, 22.62187500034139731, 42.41743335407647209 ) ) ;
#9144=CARTESIAN_POINT ( 'NONE',  ( -40.45084971874737789, 37.58125000068280031, -29.38926261462365730 ) ) ;
#9146=CARTESIAN_POINT ( 'NONE',  ( -2.445080149700054274E-14, 46.28125000068280315, 50.00000000000000000 ) ) ;
#9148=EDGE_CURVE ( 'NONE', #13843, #2741, #551, .T. ) ;
#9155=CYLINDRICAL_SURFACE ( 'NONE', #16116, 50.00000000000000000 ) ;
#9157=VERTEX_POINT ( 'NONE', #388 ) ;
#9159=CARTESIAN_POINT ( 'NONE',  ( -7.790398555160043870, 38.21309231270640794, 92.94217575349884441 ) ) ;
#9164=CARTESIAN_POINT ( 'NONE',  ( -40.45084971874737789, 29.58125000068279675, -29.38926261462365730 ) ) ;
#9166=CARTESIAN_POINT ( 'NONE',  ( -47.79496856443377339, 20.00000000000000355, 14.21716018044757668 ) ) ;
#9167=CARTESIAN_POINT ( 'NONE',  ( -40.34137639590981195, 32.12187500034140442, 29.30972558990012189 ) ) ;
#9168=CARTESIAN_POINT ( 'NONE',  ( -15.45084971874736368, 22.39999999999999858, 47.55282581475768211 ) ) ;
#9169=CARTESIAN_POINT ( 'NONE',  ( -15.45084971874737256, 31.60000000000000142, -47.55282581475767500 ) ) ;
#9170=CARTESIAN_POINT ( 'NONE',  ( -3.210462471511496205E-15, 33.35937500034140157, -52.43083105670540789 ) ) ;
#9173=ORIENTED_EDGE ( 'NONE', *, *, #13712, .T. ) ;
#9175=EDGE_CURVE ( 'NONE', #14909, #15954, #7315, .T. ) ;
#9181=CARTESIAN_POINT ( 'NONE',  ( -7.919222016226752814, 37.55125428154683931, -50.00000000000000711 ) ) ;
#9184=CARTESIAN_POINT ( 'NONE',  ( -30.81806926056963292, 35.62187500034140442, -42.41743335407647209 ) ) ;
#9185=CARTESIAN_POINT ( 'NONE',  ( 30.81806926056962936, 43.15937500034139873, -42.41743335407646498 ) ) ;
#9191=CARTESIAN_POINT ( 'NONE',  ( -3.210462471511496205E-15, 49.35937500034138736, -52.43083105670540789 ) ) ;
#9192=CARTESIAN_POINT ( 'NONE',  ( 6.190300238984888459, 38.87860627667793523, 92.94022342448253937 ) ) ;
#9195=CARTESIAN_POINT ( 'NONE',  ( 9.631387414534489405E-15, 26.42187500034139447, 52.43083105670540789 ) ) ;
#9197=DIRECTION ( 'NONE',  ( 0.000000000000000000, 1.000000000000000000, 0.000000000000000000 ) ) ;
#9206=CARTESIAN_POINT ( 'NONE',  ( 50.00000000000000000, 30.78125000068279959, -6.123233995736766085E-15 ) ) ;
#9209=CARTESIAN_POINT ( 'NONE',  ( -49.86468353124999453, 21.95937500034138878, 16.20201782572377525 ) ) ;
#9211=CARTESIAN_POINT ( 'NONE',  ( -15.40903463028480580, 42.32187500034139305, 47.42413220539094709 ) ) ;
#9214=VECTOR ( 'NONE', #11800, 1000.000000000000227 ) ;
#9216=CARTESIAN_POINT ( 'NONE',  ( 49.86468353125001585, 46.82187500034139305, 16.20201782572375038 ) ) ;
#9222=EDGE_LOOP ( 'NONE', ( #4598, #6917, #7703, #13596 ) ) ;
#9225=CARTESIAN_POINT ( 'NONE',  ( -7.919222016226838967, 44.22999571913595673, 49.99999999999999289 ) ) ;
#9229=CARTESIAN_POINT ( 'NONE',  ( -49.99999999999999289, 24.10000000000000142, 16.24598481164533226 ) ) ;
#9230=CARTESIAN_POINT ( 'NONE',  ( -49.86468353125000164, 41.85937500034139447, 0.000000000000000000 ) ) ;
#9231=CARTESIAN_POINT ( 'NONE',  ( 2.600676159226420495E-13, 31.28125000068279604, -49.99999999999999289 ) ) ;
#9234=AXIS2_PLACEMENT_3D ( 'NONE', #13653, #7112, #2261 ) ;
#9236=CARTESIAN_POINT ( 'NONE',  ( -49.99999999999999289, 41.88125000068279746, 16.24598481164533226 ) ) ;
#9238=CARTESIAN_POINT ( 'NONE',  ( 30.90169943749475223, 22.48125000068279533, 42.53254041760199300 ) ) ;
#9241=( BOUNDED_CURVE ( )  B_SPLINE_CURVE ( 2, ( #5310, #10360, #607, #15593, #6797, #13335, #7944, #13096, #452, #4214, #11847, #1701, #5553 ),
 .UNSPECIFIED., .F., .F. ) 
 B_SPLINE_CURVE_WITH_KNOTS ( ( 3, 2, 2, 2, 2, 2, 3 ),
 ( 0.7166666666666666741, 0.7199999999999999734, 0.7266666666666666829, 0.7333333333333332815, 0.7399999999999999911, 0.7466666666666667007, 0.7500000000000000000 ),
 .UNSPECIFIED. ) 
 CURVE ( )  GEOMETRIC_REPRESENTATION_ITEM ( )  RATIONAL_B_SPLINE_CURVE ( ( 0.9755282581475768211, 0.9755282581475768211, 1.000000000000000000, 0.9510565162951535312, 1.000000000000000000, 0.9510565162951535312, 1.000000000000000000, 0.9510565162951535312, 1.000000000000000000, 0.9510565162951535312, 1.000000000000000000, 0.9755282581475768211, 0.9755282581475768211 ) ) 
 REPRESENTATION_ITEM ( '' )  );
#9243=EDGE_LOOP ( 'NONE', ( #4575, #13546, #5272, #10443 ) ) ;
#9245=CARTESIAN_POINT ( 'NONE',  ( 0.000000000000000000, 20.00000000000000355, 0.000000000000000000 ) ) ;
#9246=CARTESIAN_POINT ( 'NONE',  ( 0.000000000000000000, 20.00000000000000355, 50.00000000000000000 ) ) ;
#9251=CYLINDRICAL_SURFACE ( 'NONE', #5414, 50.00000000000000000 ) ;
#9254=CARTESIAN_POINT ( 'NONE',  ( 15.72133679436987386, 14.79214933101786222, 96.11488922061346329 ) ) ;
#9255=CARTESIAN_POINT ( 'NONE',  ( -46.50201513659311559, 20.00000000000000355, 18.00136805656113026 ) ) ;
#9256=CARTESIAN_POINT ( 'NONE',  ( -30.81806926056962226, 28.22187500034139873, 42.41743335407647209 ) ) ;
#9257=CARTESIAN_POINT ( 'NONE',  ( 1.293669679204937499E-13, 41.50000000000000000, -50.00000000000000000 ) ) ;
#9259=CARTESIAN_POINT ( 'NONE',  ( -15.40903463028480580, 32.25937500034140015, 47.42413220539094709 ) ) ;
#9264=VERTEX_POINT ( 'NONE', #15614 ) ;
#9267=CARTESIAN_POINT ( 'NONE',  ( -15.45084971874737256, 37.60000000000000142, -47.55282581475767500 ) ) ;
#9273=CARTESIAN_POINT ( 'NONE',  ( -30.81806926056962226, 34.22187500034139873, 42.41743335407647919 ) ) ;
#9274=CARTESIAN_POINT ( 'NONE',  ( -49.86468353124999453, 33.75937500034140015, -16.20201782572375393 ) ) ;
#9278=CARTESIAN_POINT ( 'NONE',  ( 9.631387414534489405E-15, 48.35937500034140157, 52.43083105670540789 ) ) ;
#9280=CARTESIAN_POINT ( 'NONE',  ( -15.40903463028481646, 29.52187500034139589, -47.42413220539093999 ) ) ;
#9290=CARTESIAN_POINT ( 'NONE',  ( -49.86468353125000164, 25.85937500034139802, 0.000000000000000000 ) ) ;
#9293=CARTESIAN_POINT ( 'NONE',  ( 15.40903463028481113, 39.32187500034140015, -47.42413220539094709 ) ) ;
#9297=ADVANCED_FACE ( 'NONE', ( #1724 ), #4396, .F. ) ;
#9298=CARTESIAN_POINT ( 'NONE',  ( -40.34137639590981905, 45.72187500034139873, -29.30972558990011478 ) ) ;
#9300=ORIENTED_EDGE ( 'NONE', *, *, #5033, .T. ) ;
#9302=ORIENTED_EDGE ( 'NONE', *, *, #1781, .F. ) ;
#9305=CARTESIAN_POINT ( 'NONE',  ( -15.45084971874736368, 44.18125000068280173, 47.55282581475768211 ) ) ;
#9308=CARTESIAN_POINT ( 'NONE',  ( 30.90169943749474157, 25.30000000000000071, -42.53254041760200721 ) ) ;
#9309=CARTESIAN_POINT ( 'NONE',  ( 30.81806926056964002, 44.55937500034139020, 42.41743335407647209 ) ) ;
#9311=DIRECTION ( 'NONE',  ( 0.000000000000000000, 1.000000000000000000, 0.000000000000000000 ) ) ;
#9314=CARTESIAN_POINT ( 'NONE',  ( 40.45084971874737079, 30.98125000068279888, -29.38926261462366440 ) ) ;
#9317=CARTESIAN_POINT ( 'NONE',  ( 49.99999999999999289, 20.88125000068279746, -16.24598481164532160 ) ) ;
#9320=ORIENTED_EDGE ( 'NONE', *, *, #1205, .T. ) ;
#9325=DIRECTION ( 'NONE',  ( 0.000000000000000000, 0.000000000000000000, 1.000000000000000000 ) ) ;
#9328=DIRECTION ( 'NONE',  ( -0.000000000000000000, 1.000000000000000000, -0.000000000000000000 ) ) ;
#9332=CARTESIAN_POINT ( 'NONE',  ( 1.293669679204937499E-13, 37.28125000068280315, -50.00000000000000000 ) ) ;
#9333=CARTESIAN_POINT ( 'NONE',  ( 14.27695618825629431, 12.36406312199577506, 96.77295768394273523 ) ) ;
#9335=CARTESIAN_POINT ( 'NONE',  ( 15.40903463028482356, 26.52187500034139589, 47.42413220539093999 ) ) ;
#9339=CARTESIAN_POINT ( 'NONE',  ( 15.40903463028481113, 31.25937500034140015, -47.42413220539094709 ) ) ;
#9344=CARTESIAN_POINT ( 'NONE',  ( -2.547328955960238000E-13, 22.28125000068279604, 49.99999999999999289 ) ) ;
#9349=CARTESIAN_POINT ( 'NONE',  ( 40.34137639590981195, 37.12187500034139731, -29.30972558990011834 ) ) ;
#9350=CARTESIAN_POINT ( 'NONE',  ( -30.81806926056963292, 33.55937500034139020, -42.41743335407646498 ) ) ;
#9353=CARTESIAN_POINT ( 'NONE',  ( -50.00000000000000000, 23.78125000068279959, 0.000000000000000000 ) ) ;
#9355=CARTESIAN_POINT ( 'NONE',  ( -15.40903463028481646, 25.52187500034139589, -47.42413220539093999 ) ) ;
#9365=AXIS2_PLACEMENT_3D ( 'NONE', #14102, #12954, #132 ) ;
#9366=CARTESIAN_POINT ( 'NONE',  ( -15.45084971874736368, 34.18125000068279462, 47.55282581475768211 ) ) ;
#9368=CARTESIAN_POINT ( 'NONE',  ( -30.81806926056962226, 24.15937500034139873, 42.41743335407647919 ) ) ;
#9371=CARTESIAN_POINT ( 'NONE',  ( 40.34137639590981195, 41.12187500034139731, -29.30972558990011834 ) ) ;
#9373=CARTESIAN_POINT ( 'NONE',  ( -40.34137639590981195, 46.12187500034139731, 29.30972558990012189 ) ) ;
#9381=DIRECTION ( 'NONE',  ( 1.000000000000000000, 0.000000000000000000, 0.000000000000000000 ) ) ;
#9384=CARTESIAN_POINT ( 'NONE',  ( 15.45084971874737789, 24.60000000000000142, 47.55282581475767500 ) ) ;
#9385=CARTESIAN_POINT ( 'NONE',  ( -30.81806926056963292, 45.55937500034139731, -42.41743335407647209 ) ) ;
#9386=CARTESIAN_POINT ( 'NONE',  ( -7.919222016226688865, 31.33250428222963890, -50.00000000000003553 ) ) ;
#9390=CARTESIAN_POINT ( 'NONE',  ( 0.000000000000000000, 20.00000000000000355, 50.00000000000000000 ) ) ;
#9393=CARTESIAN_POINT ( 'NONE',  ( 50.00000000000000711, 34.68125000068279462, 16.24598481164530739 ) ) ;
#9406=CARTESIAN_POINT ( 'NONE',  ( 0.000000000000000000, 20.00000000000000355, 0.000000000000000000 ) ) ;
#9407=CARTESIAN_POINT ( 'NONE',  ( 30.90169943749475223, 22.69999999999999929, 42.53254041760199300 ) ) ;
#9411=CARTESIAN_POINT ( 'NONE',  ( 30.90169943749473802, 47.29999999999999716, -42.53254041760200721 ) ) ;
#9412=CARTESIAN_POINT ( 'NONE',  ( -48.32661496269150803, 20.00000000000000355, 12.28922088333830054 ) ) ;
#9413=CARTESIAN_POINT ( 'NONE',  ( -30.81806926056962226, 24.22187500034139518, 42.41743335407647209 ) ) ;
#9417=CARTESIAN_POINT ( 'NONE',  ( 15.40903463028482356, 24.45937500034139589, 47.42413220539093999 ) ) ;
#9428=CARTESIAN_POINT ( 'NONE',  ( 30.81806926056962936, 35.22187500034138452, -42.41743335407647209 ) ) ;
#9429=CARTESIAN_POINT ( 'NONE',  ( -49.86468353125000164, 35.85937500034140157, 0.000000000000000000 ) ) ;
#9430=CARTESIAN_POINT ( 'NONE',  ( -30.90169943749474513, 43.70000000000000284, -42.53254041760200721 ) ) ;
#9433=CARTESIAN_POINT ( 'NONE',  ( -30.90169943749474868, 21.48125000068279533, -42.53254041760200721 ) ) ;
#9437=CARTESIAN_POINT ( 'NONE',  ( 40.34137639590981195, 23.12187500034139731, -29.30972558990011834 ) ) ;
#9442=ORIENTED_EDGE ( 'NONE', *, *, #14467, .T. ) ;
#9446=CARTESIAN_POINT ( 'NONE',  ( -30.81806926056963292, 23.55937500034139376, -42.41743335407647209 ) ) ;
#9451=CARTESIAN_POINT ( 'NONE',  ( -50.00000000000000000, 40.00000000000000000, 0.000000000000000000 ) ) ;
#9452=CARTESIAN_POINT ( 'NONE',  ( 15.40903463028482356, 46.52187500034139589, 47.42413220539093999 ) ) ;
#9457=AXIS2_PLACEMENT_3D ( 'NONE', #9703, #11032, #796 ) ;
#9468=CARTESIAN_POINT ( 'NONE',  ( 49.86468353124999453, 46.95937500034139589, -16.20201782572376459 ) ) ;
#9471=CARTESIAN_POINT ( 'NONE',  ( -15.40903463028481646, 47.45937500034139589, -47.42413220539093999 ) ) ;
#9477=SHAPE_REPRESENTATION ( 'container base & motor', ( #15812 ), #1480 ) ;
#9480=CARTESIAN_POINT ( 'NONE',  ( 7.919222016226940219, 21.22999571913595673, -49.99999999999996447 ) ) ;
#9496=FACE_OUTER_BOUND ( 'NONE', #2994, .T. ) ;
#9499=CARTESIAN_POINT ( 'NONE',  ( 17.27465264870989259, 19.64379522392349031, 94.97817908659912689 ) ) ;
#9500=CARTESIAN_POINT ( 'NONE',  ( -47.93512317712408333, 19.99999999999999645, 13.73719875613861241 ) ) ;
#9502=CARTESIAN_POINT ( 'NONE',  ( 40.34137639590981195, 23.12187500034139731, -29.30972558990011834 ) ) ;
#9506=CARTESIAN_POINT ( 'NONE',  ( -40.34137639590981195, 24.05937500034139731, 29.30972558990012189 ) ) ;
#9517=CARTESIAN_POINT ( 'NONE',  ( 15.40903463028481113, 27.32187500034139660, -47.42413220539094709 ) ) ;
#9518=CARTESIAN_POINT ( 'NONE',  ( 9.631387414534489405E-15, 38.35937500034139447, 52.43083105670540789 ) ) ;
#9519=CARTESIAN_POINT ( 'NONE',  ( -40.45084971874737079, 44.20000000000000284, 29.38926261462367151 ) ) ;
#9522=CARTESIAN_POINT ( 'NONE',  ( -30.81806926056963292, 45.55937500034139731, -42.41743335407647209 ) ) ;
#9525=CARTESIAN_POINT ( 'NONE',  ( -49.86468353124999453, 21.82187500034139305, -16.20201782572375393 ) ) ;
#9533=CARTESIAN_POINT ( 'NONE',  ( 6.123233995736766085E-15, 20.00000000000000355, -50.00000000000000000 ) ) ;
#9536=CARTESIAN_POINT ( 'NONE',  ( 49.86468353124999453, 47.02187500034139589, -16.20201782572376459 ) ) ;
#9538=CARTESIAN_POINT ( 'NONE',  ( -49.99999999999999289, 37.90000000000000568, -16.24598481164531449 ) ) ;
#9540=CARTESIAN_POINT ( 'NONE',  ( -49.86468353124999453, 39.82187500034140015, -16.20201782572375393 ) ) ;
#9548=LINE ( 'NONE', #3219, #13156 ) ;
#9552=CARTESIAN_POINT ( 'NONE',  ( 9.631387414534489405E-15, 44.35937500034140157, 52.43083105670540789 ) ) ;
#9553=CARTESIAN_POINT ( 'NONE',  ( 30.81806926056964002, 46.55937500034139020, 42.41743335407646498 ) ) ;
#9558=CARTESIAN_POINT ( 'NONE',  ( 0.000000000000000000, 20.00000000000000355, 0.000000000000000000 ) ) ;
#9559=EDGE_CURVE ( 'NONE', #8721, #14669, #9548, .T. ) ;
#9561=DIRECTION ( 'NONE',  ( 0.000000000000000000, 1.000000000000000000, 0.000000000000000000 ) ) ;
#9564=ORIENTED_EDGE ( 'NONE', *, *, #6034, .F. ) ;
#9576=CARTESIAN_POINT ( 'NONE',  ( 0.000000000000000000, 20.00000000000000355, 0.000000000000000000 ) ) ;
#9581=CARTESIAN_POINT ( 'NONE',  ( 49.86468353125001585, 20.82187500034140015, 16.20201782572375038 ) ) ;
#9585=CARTESIAN_POINT ( 'NONE',  ( 15.40903463028481113, 23.25937500034139660, -47.42413220539094709 ) ) ;
#9586=CARTESIAN_POINT ( 'NONE',  ( -3.111920190527341144E-15, 29.50000000000000000, -50.00000000000000000 ) ) ;
#9587=ORIENTED_EDGE ( 'NONE', *, *, #15336, .F. ) ;
#9592=CARTESIAN_POINT ( 'NONE',  ( 15.45084971874737789, 28.38125000068279746, 47.55282581475767500 ) ) ;
#9594=CARTESIAN_POINT ( 'NONE',  ( 9.631387414534489405E-15, 26.42187500034139447, 52.43083105670540789 ) ) ;
#9595=CARTESIAN_POINT ( 'NONE',  ( 40.34137639590981195, 33.05937500034139731, -29.30972558990011834 ) ) ;
#9598=FACE_OUTER_BOUND ( 'NONE', #15252, .T. ) ;
#9599=CARTESIAN_POINT ( 'NONE',  ( -30.81806926056962226, 42.15937500034139163, 42.41743335407647919 ) ) ;
#9601=CARTESIAN_POINT ( 'NONE',  ( -3.210462471511496205E-15, 21.42187500034139802, -52.43083105670540789 ) ) ;
#9604=ORIENTED_EDGE ( 'NONE', *, *, #11870, .T. ) ;
#9608=CYLINDRICAL_SURFACE ( 'NONE', #15006, 50.00000000000000000 ) ;
#9611=CARTESIAN_POINT ( 'NONE',  ( -49.86468353124999453, 49.82187500034140015, -16.20201782572375393 ) ) ;
#9614=CARTESIAN_POINT ( 'NONE',  ( -49.99999999999999289, 40.09999999999999432, 16.24598481164533226 ) ) ;
#9615=CARTESIAN_POINT ( 'NONE',  ( -30.81806926056963292, 41.62187500034139020, -42.41743335407647209 ) ) ;
#9624=CARTESIAN_POINT ( 'NONE',  ( -50.00000000000000000, 49.78125000068280315, 0.000000000000000000 ) ) ;
#9626=CARTESIAN_POINT ( 'NONE',  ( -49.86468353124999453, 35.95937500034139589, 16.20201782572377525 ) ) ;
#9627=CARTESIAN_POINT ( 'NONE',  ( -49.86468353125000164, 45.85937500034140157, 0.000000000000000000 ) ) ;
#9631=CARTESIAN_POINT ( 'NONE',  ( 0.000000000000000000, 50.00000000000000000, 0.000000000000000000 ) ) ;
#9632=CARTESIAN_POINT ( 'NONE',  ( 50.00000000000000711, 36.89999999999999858, 16.24598481164530739 ) ) ;
#9634=VERTEX_POINT ( 'NONE', #13683 ) ;
#9639=VERTEX_POINT ( 'NONE', #12529 ) ;
#9642=CARTESIAN_POINT ( 'NONE',  ( -30.90169943749474513, 39.69999999999999574, -42.53254041760200721 ) ) ;
#9645=CARTESIAN_POINT ( 'NONE',  ( -15.45084971874736368, 38.40000000000000568, 47.55282581475768211 ) ) ;
#9646=LINE ( 'NONE', #8481, #11165 ) ;
#9655=CARTESIAN_POINT ( 'NONE',  ( 49.86468353124999453, 25.02187500034139589, -16.20201782572376104 ) ) ;
#9658=CARTESIAN_POINT ( 'NONE',  ( -49.86468353124999453, 25.75937500034140015, -16.20201782572375393 ) ) ;
#9659=AXIS2_PLACEMENT_3D ( 'NONE', #6771, #5526, #11981 ) ;
#9666=( BOUNDED_CURVE ( )  B_SPLINE_CURVE ( 2, ( #6530, #16248, #4882, #27, #6200, #16330, #2442, #1187, #6285, #10107, #11356, #16421, #15159 ),
 .UNSPECIFIED., .F., .F. ) 
 B_SPLINE_CURVE_WITH_KNOTS ( ( 3, 2, 2, 2, 2, 2, 3 ),
 ( 0.5166666666666667185, 0.5200000000000000178, 0.5266666666666666163, 0.5333333333333333259, 0.5400000000000000355, 0.5466666666666666341, 0.5500000000000000444 ),
 .UNSPECIFIED. ) 
 CURVE ( )  GEOMETRIC_REPRESENTATION_ITEM ( )  RATIONAL_B_SPLINE_CURVE ( ( 0.9755282581475768211, 0.9755282581475771542, 1.000000000000000000, 0.9510565162951535312, 1.000000000000000000, 0.9510565162951535312, 1.000000000000000000, 0.9510565162951535312, 1.000000000000000000, 0.9510565162951535312, 1.000000000000000000, 0.9755282581475763770, 0.9755282581475768211 ) ) 
 REPRESENTATION_ITEM ( '' )  );
#9670=VECTOR ( 'NONE', #9721, 1000.000000000000000 ) ;
#9672=CARTESIAN_POINT ( 'NONE',  ( -49.86468353124999453, 30.02187500034139234, 16.20201782572377525 ) ) ;
#9673=CARTESIAN_POINT ( 'NONE',  ( 49.86468353124999453, 30.95937500034139944, -16.20201782572376104 ) ) ;
#9674=CARTESIAN_POINT ( 'NONE',  ( 0.000000000000000000, 20.00000000000000355, 50.00000000000000000 ) ) ;
#9678=CARTESIAN_POINT ( 'NONE',  ( 9.631387414534489405E-15, 44.35937500034140157, 52.43083105670540789 ) ) ;
#9681=CARTESIAN_POINT ( 'NONE',  ( -49.86468353124999453, 20.02187500034139589, 16.20201782572377525 ) ) ;
#9687=ORIENTED_EDGE ( 'NONE', *, *, #1165, .T. ) ;
#9690=CARTESIAN_POINT ( 'NONE',  ( 30.81806926056962936, 49.22187500034139873, -42.41743335407647209 ) ) ;
#9692=DIRECTION ( 'NONE',  ( -0.000000000000000000, 1.000000000000000000, -0.000000000000000000 ) ) ;
#9693=AXIS2_PLACEMENT_3D ( 'NONE', #9245, #15632, #10577 ) ;
#9696=CARTESIAN_POINT ( 'NONE',  ( -15.45084971874737256, 33.38125000068280457, -47.55282581475767500 ) ) ;
#9697=CARTESIAN_POINT ( 'NONE',  ( -30.90169943749473802, 38.29999999999999716, 42.53254041760200721 ) ) ;
#9699=CARTESIAN_POINT ( 'NONE',  ( 30.81806926056962936, 43.22187500034140584, -42.41743335407647209 ) ) ;
#9703=CARTESIAN_POINT ( 'NONE',  ( 8.660254037844387298, 28.00000000000000355, 5.000000000000000000 ) ) ;
#9709=COLOUR_RGB ( '', 0.08235294, 0.09019608, 0.10196078) ;
#9712=CARTESIAN_POINT ( 'NONE',  ( -40.45084971874737079, 21.98125000068279888, 29.38926261462367151 ) ) ;
#9714=CARTESIAN_POINT ( 'NONE',  ( -49.86468353124999453, 37.95937500034140299, 16.20201782572377525 ) ) ;
#9715=CARTESIAN_POINT ( 'NONE',  ( 40.34137639590981195, 49.05937500034139731, -29.30972558990011834 ) ) ;
#9721=DIRECTION ( 'NONE',  ( -0.000000000000000000, 1.000000000000000000, -0.000000000000000000 ) ) ;
#9726=CARTESIAN_POINT ( 'NONE',  ( 40.45084971874737789, 44.58125000068280031, 29.38926261462365375 ) ) ;
#9733=VECTOR ( 'NONE', #4873, 1000.000000000000000 ) ;
#9742=CYLINDRICAL_SURFACE ( 'NONE', #15021, 50.00000000000000000 ) ;
#9743=CARTESIAN_POINT ( 'NONE',  ( 0.000000000000000000, 20.00000000000000355, 0.000000000000000000 ) ) ;
#9746=CARTESIAN_POINT ( 'NONE',  ( -50.00000000000000000, 32.00000000000000000, 0.000000000000000000 ) ) ;
#9749=CARTESIAN_POINT ( 'NONE',  ( -49.86468353124999453, 23.82187500034139305, -16.20201782572375393 ) ) ;
#9752=CARTESIAN_POINT ( 'NONE',  ( 30.81806926056964002, 28.55937500034139731, 42.41743335407647209 ) ) ;
#9757=CARTESIAN_POINT ( 'NONE',  ( 50.00000000000000000, 45.00000000000000711, -6.123233995736766085E-15 ) ) ;
#9759=CARTESIAN_POINT ( 'NONE',  ( 49.99999999999999289, 49.10000000000000142, -16.24598481164532160 ) ) ;
#9765=CARTESIAN_POINT ( 'NONE',  ( 40.34137639590981905, 32.72187500034139873, 29.30972558990010768 ) ) ;
#9766=CARTESIAN_POINT ( 'NONE',  ( 49.86468353125001585, 28.75937500034139305, 16.20201782572375038 ) ) ;
#9767=CARTESIAN_POINT ( 'NONE',  ( 7.919222016226809657, 27.22999571913595318, -50.00000000000000000 ) ) ;
#9770=CARTESIAN_POINT ( 'NONE',  ( -49.86468353124999453, 47.75937500034139305, -16.20201782572375393 ) ) ;
#9773=CARTESIAN_POINT ( 'NONE',  ( -15.40903463028480580, 20.32187500034139660, 47.42413220539094709 ) ) ;
#9785=CARTESIAN_POINT ( 'NONE',  ( -49.86468353124999453, 21.75937500034140015, -16.20201782572375393 ) ) ;
#9788=CARTESIAN_POINT ( 'NONE',  ( 49.99999999999999289, 32.88125000068280457, -16.24598481164532160 ) ) ;
#9789=CARTESIAN_POINT ( 'NONE',  ( -15.40903463028481646, 37.52187500034139589, -47.42413220539093999 ) ) ;
#9791=VERTEX_POINT ( 'NONE', #10621 ) ;
#9799=CARTESIAN_POINT ( 'NONE',  ( 0.000000000000000000, 20.00000000000000355, 0.000000000000000000 ) ) ;
#9801=CARTESIAN_POINT ( 'NONE',  ( 49.86468353125001585, 40.75937500034138594, 16.20201782572375038 ) ) ;
#9811=CARTESIAN_POINT ( 'NONE',  ( -3.111920190527341144E-15, 25.28125000068279604, -50.00000000000000000 ) ) ;
#9816=CARTESIAN_POINT ( 'NONE',  ( 0.000000000000000000, 20.00000000000000355, 0.000000000000000000 ) ) ;
#9817=CARTESIAN_POINT ( 'NONE',  ( 7.919222016226809657, 29.44874571845315359, -50.00000000000000000 ) ) ;
#9821=CARTESIAN_POINT ( 'NONE',  ( -12.83488150441995401, 10.59022649794657234, 97.29057659180030271 ) ) ;
#9822=DIRECTION ( 'NONE',  ( 0.000000000000000000, 0.000000000000000000, 1.000000000000000000 ) ) ;
#9828=CARTESIAN_POINT ( 'NONE',  ( -45.93954244148126520, 20.00000000000000355, 19.39188242381481331 ) ) ;
#9829=CARTESIAN_POINT ( 'NONE',  ( 9.657523855033129090E-15, 44.28125000068280315, 52.57311121191334990 ) ) ;
#9833=CARTESIAN_POINT ( 'NONE',  ( -15.40903463028480580, 22.25937500034139660, 47.42413220539094709 ) ) ;
#9837=CARTESIAN_POINT ( 'NONE',  ( 7.919222016226809657, 45.44874571845314648, -50.00000000000000000 ) ) ;
#9842=FACE_OUTER_BOUND ( 'NONE', #8634, .T. ) ;
#9843=CARTESIAN_POINT ( 'NONE',  ( 49.99999999999999289, 28.88125000068279391, -16.24598481164532160 ) ) ;
#9845=CARTESIAN_POINT ( 'NONE',  ( -3.210462471511496205E-15, 27.42187500034139092, -52.43083105670540789 ) ) ;
#9846=CARTESIAN_POINT ( 'NONE',  ( -49.86468353124999453, 29.95937500034139589, 16.20201782572377169 ) ) ;
#9847=CARTESIAN_POINT ( 'NONE',  ( 30.90169943749475223, 26.48125000068279888, 42.53254041760199300 ) ) ;
#9848=CARTESIAN_POINT ( 'NONE',  ( -49.86468353124999453, 35.82187500034139305, -16.20201782572375393 ) ) ;
#9850=CARTESIAN_POINT ( 'NONE',  ( -49.86468353125000164, 43.85937500034140157, 0.000000000000000000 ) ) ;
#9852=CARTESIAN_POINT ( 'NONE',  ( 30.90169943749474157, 47.29999999999999716, -42.53254041760200721 ) ) ;
#9853=ORIENTED_EDGE ( 'NONE', *, *, #8457, .T. ) ;
#9859=CARTESIAN_POINT ( 'NONE',  ( 15.40903463028482356, 48.52187500034140299, 47.42413220539093999 ) ) ;
#9862=CARTESIAN_POINT ( 'NONE',  ( -3.219174618344376363E-15, 31.28125000068279604, -52.57311121191334990 ) ) ;
#9865=CARTESIAN_POINT ( 'NONE',  ( 40.34137639590981195, 39.12187500034139731, -29.30972558990011834 ) ) ;
#9873=ORIENTED_EDGE ( 'NONE', *, *, #3544, .F. ) ;
#9877=CARTESIAN_POINT ( 'NONE',  ( 8.446640517145639571E-15, 26.50000000000000000, 50.00000000000000000 ) ) ;
#9878=FACE_OUTER_BOUND ( 'NONE', #1437, .T. ) ;
#9879=CARTESIAN_POINT ( 'NONE',  ( -49.86468353124999453, 39.95937500034139589, 16.20201782572377525 ) ) ;
#9880=CARTESIAN_POINT ( 'NONE',  ( -15.40903463028480580, 42.25937500034139305, 47.42413220539094709 ) ) ;
#9882=CARTESIAN_POINT ( 'NONE',  ( -15.40903463028481646, 49.52187500034140299, -47.42413220539093999 ) ) ;
#9884=CARTESIAN_POINT ( 'NONE',  ( -49.95625437244530787, 20.00000000000000355, 4.103175251694850090 ) ) ;
#9886=CARTESIAN_POINT ( 'NONE',  ( 7.513064459987437071E-14, 42.50000000000000000, 50.00000000000000000 ) ) ;
#9895=( NAMED_UNIT ( * ) PLANE_ANGLE_UNIT ( ) SI_UNIT ( $, .RADIAN. ) );
#9900=CARTESIAN_POINT ( 'NONE',  ( -15.96758378294258662, 15.31621546249057708, 95.98047841688359938 ) ) ;
#9905=LINE ( 'NONE', #1553, #13194 ) ;
#9908=CARTESIAN_POINT ( 'NONE',  ( -49.99999999999999289, 45.68125000068280173, -16.24598481164531449 ) ) ;
#9909=CARTESIAN_POINT ( 'NONE',  ( 7.919222016226693306, 20.55125428154684641, 50.00000000000003553 ) ) ;
#9911=CARTESIAN_POINT ( 'NONE',  ( -40.45084971874737079, 26.20000000000000284, 29.38926261462367151 ) ) ;
#9917=CARTESIAN_POINT ( 'NONE',  ( 15.45084971874737789, 44.60000000000000142, 47.55282581475767500 ) ) ;
#9923=CARTESIAN_POINT ( 'NONE',  ( 7.919222016226693306, 34.55125428154684641, 50.00000000000003553 ) ) ;
#9925=CARTESIAN_POINT ( 'NONE',  ( -49.86468353124999453, 26.02187500034139944, 16.20201782572377525 ) ) ;
#9926=CARTESIAN_POINT ( 'NONE',  ( 49.86468353125001585, 32.75937500034140015, 16.20201782572375038 ) ) ;
#9928=CARTESIAN_POINT ( 'NONE',  ( 49.86468353124999453, 33.02187500034139589, -16.20201782572376104 ) ) ;
#9931=CARTESIAN_POINT ( 'NONE',  ( 40.34137639590981195, 37.05937500034139731, -29.30972558990011834 ) ) ;
#9933=CARTESIAN_POINT ( 'NONE',  ( -49.99999999999999289, 48.10000000000000142, 16.24598481164533226 ) ) ;
#9941=CARTESIAN_POINT ( 'NONE',  ( -30.81806926056963292, 41.62187500034139020, -42.41743335407647209 ) ) ;
#9942=DIRECTION ( 'NONE',  ( -0.000000000000000000, 1.000000000000000000, -0.000000000000000000 ) ) ;
#9944=CARTESIAN_POINT ( 'NONE',  ( 15.45084971874736723, 29.18125000068279817, -47.55282581475768211 ) ) ;
#9946=CARTESIAN_POINT ( 'NONE',  ( 49.86468353125001585, 32.82187500034139305, 16.20201782572375038 ) ) ;
#9952=ORIENTED_EDGE ( 'NONE', *, *, #4314, .T. ) ;
#9957=DIRECTION ( 'NONE',  ( 0.000000000000000000, -0.000000000000000000, 1.000000000000000000 ) ) ;
#9958=CARTESIAN_POINT ( 'NONE',  ( -30.90169943749473447, 24.08125000068279675, 42.53254041760200721 ) ) ;
#9959=CARTESIAN_POINT ( 'NONE',  ( 40.34137639590981905, 30.65937500034139518, 29.30972558990010768 ) ) ;
#9960=CARTESIAN_POINT ( 'NONE',  ( 30.81806926056964002, 40.55937500034139731, 42.41743335407646498 ) ) ;
#9963=LINE ( 'NONE', #13693, #373 ) ;
#9972=ORIENTED_EDGE ( 'NONE', *, *, #1682, .F. ) ;
#9978=VERTEX_POINT ( 'NONE', #612 ) ;
#9980=CYLINDRICAL_SURFACE ( 'NONE', #12202, 50.00000000000000000 ) ;
#9981=DIRECTION ( 'NONE',  ( 0.000000000000000000, 0.000000000000000000, 1.000000000000000000 ) ) ;
#9990=CARTESIAN_POINT ( 'NONE',  ( -50.00000000000000000, 45.78125000068279604, 0.000000000000000000 ) ) ;
#9992=CARTESIAN_POINT ( 'NONE',  ( 9.631387414534489405E-15, 22.35937500034139802, 52.43083105670540789 ) ) ;
#10000=CARTESIAN_POINT ( 'NONE',  ( 15.45084971874736723, 43.18125000068280173, -47.55282581475768211 ) ) ;
#10001=VERTEX_POINT ( 'NONE', #12419 ) ;
#10010=CARTESIAN_POINT ( 'NONE',  ( -30.81806926056963292, 25.62187500034139731, -42.41743335407647209 ) ) ;
#10011=CARTESIAN_POINT ( 'NONE',  ( 40.34137639590981905, 20.65937500034139873, 29.30972558990010768 ) ) ;
#10014=CARTESIAN_POINT ( 'NONE',  ( -15.40903463028480580, 36.32187500034140015, 47.42413220539094709 ) ) ;
#10015=AXIS2_PLACEMENT_3D ( 'NONE', #2668, #1506, #248 ) ;
#10017=CARTESIAN_POINT ( 'NONE',  ( -40.45084971874737789, 35.79999999999999716, -29.38926261462365730 ) ) ;
#10018=CARTESIAN_POINT ( 'NONE',  ( 49.86468353124999453, 40.95937500034140299, -16.20201782572376459 ) ) ;
#10021=CARTESIAN_POINT ( 'NONE',  ( -49.99999999999999289, 44.09999999999999432, 16.24598481164533226 ) ) ;
#10032=CARTESIAN_POINT ( 'NONE',  ( 30.81806926056962936, 39.22187500034139873, -42.41743335407647209 ) ) ;
#10033=EDGE_CURVE ( 'NONE', #12541, #40, #12496, .T. ) ;
#10036=CARTESIAN_POINT ( 'NONE',  ( 50.00000000000000000, 28.78125000068279959, -6.123233995736766085E-15 ) ) ;
#10037=CARTESIAN_POINT ( 'NONE',  ( 40.34137639590981195, 35.12187500034139731, -29.30972558990011834 ) ) ;
#10045=CARTESIAN_POINT ( 'NONE',  ( -40.45084971874737079, 24.20000000000000284, 29.38926261462367151 ) ) ;
#10047=CARTESIAN_POINT ( 'NONE',  ( -3.210462471511496205E-15, 29.35937500034139802, -52.43083105670540789 ) ) ;
#10049=CARTESIAN_POINT ( 'NONE',  ( 15.40903463028482356, 46.52187500034139589, 47.42413220539093999 ) ) ;
#10065=CARTESIAN_POINT ( 'NONE',  ( 7.919222016226693306, 32.33250428222964246, 50.00000000000003553 ) ) ;
#10072=CARTESIAN_POINT ( 'NONE',  ( -15.45084971874737256, 45.38125000068279746, -47.55282581475767500 ) ) ;
#10075=CARTESIAN_POINT ( 'NONE',  ( 15.40903463028481113, 21.25937500034139660, -47.42413220539094709 ) ) ;
#10090=ADVANCED_FACE ( 'NONE', ( #9842 ), #8198, .F. ) ;
#10093=CARTESIAN_POINT ( 'NONE',  ( -49.86468353125000164, 25.92187500034139802, 0.000000000000000000 ) ) ;
#10094=CARTESIAN_POINT ( 'NONE',  ( -49.86468353125000164, 21.85937500034139802, 0.000000000000000000 ) ) ;
#10095=CARTESIAN_POINT ( 'NONE',  ( 49.86468353125001585, 32.82187500034139305, 16.20201782572375038 ) ) ;
#10096=CARTESIAN_POINT ( 'NONE',  ( 0.000000000000000000, 20.00000000000000355, 50.00000000000000000 ) ) ;
#10097=CARTESIAN_POINT ( 'NONE',  ( 30.90169943749474157, 31.30000000000000071, -42.53254041760200721 ) ) ;
#10098=CARTESIAN_POINT ( 'NONE',  ( -30.81806926056962226, 38.15937500034138452, 42.41743335407647919 ) ) ;
#10100=CARTESIAN_POINT ( 'NONE',  ( 40.45084971874737789, 46.80000000000000426, 29.38926261462365375 ) ) ;
#10107=CARTESIAN_POINT ( 'NONE',  ( -30.90169943749474513, 33.70000000000000284, -42.53254041760200721 ) ) ;
#10111=CARTESIAN_POINT ( 'NONE',  ( 15.40903463028481113, 41.32187500034140015, -47.42413220539094709 ) ) ;
#10115=CARTESIAN_POINT ( 'NONE',  ( -30.90169943749473802, 30.08125000068279675, 42.53254041760200721 ) ) ;
#10117=CARTESIAN_POINT ( 'NONE',  ( -40.34137639590981905, 31.72187500034139873, -29.30972558990011478 ) ) ;
#10118=CARTESIAN_POINT ( 'NONE',  ( 15.45084971874737789, 38.60000000000000142, 47.55282581475767500 ) ) ;
#10119=FACE_OUTER_BOUND ( 'NONE', #2222, .T. ) ;
#10121=ORIENTED_EDGE ( 'NONE', *, *, #1424, .F. ) ;
#10127=CARTESIAN_POINT ( 'NONE',  ( 15.40903463028482356, 28.45937500034139589, 47.42413220539093999 ) ) ;
#10129=CARTESIAN_POINT ( 'NONE',  ( 49.86468353125000164, 46.92187500034139447, -6.106662507704105588E-15 ) ) ;
#10130=FACE_OUTER_BOUND ( 'NONE', #13805, .T. ) ;
#10132=CARTESIAN_POINT ( 'NONE',  ( -15.45084971874736368, 42.39999999999999858, 47.55282581475768211 ) ) ;
#10137=EDGE_LOOP ( 'NONE', ( #3046, #12256, #3737, #3314 ) ) ;
#10139=CARTESIAN_POINT ( 'NONE',  ( 40.45084971874737789, 34.58125000068280031, 29.38926261462365375 ) ) ;
#10149=CARTESIAN_POINT ( 'NONE',  ( -15.45084971874737256, 49.38125000068280457, -47.55282581475767500 ) ) ;
#10164=FACE_OUTER_BOUND ( 'NONE', #9243, .T. ) ;
#10169=CARTESIAN_POINT ( 'NONE',  ( -49.86468353125000164, 25.85937500034139802, 0.000000000000000000 ) ) ;
#10171=CARTESIAN_POINT ( 'NONE',  ( -30.81806926056962226, 38.22187500034139873, 42.41743335407647209 ) ) ;
#10173=CARTESIAN_POINT ( 'NONE',  ( 50.00000000000000000, 31.00000000000000355, -6.123233995736766085E-15 ) ) ;
#10174=CARTESIAN_POINT ( 'NONE',  ( -30.81806926056962226, 36.15937500034139163, 42.41743335407647919 ) ) ;
#10177=CARTESIAN_POINT ( 'NONE',  ( 15.45084971874737789, 44.60000000000000142, 47.55282581475767500 ) ) ;
#10191=CARTESIAN_POINT ( 'NONE',  ( -49.86468353124999453, 43.82187500034140015, -16.20201782572375393 ) ) ;
#10195=CARTESIAN_POINT ( 'NONE',  ( -30.90169943749473802, 26.08125000068279320, 42.53254041760200721 ) ) ;
#10196=CARTESIAN_POINT ( 'NONE',  ( -49.99999999999999289, 35.68125000068279462, -16.24598481164531449 ) ) ;
#10197=CARTESIAN_POINT ( 'NONE',  ( -30.81806926056962226, 36.22187500034139873, 42.41743335407647919 ) ) ;
#10199=CARTESIAN_POINT ( 'NONE',  ( -50.00000000000000000, 28.00000000000000000, 0.000000000000000000 ) ) ;
#10205=CARTESIAN_POINT ( 'NONE',  ( -15.45084971874737256, 23.60000000000000142, -47.55282581475767500 ) ) ;
#10207=CARTESIAN_POINT ( 'NONE',  ( 9.631387414534489405E-15, 30.35937500034139447, 52.43083105670540789 ) ) ;
#10210=CARTESIAN_POINT ( 'NONE',  ( 9.631387414534489405E-15, 48.42187500034139447, 52.43083105670540789 ) ) ;
#10216=VERTEX_POINT ( 'NONE', #10243 ) ;
#10217=CARTESIAN_POINT ( 'NONE',  ( -49.99999999999999289, 45.68125000068280173, -16.24598481164531449 ) ) ;
#10224=CARTESIAN_POINT ( 'NONE',  ( 0.000000000000000000, 20.00000000000000355, 50.00000000000000000 ) ) ;
#10225=CARTESIAN_POINT ( 'NONE',  ( 0.000000000000000000, 20.00000000000000355, 0.000000000000000000 ) ) ;
#10226=EDGE_CURVE ( 'NONE', #383, #9791, #8863, .T. ) ;
#10230=CYLINDRICAL_SURFACE ( 'NONE', #10728, 50.00000000000000000 ) ;
#10231=CARTESIAN_POINT ( 'NONE',  ( -30.90169943749474868, 39.48125000068278467, -42.53254041760200721 ) ) ;
#10232=CARTESIAN_POINT ( 'NONE',  ( 50.00000000000000711, 20.90000000000000213, 16.24598481164530739 ) ) ;
#10233=CARTESIAN_POINT ( 'NONE',  ( 49.99999999999999289, 46.88125000068279036, -16.24598481164532160 ) ) ;
#10243=CARTESIAN_POINT ( 'NONE',  ( -2.547328955960238000E-13, 20.49999999999999645, 49.99999999999999289 ) ) ;
#10247=DIRECTION ( 'NONE',  ( -0.000000000000000000, 1.000000000000000000, -0.000000000000000000 ) ) ;
#10248=CARTESIAN_POINT ( 'NONE',  ( -15.40903463028480580, 26.25937500034140015, 47.42413220539094709 ) ) ;
#10250=CARTESIAN_POINT ( 'NONE',  ( 30.81806926056962936, 29.22187500034139873, -42.41743335407646498 ) ) ;
#10251=CARTESIAN_POINT ( 'NONE',  ( 0.000000000000000000, 20.00000000000000355, 0.000000000000000000 ) ) ;
#10253=CARTESIAN_POINT ( 'NONE',  ( -15.45084971874736368, 30.40000000000000213, 47.55282581475768211 ) ) ;
#10254=CARTESIAN_POINT ( 'NONE',  ( -40.34137639590981905, 35.65937500034139873, -29.30972558990011478 ) ) ;
#10259=CARTESIAN_POINT ( 'NONE',  ( 50.00000000000000711, 40.89999999999999858, 16.24598481164530739 ) ) ;
#10260=ORIENTED_EDGE ( 'NONE', *, *, #1371, .T. ) ;
#10264=EDGE_LOOP ( 'NONE', ( #4859, #7213, #11230, #8844, #6060, #7299, #4106, #16134, #3665, #10945, #11705, #12921, #4721, #15110, #13039, #11331, #12756, #10930, #6119, #11222, #15386, #939, #9302, #1742, #10837, #9564, #8974, #7067, #12069, #13414, #7099, #10815, #14055, #12753 ) ) ;
#10269=PLANE ( 'NONE',  #1170 ) ;
#10275=CARTESIAN_POINT ( 'NONE',  ( -15.40903463028480580, 42.32187500034139305, 47.42413220539094709 ) ) ;
#10276=CARTESIAN_POINT ( 'NONE',  ( -49.86468353125000164, 41.85937500034139447, 0.000000000000000000 ) ) ;
#10280=CARTESIAN_POINT ( 'NONE',  ( 40.45084971874737079, 26.98125000068279888, -29.38926261462366440 ) ) ;
#10281=CARTESIAN_POINT ( 'NONE',  ( 17.39140362934560713, 24.75402226344611378, 94.04076213220706393 ) ) ;
#10282=CARTESIAN_POINT ( 'NONE',  ( -15.40903463028481646, 31.52187500034139944, -47.42413220539093999 ) ) ;
#10287=ORIENTED_EDGE ( 'NONE', *, *, #14886, .F. ) ;
#10290=ADVANCED_FACE ( 'NONE', ( #10164 ), #7669, .F. ) ;
#10295=CARTESIAN_POINT ( 'NONE',  ( -15.40903463028481646, 33.45937500034139589, -47.42413220539093999 ) ) ;
#10296=CARTESIAN_POINT ( 'NONE',  ( -3.210462471511496205E-15, 49.42187500034138736, -52.43083105670540789 ) ) ;
#10299=DIRECTION ( 'NONE',  ( -0.000000000000000000, 1.000000000000000000, -0.000000000000000000 ) ) ;
#10303=ORIENTED_EDGE ( 'NONE', *, *, #5840, .T. ) ;
#10307=( BOUNDED_CURVE ( )  B_SPLINE_CURVE ( 2, ( #984, #7403, #14949, #2148, #6083, #10893, #12220, #11228, #4504, #9642, #822, #15957, #10971 ),
 .UNSPECIFIED., .F., .F. ) 
 B_SPLINE_CURVE_WITH_KNOTS ( ( 3, 2, 2, 2, 2, 2, 3 ),
 ( 0.3166666666666667074, 0.3200000000000000067, 0.3266666666666666607, 0.3333333333333333148, 0.3400000000000000244, 0.3466666666666666785, 0.3500000000000000333 ),
 .UNSPECIFIED. ) 
 CURVE ( )  GEOMETRIC_REPRESENTATION_ITEM ( )  RATIONAL_B_SPLINE_CURVE ( ( 0.9755282581475768211, 0.9755282581475770431, 1.000000000000000000, 0.9510565162951535312, 1.000000000000000000, 0.9510565162951535312, 1.000000000000000000, 0.9510565162951535312, 1.000000000000000000, 0.9510565162951535312, 1.000000000000000000, 0.9755282581475765991, 0.9755282581475768211 ) ) 
 REPRESENTATION_ITEM ( '' )  );
#10316=DIRECTION ( 'NONE',  ( 0.000000000000000000, 0.000000000000000000, 1.000000000000000000 ) ) ;
#10317=CARTESIAN_POINT ( 'NONE',  ( 49.99999999999999289, 40.88125000068279036, -16.24598481164532160 ) ) ;
#10325=CARTESIAN_POINT ( 'NONE',  ( 7.513064459987437071E-14, 42.50000000000000000, 50.00000000000000000 ) ) ;
#10327=ORIENTED_EDGE ( 'NONE', *, *, #14864, .T. ) ;
#10329=CYLINDRICAL_SURFACE ( 'NONE', #2554, 50.00000000000000000 ) ;
#10330=CARTESIAN_POINT ( 'NONE',  ( -5.642626679385776889, 39.07526700153634636, 92.94045629140883591 ) ) ;
#10333=CARTESIAN_POINT ( 'NONE',  ( -40.45084971874737079, 37.98125000068279888, 29.38926261462367151 ) ) ;
#10334=CARTESIAN_POINT ( 'NONE',  ( 15.40903463028482356, 22.45937500034139589, 47.42413220539093999 ) ) ;
#10336=CARTESIAN_POINT ( 'NONE',  ( -40.34137639590981195, 28.12187500034139731, 29.30972558990012189 ) ) ;
#10338=CARTESIAN_POINT ( 'NONE',  ( -30.90169943749473802, 28.30000000000000071, 42.53254041760200721 ) ) ;
#10339=CARTESIAN_POINT ( 'NONE',  ( -49.86468353124999453, 31.75937500034140015, -16.20201782572375393 ) ) ;
#10351=CARTESIAN_POINT ( 'NONE',  ( -40.34137639590981195, 36.12187500034139731, 29.30972558990012189 ) ) ;
#10352=CARTESIAN_POINT ( 'NONE',  ( -40.34137639590981195, 42.05937500034139731, 29.30972558990012189 ) ) ;
#10355=CARTESIAN_POINT ( 'NONE',  ( 50.00000000000000000, 22.78125000068279959, -6.123233995736766085E-15 ) ) ;
#10359=CARTESIAN_POINT ( 'NONE',  ( -40.34137639590981195, 26.12187500034139731, 29.30972558990012189 ) ) ;
#10360=CARTESIAN_POINT ( 'NONE',  ( -7.919222016226804328, 28.22999571913594963, 50.00000000000000000 ) ) ;
#10369=( BOUNDED_CURVE ( )  B_SPLINE_CURVE ( 2, ( #45, #4988, #11133, #9958, #3648, #2299, #13770, #13930, #1046, #7707, #4823, #8869, #5073 ),
 .UNSPECIFIED., .F., .F. ) 
 B_SPLINE_CURVE_WITH_KNOTS ( ( 3, 2, 2, 2, 2, 2, 3 ),
 ( 0.8500000000000000888, 0.8533333333333333881, 0.8599999999999999867, 0.8666666666666666963, 0.8733333333333332948, 0.8800000000000000044, 0.8833333333333334147 ),
 .UNSPECIFIED. ) 
 CURVE ( )  GEOMETRIC_REPRESENTATION_ITEM ( )  RATIONAL_B_SPLINE_CURVE ( ( 0.9755282581475768211, 0.9755282581475771542, 1.000000000000000000, 0.9510565162951535312, 1.000000000000000000, 0.9510565162951535312, 1.000000000000000000, 0.9510565162951535312, 1.000000000000000000, 0.9510565162951535312, 1.000000000000000000, 0.9755282581475763770, 0.9755282581475768211 ) ) 
 REPRESENTATION_ITEM ( '' )  );
#10370=CARTESIAN_POINT ( 'NONE',  ( -49.86468353124999453, 25.95937500034139944, 16.20201782572377525 ) ) ;
#10374=CARTESIAN_POINT ( 'NONE',  ( 30.81806926056962936, 45.22187500034139873, -42.41743335407646498 ) ) ;
#10378=CARTESIAN_POINT ( 'NONE',  ( -49.86468353125000164, 47.92187500034139447, 0.000000000000000000 ) ) ;
#10388=DIRECTION ( 'NONE',  ( 0.000000000000000000, 0.000000000000000000, 1.000000000000000000 ) ) ;
#10391=CARTESIAN_POINT ( 'NONE',  ( -49.99999999999999289, 25.89999999999999858, -16.24598481164531449 ) ) ;
#10392=CARTESIAN_POINT ( 'NONE',  ( 15.40903463028481113, 49.25937500034139305, -47.42413220539094709 ) ) ;
#10394=CARTESIAN_POINT ( 'NONE',  ( 0.000000000000000000, 20.00000000000000355, 50.00000000000000000 ) ) ;
#10395=CARTESIAN_POINT ( 'NONE',  ( -49.86468353124999453, 24.02187500034139589, 16.20201782572377525 ) ) ;
#10397=CARTESIAN_POINT ( 'NONE',  ( -49.99999999999999289, 37.68125000068278752, -16.24598481164531449 ) ) ;
#10406=EDGE_CURVE ( 'NONE', #12541, #4002, #2874, .T. ) ;
#10415=CARTESIAN_POINT ( 'NONE',  ( -49.99999999999999289, 29.88125000068279391, 16.24598481164533226 ) ) ;
#10418=CARTESIAN_POINT ( 'NONE',  ( -47.69912754770682284, 20.00000000000000355, 14.53642574140364019 ) ) ;
#10420=CARTESIAN_POINT ( 'NONE',  ( 40.34137639590981905, 26.72187500034139518, 29.30972558990010768 ) ) ;
#10422=CARTESIAN_POINT ( 'NONE',  ( -15.45084971874737256, 33.60000000000000142, -47.55282581475767500 ) ) ;
#10423=CARTESIAN_POINT ( 'NONE',  ( -40.34137639590981905, 33.65937500034139873, -29.30972558990011478 ) ) ;
#10431=CARTESIAN_POINT ( 'NONE',  ( -49.99999999999999289, 38.10000000000000142, 16.24598481164533226 ) ) ;
#10434=CARTESIAN_POINT ( 'NONE',  ( 40.34137639590981195, 39.12187500034139731, -29.30972558990011834 ) ) ;
#10435=CARTESIAN_POINT ( 'NONE',  ( -40.34137639590981905, 43.65937500034139163, -29.30972558990011478 ) ) ;
#10436=CARTESIAN_POINT ( 'NONE',  ( -50.00000000000000000, 44.00000000000000711, 0.000000000000000000 ) ) ;
#10439=CARTESIAN_POINT ( 'NONE',  ( -30.90169943749473802, 20.08125000068279320, 42.53254041760200721 ) ) ;
#10441=CARTESIAN_POINT ( 'NONE',  ( 15.40903463028482356, 30.52187500034139589, 47.42413220539093999 ) ) ;
#10442=CARTESIAN_POINT ( 'NONE',  ( -7.919222016226804328, 28.44874571845315003, 50.00000000000000000 ) ) ;
#10443=ORIENTED_EDGE ( 'NONE', *, *, #7269, .F. ) ;
#10451=CARTESIAN_POINT ( 'NONE',  ( -30.81806926056962226, 22.15937500034139873, 42.41743335407647919 ) ) ;
#10453=CARTESIAN_POINT ( 'NONE',  ( 49.86468353124999453, 39.02187500034138878, -16.20201782572376104 ) ) ;
#10457=CARTESIAN_POINT ( 'NONE',  ( -15.40903463028480580, 48.32187500034140015, 47.42413220539094709 ) ) ;
#10466=CARTESIAN_POINT ( 'NONE',  ( 30.90169943749475223, 38.48125000068279888, 42.53254041760199300 ) ) ;
#10469=CARTESIAN_POINT ( 'NONE',  ( -3.219174618344376363E-15, 27.50000000000000355, -52.57311121191334990 ) ) ;
#10470=CARTESIAN_POINT ( 'NONE',  ( -30.81806926056962226, 42.15937500034139163, 42.41743335407647919 ) ) ;
#10471=CARTESIAN_POINT ( 'NONE',  ( -40.45084971874737079, 25.98125000068279888, 29.38926261462367151 ) ) ;
#10473=LINE ( 'NONE', #9390, #11595 ) ;
#10475=CARTESIAN_POINT ( 'NONE',  ( -15.45084971874736368, 40.18125000068280173, 47.55282581475768211 ) ) ;
#10485=ORIENTED_EDGE ( 'NONE', *, *, #12974, .F. ) ;
#10490=ORIENTED_EDGE ( 'NONE', *, *, #7836, .T. ) ;
#10494=CARTESIAN_POINT ( 'NONE',  ( 15.45084971874737789, 22.60000000000000142, 47.55282581475767500 ) ) ;
#10501=CARTESIAN_POINT ( 'NONE',  ( -47.02241032844462154, 19.99999999999999645, 16.59456509147196357 ) ) ;
#10502=CARTESIAN_POINT ( 'NONE',  ( -49.86468353125000164, 25.92187500034139802, 0.000000000000000000 ) ) ;
#10506=CARTESIAN_POINT ( 'NONE',  ( 15.40903463028482356, 30.45937500034139589, 47.42413220539093999 ) ) ;
#10507=CARTESIAN_POINT ( 'NONE',  ( 30.90169943749475223, 38.69999999999999574, 42.53254041760199300 ) ) ;
#10509=AXIS2_PLACEMENT_3D ( 'NONE', #7887, #5492, #14517 ) ;
#10520=CARTESIAN_POINT ( 'NONE',  ( 49.86468353124999453, 33.02187500034139589, -16.20201782572376459 ) ) ;
#10521=CARTESIAN_POINT ( 'NONE',  ( 15.40903463028481113, 35.25937500034139305, -47.42413220539094709 ) ) ;
#10527=CARTESIAN_POINT ( 'NONE',  ( 9.657523855033129090E-15, 20.28125000068279959, 52.57311121191334990 ) ) ;
#10530=CARTESIAN_POINT ( 'NONE',  ( 40.34137639590981905, 26.72187500034139518, 29.30972558990010768 ) ) ;
#10538=CARTESIAN_POINT ( 'NONE',  ( -2.547328955960238000E-13, 30.28125000068279604, 49.99999999999999289 ) ) ;
#10544=CARTESIAN_POINT ( 'NONE',  ( -30.81806926056963292, 27.55937500034139376, -42.41743335407647209 ) ) ;
#10546=CARTESIAN_POINT ( 'NONE',  ( -49.86468353124999453, 40.02187500034139589, 16.20201782572377169 ) ) ;
#10549=CARTESIAN_POINT ( 'NONE',  ( 0.000000000000000000, 20.00000000000000355, 0.000000000000000000 ) ) ;
#10551=CARTESIAN_POINT ( 'NONE',  ( 30.81806926056964002, 44.62187500034140442, 42.41743335407647209 ) ) ;
#10553=ORIENTED_EDGE ( 'NONE', *, *, #4595, .T. ) ;
#10555=ORIENTED_EDGE ( 'NONE', *, *, #12236, .T. ) ;
#10563=CARTESIAN_POINT ( 'NONE',  ( 50.00000000000000711, 22.90000000000000213, 16.24598481164530739 ) ) ;
#10564=CARTESIAN_POINT ( 'NONE',  ( 49.86468353124999453, 44.95937500034139589, -16.20201782572376459 ) ) ;
#10565=CARTESIAN_POINT ( 'NONE',  ( 8.446640517145639571E-15, 26.28125000068279959, 50.00000000000000000 ) ) ;
#10569=CARTESIAN_POINT ( 'NONE',  ( -49.99999999999999289, 39.68125000068280173, -16.24598481164531449 ) ) ;
#10576=VERTEX_POINT ( 'NONE', #16292 ) ;
#10577=DIRECTION ( 'NONE',  ( 0.000000000000000000, 0.000000000000000000, 1.000000000000000000 ) ) ;
#10580=VERTEX_POINT ( 'NONE', #8555 ) ;
#10587=CARTESIAN_POINT ( 'NONE',  ( 4.613455220948956104, 5.578608468406812904, 98.91547126341453122 ) ) ;
#10588=CARTESIAN_POINT ( 'NONE',  ( -48.24365308685478482, 20.00000000000001066, 12.61207274729074790 ) ) ;
#10589=CARTESIAN_POINT ( 'NONE',  ( -49.86468353124999453, 29.82187500034139660, -16.20201782572375393 ) ) ;
#10591=CARTESIAN_POINT ( 'NONE',  ( -15.45084971874737256, 21.60000000000000142, -47.55282581475767500 ) ) ;
#10593=CARTESIAN_POINT ( 'NONE',  ( -15.40903463028481646, 29.45937500034139589, -47.42413220539093999 ) ) ;
#10595=AXIS2_PLACEMENT_3D ( 'NONE', #8462, #1962, #13527 ) ;
#10597=VERTEX_POINT ( 'NONE', #12145 ) ;
#10606=CIRCLE ( 'NONE', #7148, 85.01963570546854498 ) ;
#10607=CARTESIAN_POINT ( 'NONE',  ( -3.210462471511496205E-15, 37.42187500034140157, -52.43083105670540789 ) ) ;
#10608=CARTESIAN_POINT ( 'NONE',  ( 40.34137639590981195, 35.05937500034139731, -29.30972558990011834 ) ) ;
#10611=CARTESIAN_POINT ( 'NONE',  ( -49.99999999999999289, 21.88125000068280102, 16.24598481164533226 ) ) ;
#10613=CARTESIAN_POINT ( 'NONE',  ( 40.34137639590981195, 27.12187500034139731, -29.30972558990011834 ) ) ;
#10614=VECTOR ( 'NONE', #16441, 1000.000000000000000 ) ;
#10619=VERTEX_POINT ( 'NONE', #904 ) ;
#10621=CARTESIAN_POINT ( 'NONE',  ( -17.50000000000000000, 22.50000000000000000, 94.42467108177066848 ) ) ;
#10622=CARTESIAN_POINT ( 'NONE',  ( -49.99999999999999289, 33.68125000068278752, -16.24598481164531449 ) ) ;
#10624=CARTESIAN_POINT ( 'NONE',  ( 40.34137639590981195, 27.05937500034139731, -29.30972558990011834 ) ) ;
#10626=CARTESIAN_POINT ( 'NONE',  ( 30.81806926056962936, 41.22187500034139873, -42.41743335407646498 ) ) ;
#10629=CARTESIAN_POINT ( 'NONE',  ( -30.81806926056962226, 48.22187500034139163, 42.41743335407647919 ) ) ;
#10637=DIRECTION ( 'NONE',  ( 0.000000000000000000, 0.000000000000000000, -1.000000000000000000 ) ) ;
#10638=CARTESIAN_POINT ( 'NONE',  ( 6.123233995736766085E-15, 20.00000000000000355, -50.00000000000000000 ) ) ;
#10639=CARTESIAN_POINT ( 'NONE',  ( 30.90169943749474157, 27.29999999999999716, -42.53254041760200721 ) ) ;
#10640=CARTESIAN_POINT ( 'NONE',  ( 40.34137639590981195, 47.05937500034140442, -29.30972558990011834 ) ) ;
#10645=CARTESIAN_POINT ( 'NONE',  ( -3.219174618344376363E-15, 37.28125000068280315, -52.57311121191334990 ) ) ;
#10666=CARTESIAN_POINT ( 'NONE',  ( -47.29342682910125717, 19.99999999999999645, 15.80652463092984839 ) ) ;
#10667=CARTESIAN_POINT ( 'NONE',  ( -15.40903463028480580, 22.32187500034139660, 47.42413220539094709 ) ) ;
#10670=CARTESIAN_POINT ( 'NONE',  ( -15.40903463028481646, 33.45937500034139589, -47.42413220539093999 ) ) ;
#10680=CARTESIAN_POINT ( 'NONE',  ( -30.81806926056962226, 36.22187500034139873, 42.41743335407647919 ) ) ;
#10681=CARTESIAN_POINT ( 'NONE',  ( 40.34137639590981195, 37.05937500034139731, -29.30972558990011834 ) ) ;
#10682=CARTESIAN_POINT ( 'NONE',  ( -49.99999999999999289, 43.89999999999999858, -16.24598481164531449 ) ) ;
#10684=CARTESIAN_POINT ( 'NONE',  ( -40.45084971874737079, 23.98125000068279888, 29.38926261462367151 ) ) ;
#10686=ADVANCED_FACE ( 'NONE', ( #4765 ), #4670, .F. ) ;
#10687=CARTESIAN_POINT ( 'NONE',  ( 30.81806926056964002, 30.62187500034139020, 42.41743335407647209 ) ) ;
#10695=CARTESIAN_POINT ( 'NONE',  ( -30.90169943749473447, 34.08125000068279320, 42.53254041760200721 ) ) ;
#10697=CARTESIAN_POINT ( 'NONE',  ( 49.86468353124999453, 26.95937500034139944, -16.20201782572376459 ) ) ;
#10699=CARTESIAN_POINT ( 'NONE',  ( 50.00000000000000000, 35.00000000000000000, -6.123233995736766085E-15 ) ) ;
#10700=CARTESIAN_POINT ( 'NONE',  ( -49.86468353124999453, 44.02187500034139589, 16.20201782572377525 ) ) ;
#10709=CARTESIAN_POINT ( 'NONE',  ( 0.000000000000000000, 20.00000000000000355, 50.00000000000000000 ) ) ;
#10712=CARTESIAN_POINT ( 'NONE',  ( -15.45084971874736368, 22.39999999999999858, 47.55282581475768211 ) ) ;
#10713=CARTESIAN_POINT ( 'NONE',  ( 49.86468353125001585, 44.75937500034138594, 16.20201782572375038 ) ) ;
#10714=CARTESIAN_POINT ( 'NONE',  ( -15.40903463028481646, 49.45937500034140299, -47.42413220539093999 ) ) ;
#10719=CARTESIAN_POINT ( 'NONE',  ( -7.919222016226816763, 45.55125428154684641, -49.99999999999999289 ) ) ;
#10720=CARTESIAN_POINT ( 'NONE',  ( 50.00000000000000711, 46.68125000068279462, 16.24598481164530739 ) ) ;
#10728=AXIS2_PLACEMENT_3D ( 'NONE', #12724, #8983, #11318 ) ;
#10738=( BOUNDED_CURVE ( )  B_SPLINE_CURVE ( 2, ( #4581, #4204, #9645, #4111, #5542, #10431, #10896, #6701, #12926, #4282, #9267, #9181, #745 ),
 .UNSPECIFIED., .F., .F. ) 
 B_SPLINE_CURVE_WITH_KNOTS ( ( 3, 2, 2, 2, 2, 2, 3 ),
 ( 0.3833333333333333592, 0.3866666666666666585, 0.3933333333333333126, 0.4000000000000000222, 0.4066666666666666763, 0.4133333333333333304, 0.4166666666666666852 ),
 .UNSPECIFIED. ) 
 CURVE ( )  GEOMETRIC_REPRESENTATION_ITEM ( )  RATIONAL_B_SPLINE_CURVE ( ( 0.9755282581475768211, 0.9755282581475770431, 1.000000000000000000, 0.9510565162951535312, 1.000000000000000000, 0.9510565162951535312, 1.000000000000000000, 0.9510565162951535312, 1.000000000000000000, 0.9510565162951535312, 1.000000000000000000, 0.9755282581475765991, 0.9755282581475768211 ) ) 
 REPRESENTATION_ITEM ( '' )  );
#10741=CARTESIAN_POINT ( 'NONE',  ( 15.96528350601207613, 15.31079395116513986, 95.98183428236838211 ) ) ;
#10742=DIRECTION ( 'NONE',  ( -0.000000000000000000, 1.000000000000000000, -0.000000000000000000 ) ) ;
#10743=CARTESIAN_POINT ( 'NONE',  ( 30.81806926056964002, 20.62187500034139020, 42.41743335407646498 ) ) ;
#10744=CARTESIAN_POINT ( 'NONE',  ( -40.45084971874737789, 21.80000000000000071, -29.38926261462365730 ) ) ;
#10747=CARTESIAN_POINT ( 'NONE',  ( -30.81806926056962226, 24.15937500034139873, 42.41743335407647919 ) ) ;
#10758=CARTESIAN_POINT ( 'NONE',  ( -30.81806926056962226, 28.22187500034139873, 42.41743335407647919 ) ) ;
#10759=CARTESIAN_POINT ( 'NONE',  ( 15.40903463028482356, 34.45937500034139589, 47.42413220539093999 ) ) ;
#10760=CARTESIAN_POINT ( 'NONE',  ( -2.547328955960238000E-13, 32.50000000000000000, 49.99999999999999289 ) ) ;
#10763=CARTESIAN_POINT ( 'NONE',  ( 30.81806926056964002, 46.55937500034139020, 42.41743335407647209 ) ) ;
#10765=VECTOR ( 'NONE', #9942, 1000.000000000000000 ) ;
#10767=CARTESIAN_POINT ( 'NONE',  ( 50.00000000000000711, 48.90000000000000568, 16.24598481164530739 ) ) ;
#10768=ORIENTED_EDGE ( 'NONE', *, *, #9148, .T. ) ;
#10777=CARTESIAN_POINT ( 'NONE',  ( 30.90169943749473802, 31.08125000068280031, -42.53254041760200721 ) ) ;
#10779=CARTESIAN_POINT ( 'NONE',  ( 30.81806926056962936, 21.15937500034140228, -42.41743335407647209 ) ) ;
#10783=CARTESIAN_POINT ( 'NONE',  ( 9.657523855033129090E-15, 34.50000000000000711, 52.57311121191334990 ) ) ;
#10786=CARTESIAN_POINT ( 'NONE',  ( -49.86468353124999453, 41.82187500034140015, -16.20201782572375393 ) ) ;
#10788=CARTESIAN_POINT ( 'NONE',  ( 30.90169943749475223, 30.70000000000000284, 42.53254041760199300 ) ) ;
#10796=ORIENTED_EDGE ( 'NONE', *, *, #13545, .T. ) ;
#10799=CARTESIAN_POINT ( 'NONE',  ( -1.240322475938754499E-13, 40.28125000068280315, 50.00000000000000000 ) ) ;
#10802=CARTESIAN_POINT ( 'NONE',  ( 40.45084971874737789, 20.80000000000000426, 29.38926261462365375 ) ) ;
#10803=CARTESIAN_POINT ( 'NONE',  ( -30.81806926056962226, 44.15937500034139163, 42.41743335407647919 ) ) ;
#10805=CARTESIAN_POINT ( 'NONE',  ( 49.86468353125000164, 46.85937500034139447, -6.106662507704105588E-15 ) ) ;
#10809=CARTESIAN_POINT ( 'NONE',  ( -49.99999999999999289, 45.90000000000000568, -16.24598481164531449 ) ) ;
#10810=CARTESIAN_POINT ( 'NONE',  ( 49.99999999999999289, 22.88125000068280102, -16.24598481164532160 ) ) ;
#10815=ORIENTED_EDGE ( 'NONE', *, *, #6844, .F. ) ;
#10826=CARTESIAN_POINT ( 'NONE',  ( -50.00000000000000000, 48.00000000000000000, 0.000000000000000000 ) ) ;
#10827=CARTESIAN_POINT ( 'NONE',  ( -2.445080149700054274E-14, 46.50000000000000711, 50.00000000000000000 ) ) ;
#10829=CARTESIAN_POINT ( 'NONE',  ( -49.86468353124999453, 21.82187500034139305, -16.20201782572375393 ) ) ;
#10832=CARTESIAN_POINT ( 'NONE',  ( 49.86468353125000164, 24.85937500034139802, -6.106662507704105588E-15 ) ) ;
#10833=CARTESIAN_POINT ( 'NONE',  ( 8.446640517145639571E-15, 26.28125000068279959, 50.00000000000000000 ) ) ;
#10837=ORIENTED_EDGE ( 'NONE', *, *, #8778, .F. ) ;
#10839=( BOUNDED_CURVE ( )  B_SPLINE_CURVE ( 2, ( #13022, #7949, #14172, #6554, #11767, #211, #4219, #764, #7866, #4127, #11614, #5854, #14260 ),
 .UNSPECIFIED., .F., .F. ) 
 B_SPLINE_CURVE_WITH_KNOTS ( ( 3, 2, 2, 2, 2, 2, 3 ),
 ( 0.01666666666666666990, 0.02000000000000000042, 0.02666666666666666838, 0.03333333333333333287, 0.04000000000000000083, 0.04666666666666667573, 0.05000000000000000278 ),
 .UNSPECIFIED. ) 
 CURVE ( )  GEOMETRIC_REPRESENTATION_ITEM ( )  RATIONAL_B_SPLINE_CURVE ( ( 0.9755282581475768211, 0.9755282581475768211, 1.000000000000000000, 0.9510565162951535312, 1.000000000000000000, 0.9510565162951535312, 1.000000000000000000, 0.9510565162951535312, 1.000000000000000000, 0.9510565162951535312, 1.000000000000000000, 0.9755282581475768211, 0.9755282581475768211 ) ) 
 REPRESENTATION_ITEM ( '' )  );
#10843=CARTESIAN_POINT ( 'NONE',  ( 30.81806926056964002, 26.62187500034139731, 42.41743335407647209 ) ) ;
#10844=CARTESIAN_POINT ( 'NONE',  ( -15.40903463028481646, 33.45937500034139589, -47.42413220539093999 ) ) ;
#10845=CYLINDRICAL_SURFACE ( 'NONE', #9234, 17.50000000000000000 ) ;
#10848=CARTESIAN_POINT ( 'NONE',  ( 49.86468353125000164, 42.85937500034140157, -6.106662507704105588E-15 ) ) ;
#10850=CARTESIAN_POINT ( 'NONE',  ( -30.81806926056963292, 21.62187500034139376, -42.41743335407647209 ) ) ;
#10859=CARTESIAN_POINT ( 'NONE',  ( -40.34137639590981195, 46.12187500034139731, 29.30972558990012189 ) ) ;
#10864=CARTESIAN_POINT ( 'NONE',  ( 15.45084971874736723, 39.40000000000000568, -47.55282581475768211 ) ) ;
#10866=CARTESIAN_POINT ( 'NONE',  ( -40.34137639590981905, 39.72187500034139873, -29.30972558990011478 ) ) ;
#10874=DIRECTION ( 'NONE',  ( 0.000000000000000000, 0.000000000000000000, 1.000000000000000000 ) ) ;
#10879=CARTESIAN_POINT ( 'NONE',  ( 15.40903463028482356, 40.45937500034139589, 47.42413220539093999 ) ) ;
#10884=CARTESIAN_POINT ( 'NONE',  ( 30.90169943749473802, 37.29999999999999716, -42.53254041760200721 ) ) ;
#10893=CARTESIAN_POINT ( 'NONE',  ( -49.99999999999999289, 40.09999999999999432, 16.24598481164533226 ) ) ;
#10894=CARTESIAN_POINT ( 'NONE',  ( 40.45084971874737079, 29.19999999999999929, -29.38926261462366440 ) ) ;
#10896=CARTESIAN_POINT ( 'NONE',  ( -50.00000000000000000, 38.00000000000000711, 0.000000000000000000 ) ) ;
#10898=CARTESIAN_POINT ( 'NONE',  ( -50.00000000000000000, 20.00000000000000000, 0.000000000000000000 ) ) ;
#10904=CARTESIAN_POINT ( 'NONE',  ( 7.919222016226807881, 46.55125428154685352, 50.00000000000000000 ) ) ;
#10905=CARTESIAN_POINT ( 'NONE',  ( -38.60409515610530917, 20.00000000000000355, 31.77615201968871617 ) ) ;
#10906=CARTESIAN_POINT ( 'NONE',  ( -49.86468353124999453, 25.82187500034139305, -16.20201782572375393 ) ) ;
#10909=CARTESIAN_POINT ( 'NONE',  ( 49.86468353125000164, 22.85937500034139802, -6.106662507704105588E-15 ) ) ;
#10915=CARTESIAN_POINT ( 'NONE',  ( 7.919222016226822092, 48.55125428154684641, 49.99999999999999289 ) ) ;
#10919=CARTESIAN_POINT ( 'NONE',  ( 30.90169943749475223, 28.48125000068279888, 42.53254041760199300 ) ) ;
#10921=CARTESIAN_POINT ( 'NONE',  ( 49.86468353125000164, 30.92187500034139802, -6.106662507704105588E-15 ) ) ;
#10922=CARTESIAN_POINT ( 'NONE',  ( 40.34137639590981195, 31.05937500034139731, -29.30972558990011834 ) ) ;
#10923=CARTESIAN_POINT ( 'NONE',  ( -40.45084971874737789, 35.79999999999999716, -29.38926261462365730 ) ) ;
#10926=CARTESIAN_POINT ( 'NONE',  ( 15.40903463028482356, 46.45937500034139589, 47.42413220539093999 ) ) ;
#10928=CARTESIAN_POINT ( 'NONE',  ( 9.631387414534489405E-15, 20.42187500034139802, 52.43083105670540789 ) ) ;
#10929=( BOUNDED_CURVE ( )  B_SPLINE_CURVE ( 2, ( #7404, #9817, #743, #5829, #10894, #12473, #15958, #16038, #4665, #16133, #13465, #12221, #4760 ),
 .UNSPECIFIED., .F., .F. ) 
 B_SPLINE_CURVE_WITH_KNOTS ( ( 3, 2, 2, 2, 2, 2, 3 ),
 ( 0.6833333333333333481, 0.6866666666666666474, 0.6933333333333333570, 0.6999999999999999556, 0.7066666666666666652, 0.7133333333333333748, 0.7166666666666666741 ),
 .UNSPECIFIED. ) 
 CURVE ( )  GEOMETRIC_REPRESENTATION_ITEM ( )  RATIONAL_B_SPLINE_CURVE ( ( 0.9755282581475768211, 0.9755282581475768211, 1.000000000000000000, 0.9510565162951535312, 1.000000000000000000, 0.9510565162951535312, 1.000000000000000000, 0.9510565162951535312, 1.000000000000000000, 0.9510565162951535312, 1.000000000000000000, 0.9755282581475768211, 0.9755282581475768211 ) ) 
 REPRESENTATION_ITEM ( '' )  );
#10930=ORIENTED_EDGE ( 'NONE', *, *, #6252, .F. ) ;
#10932=ORIENTED_EDGE ( 'NONE', *, *, #1295, .T. ) ;
#10937=CARTESIAN_POINT ( 'NONE',  ( -30.81806926056962226, 20.15937500034139518, 42.41743335407647919 ) ) ;
#10941=CARTESIAN_POINT ( 'NONE',  ( 30.90169943749474157, 35.08125000068278609, -42.53254041760200721 ) ) ;
#10942=CARTESIAN_POINT ( 'NONE',  ( -40.45084971874737789, 39.80000000000000426, -29.38926261462365730 ) ) ;
#10943=CARTESIAN_POINT ( 'NONE',  ( -40.34137639590981905, 41.72187500034139873, -29.30972558990011478 ) ) ;
#10945=ORIENTED_EDGE ( 'NONE', *, *, #8288, .F. ) ;
#10954=CARTESIAN_POINT ( 'NONE',  ( -3.111920190527341144E-15, 27.50000000000000000, -50.00000000000000000 ) ) ;
#10955=CARTESIAN_POINT ( 'NONE',  ( -3.219174618344376363E-15, 21.50000000000000355, -52.57311121191334990 ) ) ;
#10956=CARTESIAN_POINT ( 'NONE',  ( 49.86468353125001585, 34.75937500034139305, 16.20201782572375038 ) ) ;
#10957=DIRECTION ( 'NONE',  ( -0.000000000000000000, 1.000000000000000000, -0.000000000000000000 ) ) ;
#10961=CARTESIAN_POINT ( 'NONE',  ( -40.45084971874737789, 45.79999999999999716, -29.38926261462365730 ) ) ;
#10963=CARTESIAN_POINT ( 'NONE',  ( 40.45084971874737789, 36.79999999999999716, 29.38926261462365375 ) ) ;
#10965=ORIENTED_EDGE ( 'NONE', *, *, #16383, .T. ) ;
#10971=CARTESIAN_POINT ( 'NONE',  ( 1.293669679204937499E-13, 39.50000000000000711, -50.00000000000000000 ) ) ;
#10975=CARTESIAN_POINT ( 'NONE',  ( -7.919222016226802552, 47.33250428222964956, -50.00000000000000000 ) ) ;
#10977=CARTESIAN_POINT ( 'NONE',  ( -1.158672503420370870, 5.028666560261853213, 99.10823753331240482 ) ) ;
#10980=CYLINDRICAL_SURFACE ( 'NONE', #12171, 50.00000000000000000 ) ;
#10981=ADVANCED_FACE ( 'NONE', ( #1117 ), #4736, .F. ) ;
#10982=CARTESIAN_POINT ( 'NONE',  ( -7.919222016226688865, 31.55125428154684286, -50.00000000000003553 ) ) ;
#10983=CARTESIAN_POINT ( 'NONE',  ( 30.90169943749475223, 46.69999999999999574, 42.53254041760199300 ) ) ;
#10985=CARTESIAN_POINT ( 'NONE',  ( 40.34137639590981195, 21.12187500034139376, -29.30972558990011834 ) ) ;
#10988=CARTESIAN_POINT ( 'NONE',  ( 9.631387414534489405E-15, 26.35937500034140157, 52.43083105670540789 ) ) ;
#10991=AXIS2_PLACEMENT_3D ( 'NONE', #3587, #3675, #10316 ) ;
#10999=DIRECTION ( 'NONE',  ( 0.000000000000000000, 0.000000000000000000, 1.000000000000000000 ) ) ;
#11002=CARTESIAN_POINT ( 'NONE',  ( 15.45084971874736723, 29.18125000068279817, -47.55282581475768211 ) ) ;
#11004=CARTESIAN_POINT ( 'NONE',  ( 15.40903463028482356, 28.52187500034139589, 47.42413220539093999 ) ) ;
#11005=CARTESIAN_POINT ( 'NONE',  ( -49.86468353124999453, 27.95937500034139944, 16.20201782572377169 ) ) ;
#11006=CARTESIAN_POINT ( 'NONE',  ( -3.111920190527341144E-15, 35.50000000000000000, -50.00000000000000000 ) ) ;
#11009=CARTESIAN_POINT ( 'NONE',  ( 30.81806926056962936, 45.15937500034139873, -42.41743335407647209 ) ) ;
#11011=CARTESIAN_POINT ( 'NONE',  ( -30.81806926056962226, 22.22187500034139163, 42.41743335407647919 ) ) ;
#11012=ORIENTED_EDGE ( 'NONE', *, *, #12207, .F. ) ;
#11021=CARTESIAN_POINT ( 'NONE',  ( 30.81806926056964002, 20.55937500034139376, 42.41743335407647209 ) ) ;
#11026=CARTESIAN_POINT ( 'NONE',  ( 49.99999999999999289, 36.88125000068279036, -16.24598481164532160 ) ) ;
#11028=CARTESIAN_POINT ( 'NONE',  ( 40.34137639590981905, 42.72187500034139873, 29.30972558990010768 ) ) ;
#11032=DIRECTION ( 'NONE',  ( 0.000000000000000000, 0.000000000000000000, -1.000000000000000000 ) ) ;
#11040=CARTESIAN_POINT ( 'NONE',  ( -15.45084971874736368, 22.18125000068279817, 47.55282581475768211 ) ) ;
#11041=CARTESIAN_POINT ( 'NONE',  ( -40.45084971874737079, 20.20000000000000284, 29.38926261462367151 ) ) ;
#11042=CARTESIAN_POINT ( 'NONE',  ( 49.86468353124999453, 38.95937500034139589, -16.20201782572376459 ) ) ;
#11043=CARTESIAN_POINT ( 'NONE',  ( -30.81806926056963292, 49.55937500034139731, -42.41743335407646498 ) ) ;
#11050=DIRECTION ( 'NONE',  ( 0.000000000000000000, 1.000000000000000000, 0.000000000000000000 ) ) ;
#11059=ORIENTED_EDGE ( 'NONE', *, *, #3983, .F. ) ;
#11060=ORIENTED_EDGE ( 'NONE', *, *, #159, .F. ) ;
#11064=EDGE_LOOP ( 'NONE', ( #10260, #15594, #13158, #9873 ) ) ;
#11065=LINE ( 'NONE', #1067, #5451 ) ;
#11067=CARTESIAN_POINT ( 'NONE',  ( 0.000000000000000000, 20.00000000000000355, 0.000000000000000000 ) ) ;
#11068=DIRECTION ( 'NONE',  ( -0.000000000000000000, 1.000000000000000000, -0.000000000000000000 ) ) ;
#11072=CARTESIAN_POINT ( 'NONE',  ( -30.90169943749473447, 32.30000000000000426, 42.53254041760200721 ) ) ;
#11073=DIRECTION ( 'NONE',  ( 0.000000000000000000, 0.000000000000000000, 1.000000000000000000 ) ) ;
#11075=CARTESIAN_POINT ( 'NONE',  ( 15.45084971874736723, 47.18125000068280173, -47.55282581475768211 ) ) ;
#11078=VECTOR ( 'NONE', #10742, 1000.000000000000000 ) ;
#11079=CARTESIAN_POINT ( 'NONE',  ( 40.34137639590981905, 24.65937500034139873, 29.30972558990010768 ) ) ;
#11081=CARTESIAN_POINT ( 'NONE',  ( -40.45084971874737079, 41.98125000068279888, 29.38926261462367151 ) ) ;
#11085=EDGE_CURVE ( 'NONE', #13440, #10580, #8845, .T. ) ;
#11090=CIRCLE ( 'NONE', #2300, 50.00000000000000000 ) ;
#11098=CARTESIAN_POINT ( 'NONE',  ( -30.81806926056963292, 27.62187500034139731, -42.41743335407647209 ) ) ;
#11099=CARTESIAN_POINT ( 'NONE',  ( 15.40903463028481113, 27.25937500034139660, -47.42413220539094709 ) ) ;
#11100=CARTESIAN_POINT ( 'NONE',  ( 40.45084971874737789, 26.58125000068279675, 29.38926261462365375 ) ) ;
#11101=CARTESIAN_POINT ( 'NONE',  ( -30.81806926056963292, 33.62187500034139731, -42.41743335407646498 ) ) ;
#11102=DIRECTION ( 'NONE',  ( 0.000000000000000000, 0.000000000000000000, 1.000000000000000000 ) ) ;
#11105=CARTESIAN_POINT ( 'NONE',  ( -30.81806926056963292, 43.55937500034139731, -42.41743335407647209 ) ) ;
#11107=CARTESIAN_POINT ( 'NONE',  ( -3.210462471511496205E-15, 23.42187500034139802, -52.43083105670540789 ) ) ;
#11117=CARTESIAN_POINT ( 'NONE',  ( -3.210462471511496205E-15, 49.42187500034138736, -52.43083105670540789 ) ) ;
#11121=CARTESIAN_POINT ( 'NONE',  ( 9.657523855033129090E-15, 32.28125000068279604, 52.57311121191334990 ) ) ;
#11122=CARTESIAN_POINT ( 'NONE',  ( 40.34137639590981195, 43.12187500034139731, -29.30972558990011834 ) ) ;
#11132=DIRECTION ( 'NONE',  ( 0.000000000000000000, 1.000000000000000000, 0.000000000000000000 ) ) ;
#11133=CARTESIAN_POINT ( 'NONE',  ( -15.45084971874736368, 24.18125000068279817, 47.55282581475768211 ) ) ;
#11134=CARTESIAN_POINT ( 'NONE',  ( 40.34137639590981195, 37.05937500034139731, -29.30972558990011834 ) ) ;
#11135=CARTESIAN_POINT ( 'NONE',  ( 15.40903463028482356, 42.45937500034140299, 47.42413220539093999 ) ) ;
#11136=CARTESIAN_POINT ( 'NONE',  ( 30.90169943749473802, 25.30000000000000071, -42.53254041760200721 ) ) ;
#11137=( BOUNDED_CURVE ( )  B_SPLINE_CURVE ( 2, ( #5727, #967, #2055, #2130, #15772, #804, #7055, #8372, #16109, #13282, #3221, #5808, #12117 ),
 .UNSPECIFIED., .F., .T. ) 
 B_SPLINE_CURVE_WITH_KNOTS ( ( 3, 2, 2, 2, 2, 2, 3 ),
 ( 0.4166666666666666852, 0.4199999999999999845, 0.4266666666666666941, 0.4333333333333333481, 0.4400000000000000022, 0.4466666666666666563, 0.4500000000000000111 ),
 .UNSPECIFIED. ) 
 CURVE ( )  GEOMETRIC_REPRESENTATION_ITEM ( )  RATIONAL_B_SPLINE_CURVE ( ( 0.9755282581475768211, 0.9755282581475770431, 1.000000000000000000, 0.9510565162951535312, 1.000000000000000000, 0.9510565162951535312, 1.000000000000000000, 0.9510565162951535312, 1.000000000000000000, 0.9510565162951535312, 1.000000000000000000, 0.9755282581475765991, 0.9755282581475768211 ) ) 
 REPRESENTATION_ITEM ( '' )  );
#11141=CARTESIAN_POINT ( 'NONE',  ( -49.40314992384925574, 20.00000000000001776, 8.200154929058633968 ) ) ;
#11142=CARTESIAN_POINT ( 'NONE',  ( 7.919222016226758143, 36.55125428154683931, 50.00000000000000711 ) ) ;
#11151=DIRECTION ( 'NONE',  ( -0.000000000000000000, 1.000000000000000000, -0.000000000000000000 ) ) ;
#11154=DIRECTION ( 'NONE',  ( -0.000000000000000000, -1.000000000000000000, -0.000000000000000000 ) ) ;
#11155=CARTESIAN_POINT ( 'NONE',  ( 17.50000000000000000, 22.50000000000000355, 94.42467108177066848 ) ) ;
#11159=CARTESIAN_POINT ( 'NONE',  ( -49.86468353125000164, 49.89062500034140157, 0.000000000000000000 ) ) ;
#11163=CARTESIAN_POINT ( 'NONE',  ( -50.00000000000000000, 43.78125000068280315, 0.000000000000000000 ) ) ;
#11165=VECTOR ( 'NONE', #5752, 1000.000000000000000 ) ;
#11168=CARTESIAN_POINT ( 'NONE',  ( -7.919222016226816763, 25.55125428154684641, -49.99999999999999289 ) ) ;
#11174=CARTESIAN_POINT ( 'NONE',  ( 30.90169943749473802, 49.29999999999999716, -42.53254041760200721 ) ) ;
#11181=CARTESIAN_POINT ( 'NONE',  ( 15.40903463028482356, 24.52187500034139589, 47.42413220539093999 ) ) ;
#11182=CARTESIAN_POINT ( 'NONE',  ( 49.86468353124999453, 26.95937500034139944, -16.20201782572376104 ) ) ;
#11183=CARTESIAN_POINT ( 'NONE',  ( 30.81806926056964002, 36.62187500034139731, 42.41743335407646498 ) ) ;
#11184=LINE ( 'NONE', #13404, #9733 ) ;
#11185=CARTESIAN_POINT ( 'NONE',  ( -30.81806926056963292, 41.55937500034139731, -42.41743335407647209 ) ) ;
#11188=B_SPLINE_CURVE_WITH_KNOTS ( 'NONE', 3,
 ( #422, #1756, #14546, #11736, #2847, #10587, #15472, #14384, #4093, #1908, #15559, #4268, #4188, #14458, #4430, #578, #9333, #3088, #12990, #9254, #10741, #15800, #5672, #9499, #6688, #1594, #3173, #8074 ),
 .UNSPECIFIED., .F., .F.,
 ( 4, 2, 2, 2, 2, 2, 2, 2, 2, 2, 2, 2, 2, 4 ),
 ( 0.01434078593568147847, 0.01607885267100278917, 0.01781691940632409640, 0.02129305287696671781, 0.02303111961228802851, 0.02476918634760933921, 0.02824531981825197102, 0.02998338655357328519, 0.03172145328889459936, 0.03345952002421591354, 0.03519758675953722771, 0.03867372023017986299, 0.04041178696550118410, 0.04214985370082251215 ),
 .UNSPECIFIED. ) ;
#11189=CARTESIAN_POINT ( 'NONE',  ( -40.45084971874737789, 45.79999999999999716, -29.38926261462365730 ) ) ;
#11190=ADVANCED_FACE ( 'NONE', ( #4526 ), #14637, .F. ) ;
#11191=VERTEX_POINT ( 'NONE', #9344 ) ;
#11196=CARTESIAN_POINT ( 'NONE',  ( 30.90169943749475223, 40.48125000068279888, 42.53254041760199300 ) ) ;
#11197=CARTESIAN_POINT ( 'NONE',  ( 40.34137639590981195, 43.12187500034139731, -29.30972558990011834 ) ) ;
#11201=CARTESIAN_POINT ( 'NONE',  ( 30.90169943749474157, 31.08125000068280031, -42.53254041760200721 ) ) ;
#11203=CARTESIAN_POINT ( 'NONE',  ( -15.40903463028480580, 34.32187500034139305, 47.42413220539094709 ) ) ;
#11215=CARTESIAN_POINT ( 'NONE',  ( -30.81806926056962226, 36.15937500034139163, 42.41743335407647919 ) ) ;
#11216=CARTESIAN_POINT ( 'NONE',  ( -30.81806926056963292, 41.55937500034139731, -42.41743335407646498 ) ) ;
#11222=ORIENTED_EDGE ( 'NONE', *, *, #7912, .F. ) ;
#11228=CARTESIAN_POINT ( 'NONE',  ( -49.99999999999999289, 39.90000000000000568, -16.24598481164531449 ) ) ;
#11230=ORIENTED_EDGE ( 'NONE', *, *, #1165, .F. ) ;
#11232=FACE_OUTER_BOUND ( 'NONE', #14009, .T. ) ;
#11237=CIRCLE ( 'NONE', #13858, 10.00000000000000000 ) ;
#11241=CARTESIAN_POINT ( 'NONE',  ( -49.99999999999999289, 47.88125000068280457, 16.24598481164533226 ) ) ;
#11244=CARTESIAN_POINT ( 'NONE',  ( -3.210462471511496205E-15, 21.35937500034139092, -52.43083105670540789 ) ) ;
#11253=EDGE_CURVE ( 'NONE', #6342, #12450, #1796, .T. ) ;
#11254=CARTESIAN_POINT ( 'NONE',  ( -38.60409515610530917, 20.00000000000000355, 31.77615201968871617 ) ) ;
#11258=CARTESIAN_POINT ( 'NONE',  ( 9.631387414534489405E-15, 22.42187500034139802, 52.43083105670540789 ) ) ;
#11259=CARTESIAN_POINT ( 'NONE',  ( -15.40903463028481646, 29.45937500034139589, -47.42413220539093999 ) ) ;
#11261=CARTESIAN_POINT ( 'NONE',  ( 40.34137639590981195, 33.12187500034139731, -29.30972558990011834 ) ) ;
#11264=CARTESIAN_POINT ( 'NONE',  ( 9.657523855033129090E-15, 40.50000000000000711, 52.57311121191334990 ) ) ;
#11265=CARTESIAN_POINT ( 'NONE',  ( 40.34137639590981905, 38.65937500034139873, 29.30972558990010768 ) ) ;
#11267=CARTESIAN_POINT ( 'NONE',  ( -50.00000000000000000, 48.00000000000000000, 0.000000000000000000 ) ) ;
#11268=VERTEX_POINT ( 'NONE', #7262 ) ;
#11275=CARTESIAN_POINT ( 'NONE',  ( 30.81806926056962936, 43.22187500034140584, -42.41743335407647209 ) ) ;
#11278=CARTESIAN_POINT ( 'NONE',  ( 50.00000000000000711, 24.68125000068279462, 16.24598481164530739 ) ) ;
#11280=CARTESIAN_POINT ( 'NONE',  ( -49.86468353125000164, 33.92187500034139447, 0.000000000000000000 ) ) ;
#11288=AXIS2_PLACEMENT_3D ( 'NONE', #4942, #13969, #3922 ) ;
#11291=CARTESIAN_POINT ( 'NONE',  ( 15.40903463028481113, 31.25937500034140015, -47.42413220539094709 ) ) ;
#11293=CARTESIAN_POINT ( 'NONE',  ( 49.86468353125001585, 48.82187500034139305, 16.20201782572375038 ) ) ;
#11306=CARTESIAN_POINT ( 'NONE',  ( 7.919222016226693306, 34.33250428222964246, 50.00000000000003553 ) ) ;
#11311=CARTESIAN_POINT ( 'NONE',  ( 40.34137639590981195, 49.05937500034139731, -29.30972558990011834 ) ) ;
#11313=CARTESIAN_POINT ( 'NONE',  ( -7.919222016226934890, 32.22999571913595673, 49.99999999999996447 ) ) ;
#11318=DIRECTION ( 'NONE',  ( 0.000000000000000000, 0.000000000000000000, 1.000000000000000000 ) ) ;
#11319=CARTESIAN_POINT ( 'NONE',  ( -15.45084971874736368, 46.18125000068280173, 47.55282581475768211 ) ) ;
#11320=CARTESIAN_POINT ( 'NONE',  ( 49.99999999999999289, 21.09999999999999787, -16.24598481164532160 ) ) ;
#11331=ORIENTED_EDGE ( 'NONE', *, *, #7836, .F. ) ;
#11334=CARTESIAN_POINT ( 'NONE',  ( -3.111920190527341144E-15, 35.28125000068280315, -50.00000000000000000 ) ) ;
#11338=CARTESIAN_POINT ( 'NONE',  ( -15.40903463028480580, 24.32187500034139660, 47.42413220539094709 ) ) ;
#11339=CARTESIAN_POINT ( 'NONE',  ( -3.210462471511496205E-15, 25.35937500034139802, -52.43083105670540789 ) ) ;
#11341=DIRECTION ( 'NONE',  ( 0.000000000000000000, -0.000000000000000000, 1.000000000000000000 ) ) ;
#11342=CARTESIAN_POINT ( 'NONE',  ( 40.34137639590981905, 34.72187500034139873, 29.30972558990010768 ) ) ;
#11345=CARTESIAN_POINT ( 'NONE',  ( -30.90169943749473802, 34.29999999999998295, 42.53254041760200721 ) ) ;
#11346=CARTESIAN_POINT ( 'NONE',  ( -49.86468353125000164, 39.85937500034139447, 0.000000000000000000 ) ) ;
#11348=CARTESIAN_POINT ( 'NONE',  ( 9.657523855033129090E-15, 46.50000000000000711, 52.57311121191334990 ) ) ;
#11356=CARTESIAN_POINT ( 'NONE',  ( -15.45084971874737256, 33.60000000000000142, -47.55282581475767500 ) ) ;
#11359=CARTESIAN_POINT ( 'NONE',  ( -3.210462471511496205E-15, 43.42187500034140157, -52.43083105670540789 ) ) ;
#11362=CARTESIAN_POINT ( 'NONE',  ( 40.45084971874737789, 30.58125000068279675, 29.38926261462365375 ) ) ;
#11364=CARTESIAN_POINT ( 'NONE',  ( -40.34137639590981195, 32.12187500034140442, 29.30972558990012189 ) ) ;
#11372=( BOUNDED_CURVE ( )  B_SPLINE_CURVE ( 2, ( #14168, #10442, #12771, #14006, #16434, #2625, #10199, #1290, #9109, #285, #4123, #11610, #2702 ),
 .UNSPECIFIED., .F., .F. ) 
 B_SPLINE_CURVE_WITH_KNOTS ( ( 3, 2, 2, 2, 2, 2, 3 ),
 ( 0.7166666666666666741, 0.7199999999999999734, 0.7266666666666666829, 0.7333333333333332815, 0.7399999999999999911, 0.7466666666666667007, 0.7500000000000000000 ),
 .UNSPECIFIED. ) 
 CURVE ( )  GEOMETRIC_REPRESENTATION_ITEM ( )  RATIONAL_B_SPLINE_CURVE ( ( 0.9755282581475768211, 0.9755282581475768211, 1.000000000000000000, 0.9510565162951535312, 1.000000000000000000, 0.9510565162951535312, 1.000000000000000000, 0.9510565162951535312, 1.000000000000000000, 0.9510565162951535312, 1.000000000000000000, 0.9755282581475768211, 0.9755282581475768211 ) ) 
 REPRESENTATION_ITEM ( '' )  );
#11377=CARTESIAN_POINT ( 'NONE',  ( 15.40903463028482356, 32.45937500034138878, 47.42413220539093999 ) ) ;
#11378=CARTESIAN_POINT ( 'NONE',  ( -3.210462471511496205E-15, 43.42187500034140157, -52.43083105670540789 ) ) ;
#11394=CARTESIAN_POINT ( 'NONE',  ( 30.90169943749473802, 33.08125000068279320, -42.53254041760200721 ) ) ;
#11398=CARTESIAN_POINT ( 'NONE',  ( -15.45084971874737256, 49.60000000000000853, -47.55282581475767500 ) ) ;
#11399=CARTESIAN_POINT ( 'NONE',  ( 49.99999999999999289, 44.88125000068279036, -16.24598481164532160 ) ) ;
#11400=CARTESIAN_POINT ( 'NONE',  ( 50.00000000000000000, 44.78125000068280315, -6.123233995736766085E-15 ) ) ;
#11401=ADVANCED_FACE ( 'NONE', ( #2006 ), #7103, .F. ) ;
#11403=CARTESIAN_POINT ( 'NONE',  ( -49.86468353124999453, 21.95937500034138878, 16.20201782572377525 ) ) ;
#11419=CARTESIAN_POINT ( 'NONE',  ( 49.86468353125001585, 24.75937500034139660, 16.20201782572375038 ) ) ;
#11421=CARTESIAN_POINT ( 'NONE',  ( 15.40903463028482356, 38.52187500034139589, 47.42413220539093999 ) ) ;
#11423=CARTESIAN_POINT ( 'NONE',  ( -49.99999999999999289, 29.89999999999999858, -16.24598481164531449 ) ) ;
#11424=CARTESIAN_POINT ( 'NONE',  ( -30.81806926056963292, 37.55937500034139020, -42.41743335407647209 ) ) ;
#11426=CARTESIAN_POINT ( 'NONE',  ( -30.90169943749474868, 47.70000000000000995, -42.53254041760200721 ) ) ;
#11438=CARTESIAN_POINT ( 'NONE',  ( 49.86468353124999453, 45.02187500034138878, -16.20201782572376459 ) ) ;
#11441=CARTESIAN_POINT ( 'NONE',  ( 40.45084971874737789, 26.58125000068279675, 29.38926261462365375 ) ) ;
#11442=CARTESIAN_POINT ( 'NONE',  ( 17.50000000000000000, 22.50000000000000355, 94.42467108177066848 ) ) ;
#11443=CARTESIAN_POINT ( 'NONE',  ( -49.86468353124999453, 33.82187500034138594, -16.20201782572375393 ) ) ;
#11445=DIRECTION ( 'NONE',  ( 0.000000000000000000, -0.000000000000000000, 1.000000000000000000 ) ) ;
#11450=CARTESIAN_POINT ( 'NONE',  ( -49.99999999999999289, 23.90000000000000213, -16.24598481164531449 ) ) ;
#11452=CARTESIAN_POINT ( 'NONE',  ( 40.34137639590981195, 31.05937500034139731, -29.30972558990011834 ) ) ;
#11453=CARTESIAN_POINT ( 'NONE',  ( 9.631387414534489405E-15, 46.42187500034139447, 52.43083105670540789 ) ) ;
#11454=CYLINDRICAL_SURFACE ( 'NONE', #2213, 10.00000000000000000 ) ;
#11460=CARTESIAN_POINT ( 'NONE',  ( -49.99999999999999289, 45.88125000068279746, 16.24598481164533226 ) ) ;
#11464=CARTESIAN_POINT ( 'NONE',  ( 30.90169943749475223, 34.48125000068279888, 42.53254041760199300 ) ) ;
#11465=CARTESIAN_POINT ( 'NONE',  ( 1.293669679204937499E-13, 39.28125000068280315, -50.00000000000000000 ) ) ;
#11467=CARTESIAN_POINT ( 'NONE',  ( 50.00000000000000000, 32.78125000068279604, -6.123233995736766085E-15 ) ) ;
#11470=CARTESIAN_POINT ( 'NONE',  ( 49.99999999999999289, 24.88125000068279746, -16.24598481164532160 ) ) ;
#11472=CARTESIAN_POINT ( 'NONE',  ( -40.45084971874737789, 49.80000000000000426, -29.38926261462365730 ) ) ;
#11473=CARTESIAN_POINT ( 'NONE',  ( -15.45084971874737256, 41.38125000068279746, -47.55282581475767500 ) ) ;
#11474=CARTESIAN_POINT ( 'NONE',  ( -3.111920190527341144E-15, 45.28125000068279604, -50.00000000000000000 ) ) ;
#11475=CARTESIAN_POINT ( 'NONE',  ( 40.45084971874737079, 46.98125000068280599, -29.38926261462366440 ) ) ;
#11480=FACE_OUTER_BOUND ( 'NONE', #817, .T. ) ;
#11487=DIRECTION ( 'NONE',  ( -0.000000000000000000, 1.000000000000000000, -0.000000000000000000 ) ) ;
#11491=CARTESIAN_POINT ( 'NONE',  ( 40.34137639590981905, 24.65937500034139873, 29.30972558990010768 ) ) ;
#11493=CARTESIAN_POINT ( 'NONE',  ( -40.34137639590981195, 26.12187500034139731, 29.30972558990012189 ) ) ;
#11494=ADVANCED_FACE ( 'NONE', ( #5184 ), #6423, .F. ) ;
#11497=CARTESIAN_POINT ( 'NONE',  ( -3.219174618344376363E-15, 33.50000000000000711, -52.57311121191334990 ) ) ;
#11498=CARTESIAN_POINT ( 'NONE',  ( -40.34137639590981195, 36.05937500034139731, 29.30972558990012189 ) ) ;
#11500=CARTESIAN_POINT ( 'NONE',  ( 40.45084971874737079, 41.20000000000000284, -29.38926261462366440 ) ) ;
#11505=EDGE_LOOP ( 'NONE', ( #5554, #8390, #5591, #5985 ) ) ;
#11510=VECTOR ( 'NONE', #13714, 1000.000000000000000 ) ;
#11512=CARTESIAN_POINT ( 'NONE',  ( 49.86468353125000164, 44.92187500034140157, -6.106662507704105588E-15 ) ) ;
#11513=CARTESIAN_POINT ( 'NONE',  ( -30.81806926056963292, 43.55937500034139731, -42.41743335407646498 ) ) ;
#11516=CARTESIAN_POINT ( 'NONE',  ( 9.657523855033129090E-15, 28.28125000068279249, 52.57311121191334990 ) ) ;
#11517=CARTESIAN_POINT ( 'NONE',  ( -40.45084971874737789, 35.58125000068279320, -29.38926261462365730 ) ) ;
#11518=CARTESIAN_POINT ( 'NONE',  ( -15.40903463028481646, 33.52187500034140299, -47.42413220539093999 ) ) ;
#11520=ORIENTED_EDGE ( 'NONE', *, *, #159, .T. ) ;
#11526=CARTESIAN_POINT ( 'NONE',  ( -49.86468353124999453, 31.75937500034140015, -16.20201782572375393 ) ) ;
#11529=CARTESIAN_POINT ( 'NONE',  ( -30.81806926056962226, 48.22187500034139163, 42.41743335407647209 ) ) ;
#11531=CARTESIAN_POINT ( 'NONE',  ( 0.000000000000000000, 20.00000000000000355, 0.000000000000000000 ) ) ;
#11539=ORIENTED_EDGE ( 'NONE', *, *, #14467, .F. ) ;
#11544=CARTESIAN_POINT ( 'NONE',  ( -30.81806926056962226, 48.15937500034139873, 42.41743335407647919 ) ) ;
#11550=CARTESIAN_POINT ( 'NONE',  ( 30.90169943749475578, 38.48125000068279178, 42.53254041760200010 ) ) ;
#11556=( BOUNDED_CURVE ( )  B_SPLINE_CURVE ( 2, ( #14416, #14498, #15505, #10777, #4131, #6804, #9206, #5561, #8108, #5709, #15843, #2883, #369 ),
 .UNSPECIFIED., .F., .T. ) 
 B_SPLINE_CURVE_WITH_KNOTS ( ( 3, 2, 2, 2, 2, 2, 3 ),
 ( 0.6166666666666666963, 0.6199999999999999956, 0.6266666666666667052, 0.6333333333333333037, 0.6400000000000000133, 0.6466666666666666119, 0.6500000000000000222 ),
 .UNSPECIFIED. ) 
 CURVE ( )  GEOMETRIC_REPRESENTATION_ITEM ( )  RATIONAL_B_SPLINE_CURVE ( ( 0.9755282581475768211, 0.9755282581475771542, 1.000000000000000000, 0.9510565162951535312, 1.000000000000000000, 0.9510565162951535312, 1.000000000000000000, 0.9510565162951535312, 1.000000000000000000, 0.9510565162951535312, 1.000000000000000000, 0.9755282581475763770, 0.9755282581475768211 ) ) 
 REPRESENTATION_ITEM ( '' )  );
#11565=CARTESIAN_POINT ( 'NONE',  ( 15.45084971874737789, 32.60000000000000142, 47.55282581475767500 ) ) ;
#11572=CARTESIAN_POINT ( 'NONE',  ( 9.631387414534489405E-15, 24.35937500034139447, 52.43083105670540789 ) ) ;
#11574=CARTESIAN_POINT ( 'NONE',  ( -49.86468353125000164, 29.92187500034139802, 0.000000000000000000 ) ) ;
#11577=CARTESIAN_POINT ( 'NONE',  ( 40.45084971874737079, 33.20000000000000284, -29.38926261462366440 ) ) ;
#11578=CARTESIAN_POINT ( 'NONE',  ( 15.40903463028481113, 33.25937500034140015, -47.42413220539094709 ) ) ;
#11583=AXIS2_PLACEMENT_3D ( 'NONE', #15508, #14265, #2887 ) ;
#11587=ORIENTED_EDGE ( 'NONE', *, *, #14133, .T. ) ;
#11588=VERTEX_POINT ( 'NONE', #170 ) ;
#11593=DIRECTION ( 'NONE',  ( -0.000000000000000000, 1.000000000000000000, -0.000000000000000000 ) ) ;
#11595=VECTOR ( 'NONE', #13210, 1000.000000000000000 ) ;
#11599=CARTESIAN_POINT ( 'NONE',  ( 9.631387414534489405E-15, 38.42187500034139447, 52.43083105670540789 ) ) ;
#11600=CARTESIAN_POINT ( 'NONE',  ( 30.81806926056964002, 44.55937500034139020, 42.41743335407646498 ) ) ;
#11601=LINE ( 'NONE', #32, #15311 ) ;
#11603=CARTESIAN_POINT ( 'NONE',  ( 15.45084971874737789, 20.38125000068279746, 47.55282581475767500 ) ) ;
#11606=CARTESIAN_POINT ( 'NONE',  ( -3.210462471511496205E-15, 27.42187500034139092, -52.43083105670540789 ) ) ;
#11609=CIRCLE ( 'NONE', #6860, 17.50000000000000000 ) ;
#11610=CARTESIAN_POINT ( 'NONE',  ( -7.919222016226816763, 27.55125428154684641, -49.99999999999999289 ) ) ;
#11614=CARTESIAN_POINT ( 'NONE',  ( 15.45084971874737789, 48.38125000068280457, 47.55282581475767500 ) ) ;
#11618=CARTESIAN_POINT ( 'NONE',  ( 49.86468353124999453, 30.95937500034139944, -16.20201782572376459 ) ) ;
#11621=CARTESIAN_POINT ( 'NONE',  ( -40.34137639590981195, 46.12187500034139731, 29.30972558990012189 ) ) ;
#11625=CARTESIAN_POINT ( 'NONE',  ( -40.34137639590981195, 48.12187500034139731, 29.30972558990012189 ) ) ;
#11630=VERTEX_POINT ( 'NONE', #12568 ) ;
#11637=DIRECTION ( 'NONE',  ( -0.000000000000000000, 1.000000000000000000, -0.000000000000000000 ) ) ;
#11638=CARTESIAN_POINT ( 'NONE',  ( -49.99999999999999289, 21.90000000000000568, -16.24598481164531449 ) ) ;
#11640=CARTESIAN_POINT ( 'NONE',  ( -7.919222016226816763, 25.33250428222964246, -49.99999999999999289 ) ) ;
#11642=CARTESIAN_POINT ( 'NONE',  ( -49.86468353124999453, 22.02187500034139589, 16.20201782572377525 ) ) ;
#11645=CARTESIAN_POINT ( 'NONE',  ( 49.99999999999999289, 38.88125000068279036, -16.24598481164532160 ) ) ;
#11646=CARTESIAN_POINT ( 'NONE',  ( -2.445080149700054274E-14, 46.50000000000000711, 50.00000000000000000 ) ) ;
#11660=CARTESIAN_POINT ( 'NONE',  ( 30.81806926056962936, 21.15937500034139518, -42.41743335407646498 ) ) ;
#11661=CARTESIAN_POINT ( 'NONE',  ( -47.39803307437431101, 19.99999999999999645, 15.49002591438328302 ) ) ;
#11662=CARTESIAN_POINT ( 'NONE',  ( 49.86468353124999453, 29.02187500034139234, -16.20201782572376104 ) ) ;
#11663=( BOUNDED_CURVE ( )  B_SPLINE_CURVE ( 2, ( #975, #15948, #7395, #6074, #8303, #16200, #13369, #13694, #1055, #16027, #14685, #8469, #14939 ),
 .UNSPECIFIED., .F., .T. ) 
 B_SPLINE_CURVE_WITH_KNOTS ( ( 3, 2, 2, 2, 2, 2, 3 ),
 ( 0.2833333333333333814, 0.2866666666666666807, 0.2933333333333333348, 0.2999999999999999889, 0.3066666666666666430, 0.3133333333333333526, 0.3166666666666667074 ),
 .UNSPECIFIED. ) 
 CURVE ( )  GEOMETRIC_REPRESENTATION_ITEM ( )  RATIONAL_B_SPLINE_CURVE ( ( 0.9755282581475768211, 0.9755282581475770431, 1.000000000000000000, 0.9510565162951535312, 1.000000000000000000, 0.9510565162951535312, 1.000000000000000000, 0.9510565162951535312, 1.000000000000000000, 0.9510565162951535312, 1.000000000000000000, 0.9755282581475765991, 0.9755282581475768211 ) ) 
 REPRESENTATION_ITEM ( '' )  );
#11665=CARTESIAN_POINT ( 'NONE',  ( -30.90169943749474868, 33.69999999999998863, -42.53254041760200721 ) ) ;
#11666=CARTESIAN_POINT ( 'NONE',  ( 49.86468353125000164, 34.85937500034140157, -6.106662507704105588E-15 ) ) ;
#11668=VERTEX_POINT ( 'NONE', #10325 ) ;
#11670=ORIENTED_EDGE ( 'NONE', *, *, #7141, .T. ) ;
#11677=CARTESIAN_POINT ( 'NONE',  ( -49.86468353124999453, 34.02187500034140299, 16.20201782572377525 ) ) ;
#11678=CARTESIAN_POINT ( 'NONE',  ( -30.81806926056962226, 44.15937500034139163, 42.41743335407647209 ) ) ;
#11681=CARTESIAN_POINT ( 'NONE',  ( 50.00000000000000000, 20.78125000068279959, -6.123233995736766085E-15 ) ) ;
#11683=CARTESIAN_POINT ( 'NONE',  ( -7.919222016226816763, 35.33250428222964246, -49.99999999999999289 ) ) ;
#11684=CARTESIAN_POINT ( 'NONE',  ( 49.86468353124999453, 27.02187500034139589, -16.20201782572376459 ) ) ;
#11689=CARTESIAN_POINT ( 'NONE',  ( -38.60409515610530917, 20.00000000000000355, 31.77615201968871617 ) ) ;
#11692=CARTESIAN_POINT ( 'NONE',  ( -3.111920190527341144E-15, 29.28125000068279604, -50.00000000000000000 ) ) ;
#11694=CARTESIAN_POINT ( 'NONE',  ( 9.631387414534489405E-15, 22.35937500034139802, 52.43083105670540789 ) ) ;
#11696=CARTESIAN_POINT ( 'NONE',  ( 9.631387414534489405E-15, 42.42187500034140157, 52.43083105670540789 ) ) ;
#11700=CARTESIAN_POINT ( 'NONE',  ( -15.40903463028481646, 47.52187500034139589, -47.42413220539093999 ) ) ;
#11705=ORIENTED_EDGE ( 'NONE', *, *, #8894, .F. ) ;
#11708=ORIENTED_EDGE ( 'NONE', *, *, #2037, .F. ) ;
#11711=CARTESIAN_POINT ( 'NONE',  ( -1.240322475938754499E-13, 38.28125000068280315, 50.00000000000000000 ) ) ;
#11712=CARTESIAN_POINT ( 'NONE',  ( -50.00000000000000000, 24.00000000000000000, 0.000000000000000000 ) ) ;
#11713=CARTESIAN_POINT ( 'NONE',  ( 9.631387414534489405E-15, 42.35937500034140157, 52.43083105670540789 ) ) ;
#11714=CARTESIAN_POINT ( 'NONE',  ( -49.99999999999999289, 25.88125000068279746, 16.24598481164533226 ) ) ;
#11715=DIRECTION ( 'NONE',  ( -0.000000000000000000, 1.000000000000000000, -0.000000000000000000 ) ) ;
#11716=CARTESIAN_POINT ( 'NONE',  ( -40.34137639590981195, 26.12187500034139731, 29.30972558990012189 ) ) ;
#11718=DIRECTION ( 'NONE',  ( 0.000000000000000000, 1.000000000000000000, 0.000000000000000000 ) ) ;
#11719=CARTESIAN_POINT ( 'NONE',  ( 15.45084971874737789, 42.38125000068279746, 47.55282581475767500 ) ) ;
#11721=CARTESIAN_POINT ( 'NONE',  ( 7.919222016226693306, 20.33250428222963890, 50.00000000000003553 ) ) ;
#11722=ADVANCED_FACE ( 'NONE', ( #3164 ), #9155, .F. ) ;
#11723=ORIENTED_EDGE ( 'NONE', *, *, #15738, .T. ) ;
#11728=CARTESIAN_POINT ( 'NONE',  ( 0.000000000000000000, 20.00000000000000355, 0.000000000000000000 ) ) ;
#11736=CARTESIAN_POINT ( 'NONE',  ( 2.313956153764268553, 5.143932793412055560, 99.06765316570249524 ) ) ;
#11738=CARTESIAN_POINT ( 'NONE',  ( 30.81806926056964002, 26.62187500034139731, 42.41743335407646498 ) ) ;
#11741=CARTESIAN_POINT ( 'NONE',  ( -49.86468353125000164, 31.85937500034139447, 0.000000000000000000 ) ) ;
#11749=DIRECTION ( 'NONE',  ( 0.000000000000000000, 0.000000000000000000, 1.000000000000000000 ) ) ;
#11754=CARTESIAN_POINT ( 'NONE',  ( 15.40903463028481113, 33.32187500034139305, -47.42413220539094709 ) ) ;
#11755=CARTESIAN_POINT ( 'NONE',  ( 40.34137639590981905, 36.65937500034139873, 29.30972558990010768 ) ) ;
#11760=CARTESIAN_POINT ( 'NONE',  ( 49.86468353124999453, 48.95937500034140299, -16.20201782572376459 ) ) ;
#11762=CARTESIAN_POINT ( 'NONE',  ( 49.86468353125001585, 26.82187500034138949, 16.20201782572375038 ) ) ;
#11767=CARTESIAN_POINT ( 'NONE',  ( 40.45084971874737079, 48.98125000068279888, -29.38926261462366440 ) ) ;
#11771=CARTESIAN_POINT ( 'NONE',  ( -49.86468353125000164, 23.85937500034139447, 0.000000000000000000 ) ) ;
#11772=CARTESIAN_POINT ( 'NONE',  ( 30.81806926056964002, 42.62187500034139731, 42.41743335407646498 ) ) ;
#11775=AXIS2_PLACEMENT_3D ( 'NONE', #990, #13382, #4510 ) ;
#11776=CARTESIAN_POINT ( 'NONE',  ( -40.34137639590981905, 49.72187500034139873, -29.30972558990011478 ) ) ;
#11783=ORIENTED_EDGE ( 'NONE', *, *, #8705, .F. ) ;
#11785=CARTESIAN_POINT ( 'NONE',  ( 6.123233995736766085E-15, 20.00000000000000355, -50.00000000000000000 ) ) ;
#11786=DIRECTION ( 'NONE',  ( -0.000000000000000000, 1.000000000000000000, -0.000000000000000000 ) ) ;
#11789=DIRECTION ( 'NONE',  ( 0.000000000000000000, -0.9848077530122080203, 0.1736481776669307198 ) ) ;
#11790=CARTESIAN_POINT ( 'NONE',  ( -49.99999999999999289, 23.90000000000000213, -16.24598481164531449 ) ) ;
#11791=CARTESIAN_POINT ( 'NONE',  ( 40.34137639590981195, 45.05937500034139731, -29.30972558990011834 ) ) ;
#11797=CARTESIAN_POINT ( 'NONE',  ( 15.45084971874737789, 40.38125000068280457, 47.55282581475767500 ) ) ;
#11798=( BOUNDED_CURVE ( )  B_SPLINE_CURVE ( 2, ( #8823, #13886, #2501, #7581, #7746, #7668, #12738, #6426, #14056, #2672, #11565, #12814, #1416 ),
 .UNSPECIFIED., .F., .F. ) 
 B_SPLINE_CURVE_WITH_KNOTS ( ( 3, 2, 2, 2, 2, 2, 3 ),
 ( 0.5500000000000000444, 0.5533333333333333437, 0.5600000000000000533, 0.5666666666666666519, 0.5733333333333333615, 0.5799999999999999600, 0.5833333333333333703 ),
 .UNSPECIFIED. ) 
 CURVE ( )  GEOMETRIC_REPRESENTATION_ITEM ( )  RATIONAL_B_SPLINE_CURVE ( ( 0.9755282581475768211, 0.9755282581475771542, 1.000000000000000000, 0.9510565162951535312, 1.000000000000000000, 0.9510565162951535312, 1.000000000000000000, 0.9510565162951535312, 1.000000000000000000, 0.9510565162951535312, 1.000000000000000000, 0.9755282581475763770, 0.9755282581475768211 ) ) 
 REPRESENTATION_ITEM ( '' )  );
#11800=DIRECTION ( 'NONE',  ( 1.003171929053523391E-16, -0.5735764363510476027, 0.8191520442889907994 ) ) ;
#11801=ORIENTED_EDGE ( 'NONE', *, *, #9141, .T. ) ;
#11815=CARTESIAN_POINT ( 'NONE',  ( -7.919222016226934890, 30.22999571913595318, 49.99999999999996447 ) ) ;
#11816=CARTESIAN_POINT ( 'NONE',  ( -43.10890719796073256, 20.03031439394993996, 25.50054622961014772 ) ) ;
#11817=CARTESIAN_POINT ( 'NONE',  ( -48.28553921371794644, 20.00000000000000355, 12.45074877219254894 ) ) ;
#11818=CARTESIAN_POINT ( 'NONE',  ( -15.40903463028480580, 28.32187500034139660, 47.42413220539094709 ) ) ;
#11821=CARTESIAN_POINT ( 'NONE',  ( -30.81806926056962226, 30.15937500034139163, 42.41743335407647919 ) ) ;
#11833=CARTESIAN_POINT ( 'NONE',  ( 49.86468353124999453, 35.02187500034139589, -16.20201782572376459 ) ) ;
#11834=CARTESIAN_POINT ( 'NONE',  ( 49.86468353125001585, 36.75937500034139305, 16.20201782572375038 ) ) ;
#11841=CARTESIAN_POINT ( 'NONE',  ( -49.99999999999999289, 19.88125000068279746, 16.24598481164533226 ) ) ;
#11845=CARTESIAN_POINT ( 'NONE',  ( 30.81806926056962936, 27.22187500034139518, -42.41743335407647209 ) ) ;
#11847=CARTESIAN_POINT ( 'NONE',  ( -15.45084971874737256, 27.38125000068280102, -47.55282581475767500 ) ) ;
#11848=VECTOR ( 'NONE', #4059, 1000.000000000000000 ) ;
#11850=VECTOR ( 'NONE', #10247, 1000.000000000000000 ) ;
#11856=CARTESIAN_POINT ( 'NONE',  ( -2.547328955960238000E-13, 34.28125000068279604, 49.99999999999999289 ) ) ;
#11858=CARTESIAN_POINT ( 'NONE',  ( 49.86468353125000164, 26.85937500034139802, -6.106662507704105588E-15 ) ) ;
#11860=CARTESIAN_POINT ( 'NONE',  ( 40.34137639590981905, 38.72187500034139873, 29.30972558990010768 ) ) ;
#11865=CARTESIAN_POINT ( 'NONE',  ( 30.81806926056964002, 48.62187500034139731, 42.41743335407647209 ) ) ;
#11870=EDGE_CURVE ( 'NONE', #6639, #13132, #5516, .T. ) ;
#11877=CARTESIAN_POINT ( 'NONE',  ( 15.45084971874736723, 23.40000000000000213, -47.55282581475768211 ) ) ;
#11878=CARTESIAN_POINT ( 'NONE',  ( 15.40903463028482356, 44.45937500034139589, 47.42413220539093999 ) ) ;
#11879=CARTESIAN_POINT ( 'NONE',  ( -15.45084971874737256, 31.38125000068280102, -47.55282581475767500 ) ) ;
#11883=CARTESIAN_POINT ( 'NONE',  ( 30.90169943749475578, 32.48125000068280599, 42.53254041760200010 ) ) ;
#11885=CARTESIAN_POINT ( 'NONE',  ( 15.45084971874736723, 23.18125000068279817, -47.55282581475768211 ) ) ;
#11887=EDGE_CURVE ( 'NONE', #3182, #10580, #13706, .T. ) ;
#11888=PRODUCT_DEFINITION ( 'UNKNOWN', '', #8385, #7925 ) ;
#11906=CARTESIAN_POINT ( 'NONE',  ( -47.34572995173778764, 19.99999999999999645, 15.64827527265654616 ) ) ;
#11907=CARTESIAN_POINT ( 'NONE',  ( 15.40903463028482356, 24.52187500034139589, 47.42413220539093999 ) ) ;
#11910=CARTESIAN_POINT ( 'NONE',  ( -3.210462471511496205E-15, 29.35937500034139802, -52.43083105670540789 ) ) ;
#11922=CARTESIAN_POINT ( 'NONE',  ( 49.86468353124999453, 39.02187500034138878, -16.20201782572376459 ) ) ;
#11923=CARTESIAN_POINT ( 'NONE',  ( -40.34137639590981905, 37.65937500034139873, -29.30972558990011478 ) ) ;
#11926=CARTESIAN_POINT ( 'NONE',  ( 40.45084971874737079, 22.98125000068279888, -29.38926261462366440 ) ) ;
#11928=CARTESIAN_POINT ( 'NONE',  ( -30.81806926056963292, 27.62187500034139731, -42.41743335407647209 ) ) ;
#11938=CARTESIAN_POINT ( 'NONE',  ( -15.40903463028480580, 26.25937500034140015, 47.42413220539094709 ) ) ;
#11940=CARTESIAN_POINT ( 'NONE',  ( -30.81806926056962226, 42.22187500034139163, 42.41743335407647209 ) ) ;
#11943=EDGE_CURVE ( 'NONE', #15320, #4733, #10307, .T. ) ;
#11944=CARTESIAN_POINT ( 'NONE',  ( -3.210462471511496205E-15, 47.42187500034138736, -52.43083105670540789 ) ) ;
#11947=EDGE_LOOP ( 'NONE', ( #12607, #2588, #9173, #1559 ) ) ;
#11951=ADVANCED_FACE ( 'NONE', ( #898 ), #16132, .F. ) ;
#11952=DIRECTION ( 'NONE',  ( 0.000000000000000000, 0.000000000000000000, 1.000000000000000000 ) ) ;
#11953=CARTESIAN_POINT ( 'NONE',  ( 15.45084971874737789, 38.38125000068279746, 47.55282581475767500 ) ) ;
#11955=CARTESIAN_POINT ( 'NONE',  ( 9.657523855033129090E-15, 22.50000000000000355, 52.57311121191334990 ) ) ;
#11956=CARTESIAN_POINT ( 'NONE',  ( 15.40903463028482356, 42.45937500034140299, 47.42413220539093999 ) ) ;
#11957=CARTESIAN_POINT ( 'NONE',  ( -40.34137639590981905, 47.65937500034139873, -29.30972558990011478 ) ) ;
#11962=CARTESIAN_POINT ( 'NONE',  ( 15.45084971874737789, 32.38125000068280457, 47.55282581475767500 ) ) ;
#11964=CARTESIAN_POINT ( 'NONE',  ( 15.45084971874736723, 37.40000000000000568, -47.55282581475768211 ) ) ;
#11971=CYLINDRICAL_SURFACE ( 'NONE', #9693, 50.00000000000000000 ) ;
#11980=CARTESIAN_POINT ( 'NONE',  ( -7.919222016226816763, 29.33250428222964601, -49.99999999999999289 ) ) ;
#11981=DIRECTION ( 'NONE',  ( 0.000000000000000000, 0.000000000000000000, -1.000000000000000000 ) ) ;
#11982=CARTESIAN_POINT ( 'NONE',  ( -48.35726954556750457, 20.00000000000000355, 12.16803787670978387 ) ) ;
#11983=CARTESIAN_POINT ( 'NONE',  ( 30.81806926056964002, 24.62187500034139731, 42.41743335407646498 ) ) ;
#11986=CARTESIAN_POINT ( 'NONE',  ( -3.210462471511496205E-15, 25.35937500034139802, -52.43083105670540789 ) ) ;
#11989=ADVANCED_FACE ( 'NONE', ( #3495 ), #8550, .F. ) ;
#11993=( BOUNDED_CURVE ( )  B_SPLINE_CURVE ( 2, ( #15364, #2399, #12790, #12545, #3905, #9055, #7647, #3821, #10139, #11464, #6235, #11306, #12875 ),
 .UNSPECIFIED., .F., .F. ) 
 B_SPLINE_CURVE_WITH_KNOTS ( ( 3, 2, 2, 2, 2, 2, 3 ),
 ( 0.4833333333333333370, 0.4866666666666666918, 0.4933333333333333459, 0.5000000000000000000, 0.5066666666666667096, 0.5133333333333333082, 0.5166666666666667185 ),
 .UNSPECIFIED. ) 
 CURVE ( )  GEOMETRIC_REPRESENTATION_ITEM ( )  RATIONAL_B_SPLINE_CURVE ( ( 0.9755282581475768211, 0.9755282581475768211, 1.000000000000000000, 0.9510565162951535312, 1.000000000000000000, 0.9510565162951535312, 1.000000000000000000, 0.9510565162951535312, 1.000000000000000000, 0.9510565162951535312, 1.000000000000000000, 0.9755282581475763770, 0.9755282581475768211 ) ) 
 REPRESENTATION_ITEM ( '' )  );
#11999=CARTESIAN_POINT ( 'NONE',  ( 30.81806926056964002, 30.62187500034139020, 42.41743335407647209 ) ) ;
#12000=CARTESIAN_POINT ( 'NONE',  ( 49.86468353125001585, 34.75937500034138594, 16.20201782572375038 ) ) ;
#12005=CARTESIAN_POINT ( 'NONE',  ( 40.34137639590981195, 47.05937500034140442, -29.30972558990011834 ) ) ;
#12007=CARTESIAN_POINT ( 'NONE',  ( 49.99999999999999289, 49.10000000000000853, -16.24598481164532160 ) ) ;
#12012=VERTEX_POINT ( 'NONE', #15192 ) ;
#12014=CARTESIAN_POINT ( 'NONE',  ( -49.99999999999999289, 33.88125000068280457, 16.24598481164533226 ) ) ;
#12016=CARTESIAN_POINT ( 'NONE',  ( -40.34137639590981905, 23.65937500034139518, -29.30972558990011478 ) ) ;
#12019=CARTESIAN_POINT ( 'NONE',  ( 15.45084971874737789, 34.60000000000000853, 47.55282581475767500 ) ) ;
#12020=CARTESIAN_POINT ( 'NONE',  ( 30.81806926056964002, 42.62187500034139731, 42.41743335407647209 ) ) ;
#12021=CARTESIAN_POINT ( 'NONE',  ( 30.90169943749473802, 31.30000000000000071, -42.53254041760200721 ) ) ;
#12025=VERTEX_POINT ( 'NONE', #1313 ) ;
#12030=CARTESIAN_POINT ( 'NONE',  ( 50.00000000000000711, 20.90000000000000213, 16.24598481164530739 ) ) ;
#12031=CARTESIAN_POINT ( 'NONE',  ( -49.86468353124999453, 43.75937500034140015, -16.20201782572375393 ) ) ;
#12032=CARTESIAN_POINT ( 'NONE',  ( 30.81806926056964002, 48.55937500034139020, 42.41743335407646498 ) ) ;
#12033=CARTESIAN_POINT ( 'NONE',  ( 50.00000000000000000, 25.00000000000000000, -6.123233995736766085E-15 ) ) ;
#12037=CARTESIAN_POINT ( 'NONE',  ( -7.919222016226870942, 36.22999571913594963, 49.99999999999997158 ) ) ;
#12038=CARTESIAN_POINT ( 'NONE',  ( -2.547328955960238000E-13, 22.28125000068279604, 49.99999999999999289 ) ) ;
#12047=CIRCLE ( 'NONE', #4906, 92.05189185291139609 ) ;
#12056=CARTESIAN_POINT ( 'NONE',  ( -7.919222016226802552, 47.55125428154684641, -50.00000000000000000 ) ) ;
#12058=CARTESIAN_POINT ( 'NONE',  ( 2.978552182361884590E-14, 47.50000000000000711, -50.00000000000000000 ) ) ;
#12060=CARTESIAN_POINT ( 'NONE',  ( 49.86468353125001585, 24.82187500034139305, 16.20201782572375038 ) ) ;
#12062=AXIS2_PLACEMENT_3D ( 'NONE', #14157, #352, #5452 ) ;
#12064=CARTESIAN_POINT ( 'NONE',  ( 9.631387414534489405E-15, 28.35937500034139802, 52.43083105670540789 ) ) ;
#12066=ORIENTED_EDGE ( 'NONE', *, *, #14017, .F. ) ;
#12069=ORIENTED_EDGE ( 'NONE', *, *, #16361, .F. ) ;
#12074=CARTESIAN_POINT ( 'NONE',  ( 49.86468353125000164, 26.92187500034139802, -6.106662507704105588E-15 ) ) ;
#12075=CARTESIAN_POINT ( 'NONE',  ( 49.86468353124999453, 34.95937500034138878, -16.20201782572376104 ) ) ;
#12080=CARTESIAN_POINT ( 'NONE',  ( 9.631387414534489405E-15, 42.35937500034140157, 52.43083105670540789 ) ) ;
#12083=CARTESIAN_POINT ( 'NONE',  ( 49.86468353125000164, 22.92187500034139802, -6.106662507704105588E-15 ) ) ;
#12086=( BOUNDED_CURVE ( )  B_SPLINE_CURVE ( 2, ( #1462, #2631, #2461, #3964, #10045, #1377, #15426, #11450, #122, #5148, #10205, #9039, #9116 ),
 .UNSPECIFIED., .F., .F. ) 
 B_SPLINE_CURVE_WITH_KNOTS ( ( 3, 2, 2, 2, 2, 2, 3 ),
 ( 0.8500000000000000888, 0.8533333333333333881, 0.8599999999999999867, 0.8666666666666666963, 0.8733333333333332948, 0.8800000000000000044, 0.8833333333333334147 ),
 .UNSPECIFIED. ) 
 CURVE ( )  GEOMETRIC_REPRESENTATION_ITEM ( )  RATIONAL_B_SPLINE_CURVE ( ( 0.9755282581475768211, 0.9755282581475771542, 1.000000000000000000, 0.9510565162951535312, 1.000000000000000000, 0.9510565162951535312, 1.000000000000000000, 0.9510565162951535312, 1.000000000000000000, 0.9510565162951535312, 1.000000000000000000, 0.9755282581475763770, 0.9755282581475768211 ) ) 
 REPRESENTATION_ITEM ( '' )  );
#12090=ORIENTED_EDGE ( 'NONE', *, *, #2216, .T. ) ;
#12093=EDGE_CURVE ( 'NONE', #12984, #7369, #11993, .T. ) ;
#12097=CARTESIAN_POINT ( 'NONE',  ( 15.40903463028481113, 47.32187500034140015, -47.42413220539094709 ) ) ;
#12102=CARTESIAN_POINT ( 'NONE',  ( 30.90169943749475578, 40.69999999999999574, 42.53254041760200010 ) ) ;
#12103=CARTESIAN_POINT ( 'NONE',  ( -40.34137639590981905, 43.72187500034139873, -29.30972558990011478 ) ) ;
#12104=CARTESIAN_POINT ( 'NONE',  ( -2.547328955960238000E-13, 30.49999999999999645, 49.99999999999999289 ) ) ;
#12117=CARTESIAN_POINT ( 'NONE',  ( -1.240322475938754499E-13, 36.28125000068280315, 50.00000000000000000 ) ) ;
#12120=CARTESIAN_POINT ( 'NONE',  ( 30.81806926056962936, 37.15937500034139873, -42.41743335407647209 ) ) ;
#12122=CARTESIAN_POINT ( 'NONE',  ( -40.34137639590981195, 46.05937500034139731, 29.30972558990012189 ) ) ;
#12125=CARTESIAN_POINT ( 'NONE',  ( -49.93234176562499727, 49.96093750017070079, 0.000000000000000000 ) ) ;
#12128=CARTESIAN_POINT ( 'NONE',  ( -50.00000000000000000, 50.00000000000000000, 0.000000000000000000 ) ) ;
#12145=CARTESIAN_POINT ( 'NONE',  ( 8.446640517145639571E-15, 28.49999999999999645, 50.00000000000000000 ) ) ;
#12151=CARTESIAN_POINT ( 'NONE',  ( 49.86468353124999453, 21.02187500034139589, -16.20201782572376104 ) ) ;
#12154=CARTESIAN_POINT ( 'NONE',  ( 15.40903463028482356, 28.45937500034139589, 47.42413220539093999 ) ) ;
#12155=CARTESIAN_POINT ( 'NONE',  ( -30.90169943749473447, 30.29999999999999716, 42.53254041760200721 ) ) ;
#12163=CARTESIAN_POINT ( 'NONE',  ( 40.45084971874737789, 34.80000000000000426, 29.38926261462365375 ) ) ;
#12165=CARTESIAN_POINT ( 'NONE',  ( -49.86468353125000164, 31.92187500034139447, 0.000000000000000000 ) ) ;
#12166=CARTESIAN_POINT ( 'NONE',  ( 40.34137639590981905, 26.65937500034139518, 29.30972558990010768 ) ) ;
#12171=AXIS2_PLACEMENT_3D ( 'NONE', #3583, #14958, #4585 ) ;
#12172=CARTESIAN_POINT ( 'NONE',  ( -30.81806926056962226, 48.15937500034139873, 42.41743335407647919 ) ) ;
#12175=CARTESIAN_POINT ( 'NONE',  ( -15.40903463028480580, 24.32187500034139660, 47.42413220539094709 ) ) ;
#12184=CARTESIAN_POINT ( 'NONE',  ( -30.81806926056962226, 46.22187500034139163, 42.41743335407647919 ) ) ;
#12187=CARTESIAN_POINT ( 'NONE',  ( 30.90169943749475578, 36.70000000000000995, 42.53254041760200010 ) ) ;
#12190=CARTESIAN_POINT ( 'NONE',  ( 9.631387414534489405E-15, 42.42187500034140157, 52.43083105670540789 ) ) ;
#12191=DIRECTION ( 'NONE',  ( -0.000000000000000000, 1.000000000000000000, -0.000000000000000000 ) ) ;
#12200=CARTESIAN_POINT ( 'NONE',  ( 2.600676159226420495E-13, 21.28125000068279604, -49.99999999999999289 ) ) ;
#12202=AXIS2_PLACEMENT_3D ( 'NONE', #16458, #7407, #13948 ) ;
#12203=CARTESIAN_POINT ( 'NONE',  ( 49.86468353125000164, 34.85937500034140157, -6.106662507704105588E-15 ) ) ;
#12207=EDGE_CURVE ( 'NONE', #9978, #13696, #15391, .T. ) ;
#12211=CARTESIAN_POINT ( 'NONE',  ( -40.45084971874737079, 46.20000000000000284, 29.38926261462367151 ) ) ;
#12220=CARTESIAN_POINT ( 'NONE',  ( -50.00000000000000000, 40.00000000000000000, 0.000000000000000000 ) ) ;
#12221=CARTESIAN_POINT ( 'NONE',  ( 7.919222016226822092, 28.55125428154684286, 49.99999999999999289 ) ) ;
#12225=CARTESIAN_POINT ( 'NONE',  ( -7.303768060548744501, 6.586594804128637293, 98.56982794341932674 ) ) ;
#12231=EDGE_CURVE ( 'NONE', #13242, #13993, #13041, .T. ) ;
#12232=CARTESIAN_POINT ( 'NONE',  ( -15.40903463028481646, 25.52187500034139589, -47.42413220539093999 ) ) ;
#12235=CARTESIAN_POINT ( 'NONE',  ( 40.34137639590981905, 26.65937500034139518, 29.30972558990010768 ) ) ;
#12236=EDGE_CURVE ( 'NONE', #14391, #6257, #6276, .T. ) ;
#12246=CARTESIAN_POINT ( 'NONE',  ( 15.40903463028482356, 30.52187500034139589, 47.42413220539093999 ) ) ;
#12247=CARTESIAN_POINT ( 'NONE',  ( 9.631387414534489405E-15, 28.35937500034139447, 52.43083105670540789 ) ) ;
#12248=CARTESIAN_POINT ( 'NONE',  ( -7.919222016226870942, 36.44874571845315359, 49.99999999999997158 ) ) ;
#12251=CARTESIAN_POINT ( 'NONE',  ( 49.86468353124999453, 44.95937500034139589, -16.20201782572376459 ) ) ;
#12254=CARTESIAN_POINT ( 'NONE',  ( -49.86468353124999453, 22.02187500034139589, 16.20201782572377525 ) ) ;
#12256=ORIENTED_EDGE ( 'NONE', *, *, #1740, .T. ) ;
#12260=ORIENTED_EDGE ( 'NONE', *, *, #7525, .F. ) ;
#12263=CARTESIAN_POINT ( 'NONE',  ( -15.40903463028481646, 21.45937500034139589, -47.42413220539093999 ) ) ;
#12264=CARTESIAN_POINT ( 'NONE',  ( 6.123233995736766085E-15, 20.00000000000000355, -50.00000000000000000 ) ) ;
#12266=CARTESIAN_POINT ( 'NONE',  ( -30.90169943749473802, 32.08125000068280031, 42.53254041760200721 ) ) ;
#12267=CARTESIAN_POINT ( 'NONE',  ( -3.210462471511496205E-15, 39.42187500034140157, -52.43083105670540789 ) ) ;
#12279=CARTESIAN_POINT ( 'NONE',  ( 50.00000000000000000, 21.00000000000000000, -6.123233995736766085E-15 ) ) ;
#12280=CARTESIAN_POINT ( 'NONE',  ( 30.81806926056964002, 36.55937500034139731, 42.41743335407647209 ) ) ;
#12281=LINE ( 'NONE', #3144, #78 ) ;
#12287=CARTESIAN_POINT ( 'NONE',  ( 15.45084971874737789, 36.60000000000000142, 47.55282581475767500 ) ) ;
#12294=EDGE_CURVE ( 'NONE', #4062, #4716, #3139, .T. ) ;
#12299=CARTESIAN_POINT ( 'NONE',  ( -40.45084971874737789, 47.58125000068280031, -29.38926261462365730 ) ) ;
#12301=EDGE_CURVE ( 'NONE', #6257, #14391, #11609, .T. ) ;
#12308=CARTESIAN_POINT ( 'NONE',  ( -40.45084971874737079, 47.98125000068279888, 29.38926261462367151 ) ) ;
#12312=CARTESIAN_POINT ( 'NONE',  ( -49.86468353125000164, 25.85937500034139802, 0.000000000000000000 ) ) ;
#12316=ORIENTED_EDGE ( 'NONE', *, *, #3672, .F. ) ;
#12323=CARTESIAN_POINT ( 'NONE',  ( 40.45084971874737789, 28.58125000068280031, 29.38926261462365375 ) ) ;
#12326=CARTESIAN_POINT ( 'NONE',  ( -49.86468353124999453, 28.02187500034139234, 16.20201782572377525 ) ) ;
#12327=CARTESIAN_POINT ( 'NONE',  ( -15.40903463028481646, 27.45937500034139944, -47.42413220539093999 ) ) ;
#12328=CARTESIAN_POINT ( 'NONE',  ( 40.45084971874737079, 26.98125000068279888, -29.38926261462366440 ) ) ;
#12332=CARTESIAN_POINT ( 'NONE',  ( -30.81806926056963292, 47.55937500034139731, -42.41743335407647209 ) ) ;
#12335=CARTESIAN_POINT ( 'NONE',  ( -40.34137639590981905, 21.72187500034139518, -29.30972558990011478 ) ) ;
#12338=AXIS2_PLACEMENT_3D ( 'NONE', #568, #1663, #14375 ) ;
#12345=CARTESIAN_POINT ( 'NONE',  ( 15.40903463028482356, 20.45937500034139589, 47.42413220539093999 ) ) ;
#12349=CARTESIAN_POINT ( 'NONE',  ( -15.45084971874736368, 34.18125000068279462, 47.55282581475768211 ) ) ;
#12350=CARTESIAN_POINT ( 'NONE',  ( 40.34137639590981905, 40.72187500034139873, 29.30972558990010768 ) ) ;
#12356=EDGE_LOOP ( 'NONE', ( #15294, #4753, #366, #13842 ) ) ;
#12366=CARTESIAN_POINT ( 'NONE',  ( -40.34137639590981905, 39.65937500034139873, -29.30972558990011478 ) ) ;
#12367=CARTESIAN_POINT ( 'NONE',  ( 49.86468353125001585, 42.75937500034138594, 16.20201782572375038 ) ) ;
#12385=ORIENTED_EDGE ( 'NONE', *, *, #12443, .F. ) ;
#12392=( LENGTH_UNIT ( ) NAMED_UNIT ( * ) SI_UNIT ( .MILLI., .METRE. ) );
#12393=AXIS2_PLACEMENT_3D ( 'NONE', #9743, #11068, #9822 ) ;
#12395=CARTESIAN_POINT ( 'NONE',  ( -7.919222016226804328, 48.22999571913595673, 50.00000000000000000 ) ) ;
#12397=CARTESIAN_POINT ( 'NONE',  ( -15.72597079336059167, 14.80126021712191964, 96.11250979253432547 ) ) ;
#12403=CARTESIAN_POINT ( 'NONE',  ( -49.99999999999999289, 49.68125000068279462, -16.24598481164531449 ) ) ;
#12407=CARTESIAN_POINT ( 'NONE',  ( 30.81806926056964002, 22.55937500034139020, 42.41743335407647209 ) ) ;
#12419=CARTESIAN_POINT ( 'NONE',  ( 1.293669679204937499E-13, 41.28125000068279604, -50.00000000000000000 ) ) ;
#12420=CARTESIAN_POINT ( 'NONE',  ( 7.919222016226809657, 35.44874571845314648, -50.00000000000000000 ) ) ;
#12422=CARTESIAN_POINT ( 'NONE',  ( 40.34137639590981905, 22.72187500034139518, 29.30972558990010768 ) ) ;
#12423=CARTESIAN_POINT ( 'NONE',  ( 30.81806926056962936, 27.15937500034139163, -42.41743335407646498 ) ) ;
#12424=CARTESIAN_POINT ( 'NONE',  ( -3.111920190527341144E-15, 27.28125000068279604, -50.00000000000000000 ) ) ;
#12425=CARTESIAN_POINT ( 'NONE',  ( -15.40903463028481646, 33.52187500034140299, -47.42413220539093999 ) ) ;
#12427=CARTESIAN_POINT ( 'NONE',  ( -15.40903463028480580, 38.25937500034140015, 47.42413220539094709 ) ) ;
#12430=CARTESIAN_POINT ( 'NONE',  ( -49.99999999999999289, 45.89999999999999858, -16.24598481164531449 ) ) ;
#12436=CARTESIAN_POINT ( 'NONE',  ( 40.45084971874737789, 40.58125000068280031, 29.38926261462365375 ) ) ;
#12437=CARTESIAN_POINT ( 'NONE',  ( -30.81806926056963292, 39.62187500034138310, -42.41743335407647209 ) ) ;
#12441=CARTESIAN_POINT ( 'NONE',  ( 15.45084971874737789, 36.38125000068279746, 47.55282581475767500 ) ) ;
#12443=EDGE_CURVE ( 'NONE', #12012, #15007, #5738, .T. ) ;
#12444=CARTESIAN_POINT ( 'NONE',  ( 9.631387414534489405E-15, 36.42187500034139447, 52.43083105670540789 ) ) ;
#12450=VERTEX_POINT ( 'NONE', #8370 ) ;
#12455=CARTESIAN_POINT ( 'NONE',  ( -30.81806926056963292, 37.55937500034139020, -42.41743335407647209 ) ) ;
#12456=CARTESIAN_POINT ( 'NONE',  ( 30.81806926056962936, 41.15937500034139873, -42.41743335407646498 ) ) ;
#12462=CARTESIAN_POINT ( 'NONE',  ( -50.00000000000000000, 20.00000000000000000, 0.000000000000000000 ) ) ;
#12466=ADVANCED_FACE ( 'NONE', ( #720 ), #7139, .F. ) ;
#12470=VERTEX_POINT ( 'NONE', #627 ) ;
#12473=CARTESIAN_POINT ( 'NONE',  ( 49.99999999999999289, 29.10000000000000142, -16.24598481164532160 ) ) ;
#12477=CARTESIAN_POINT ( 'NONE',  ( -9.335200319780161848, 7.686841762321760640, 98.20306808818041588 ) ) ;
#12482=SURFACE_STYLE_USAGE ( .BOTH. , #68 ) ;
#12484=CARTESIAN_POINT ( 'NONE',  ( 30.90169943749475578, 46.48125000068280599, 42.53254041760200010 ) ) ;
#12487=CARTESIAN_POINT ( 'NONE',  ( -50.00000000000000000, 26.00000000000000355, 0.000000000000000000 ) ) ;
#12488=CARTESIAN_POINT ( 'NONE',  ( 1.293669679204937499E-13, 41.28125000068279604, -50.00000000000000000 ) ) ;
#12491=CARTESIAN_POINT ( 'NONE',  ( -5.823736356558307894E-14, 44.50000000000000000, 50.00000000000000000 ) ) ;
#12496=LINE ( 'NONE', #9533, #2804 ) ;
#12499=CARTESIAN_POINT ( 'NONE',  ( -49.86468353124999453, 20.02187500034139589, 16.20201782572377525 ) ) ;
#12500=CARTESIAN_POINT ( 'NONE',  ( 49.86468353125001585, 30.75937500034139305, 16.20201782572375038 ) ) ;
#12502=CARTESIAN_POINT ( 'NONE',  ( -40.34137639590981195, 36.12187500034139731, 29.30972558990012189 ) ) ;
#12504=CARTESIAN_POINT ( 'NONE',  ( -15.45084971874736368, 36.39999999999999858, 47.55282581475768211 ) ) ;
#12505=CARTESIAN_POINT ( 'NONE',  ( -30.81806926056962226, 40.15937500034139163, 42.41743335407647919 ) ) ;
#12508=CARTESIAN_POINT ( 'NONE',  ( 9.657523855033129090E-15, 42.50000000000000711, 52.57311121191334990 ) ) ;
#12515=CARTESIAN_POINT ( 'NONE',  ( 0.000000000000000000, 20.00000000000000355, 50.00000000000000000 ) ) ;
#12517=CARTESIAN_POINT ( 'NONE',  ( -3.210462471511496205E-15, 39.42187500034140157, -52.43083105670540789 ) ) ;
#12520=CARTESIAN_POINT ( 'NONE',  ( -15.45084971874737256, 27.38125000068280102, -47.55282581475767500 ) ) ;
#12522=CARTESIAN_POINT ( 'NONE',  ( -30.81806926056962226, 32.22187500034139163, 42.41743335407647919 ) ) ;
#12529=CARTESIAN_POINT ( 'NONE',  ( -49.86468353125000164, 49.92187500034140157, 0.000000000000000000 ) ) ;
#12531=CARTESIAN_POINT ( 'NONE',  ( -30.90169943749474513, 21.48125000068279533, -42.53254041760200721 ) ) ;
#12533=CARTESIAN_POINT ( 'NONE',  ( -40.34137639590981905, 29.65937500034139518, -29.30972558990011478 ) ) ;
#12537=DIRECTION ( 'NONE',  ( 0.000000000000000000, 0.000000000000000000, 1.000000000000000000 ) ) ;
#12541=VERTEX_POINT ( 'NONE', #1958 ) ;
#12545=CARTESIAN_POINT ( 'NONE',  ( 30.90169943749473802, 35.08125000068278609, -42.53254041760200721 ) ) ;
#12550=CARTESIAN_POINT ( 'NONE',  ( -40.34137639590981905, 47.65937500034139873, -29.30972558990011478 ) ) ;
#12553=CARTESIAN_POINT ( 'NONE',  ( 8.660254037844387298, 28.00000000000000355, 5.000000000000000000 ) ) ;
#12558=CARTESIAN_POINT ( 'NONE',  ( -15.45084971874737256, 47.38125000068279746, -47.55282581475767500 ) ) ;
#12561=CARTESIAN_POINT ( 'NONE',  ( -30.81806926056962226, 20.15937500034139518, 42.41743335407647919 ) ) ;
#12568=CARTESIAN_POINT ( 'NONE',  ( 8.446640517145639571E-15, 48.28125000068279604, 50.00000000000000000 ) ) ;
#12574=CARTESIAN_POINT ( 'NONE',  ( 30.81806926056964002, 24.62187500034139731, 42.41743335407647209 ) ) ;
#12575=CARTESIAN_POINT ( 'NONE',  ( -15.40903463028481646, 23.45937500034139944, -47.42413220539093999 ) ) ;
#12577=CARTESIAN_POINT ( 'NONE',  ( 30.81806926056962936, 35.22187500034138452, -42.41743335407646498 ) ) ;
#12580=CARTESIAN_POINT ( 'NONE',  ( 15.45084971874736723, 37.40000000000000568, -47.55282581475768211 ) ) ;
#12581=CARTESIAN_POINT ( 'NONE',  ( 30.81806926056962936, 39.15937500034139873, -42.41743335407647209 ) ) ;
#12583=CARTESIAN_POINT ( 'NONE',  ( -40.45084971874737789, 47.80000000000000426, -29.38926261462365730 ) ) ;
#12584=ORIENTED_EDGE ( 'NONE', *, *, #2739, .F. ) ;
#12588=ORIENTED_EDGE ( 'NONE', *, *, #1682, .T. ) ;
#12596=CARTESIAN_POINT ( 'NONE',  ( -49.86468353124999453, 39.82187500034140015, -16.20201782572375393 ) ) ;
#12599=CARTESIAN_POINT ( 'NONE',  ( 50.00000000000000000, 26.78125000068279959, -6.123233995736766085E-15 ) ) ;
#12601=CARTESIAN_POINT ( 'NONE',  ( 14.26382420819190955, 32.65508274695842061, 93.15685069300390353 ) ) ;
#12602=CARTESIAN_POINT ( 'NONE',  ( -49.86468353124999453, 36.02187500034139589, 16.20201782572377525 ) ) ;
#12607=ORIENTED_EDGE ( 'NONE', *, *, #7834, .F. ) ;
#12610=VECTOR ( 'NONE', #7322, 1000.000000000000000 ) ;
#12614=CARTESIAN_POINT ( 'NONE',  ( -15.40903463028480580, 30.25937500034140015, 47.42413220539094709 ) ) ;
#12616=CARTESIAN_POINT ( 'NONE',  ( -49.86468353124999453, 44.02187500034139589, 16.20201782572377169 ) ) ;
#12627=ORIENTED_EDGE ( 'NONE', *, *, #12443, .T. ) ;
#12629=( BOUNDED_CURVE ( )  B_SPLINE_CURVE ( 2, ( #11465, #15365, #5408, #15689, #5644, #1808, #6741, #4316, #14194, #10466, #11953, #6577, #11711 ),
 .UNSPECIFIED., .F., .F. ) 
 B_SPLINE_CURVE_WITH_KNOTS ( ( 3, 2, 2, 2, 2, 2, 3 ),
 ( 0.3500000000000000333, 0.3533333333333333326, 0.3599999999999999867, 0.3666666666666666408, 0.3733333333333333504, 0.3800000000000000044, 0.3833333333333333592 ),
 .UNSPECIFIED. ) 
 CURVE ( )  GEOMETRIC_REPRESENTATION_ITEM ( )  RATIONAL_B_SPLINE_CURVE ( ( 0.9755282581475768211, 0.9755282581475770431, 1.000000000000000000, 0.9510565162951535312, 1.000000000000000000, 0.9510565162951535312, 1.000000000000000000, 0.9510565162951535312, 1.000000000000000000, 0.9510565162951535312, 1.000000000000000000, 0.9755282581475765991, 0.9755282581475768211 ) ) 
 REPRESENTATION_ITEM ( '' )  );
#12634=CARTESIAN_POINT ( 'NONE',  ( 49.86468353125001585, 48.75937500034140015, 16.20201782572375038 ) ) ;
#12644=CARTESIAN_POINT ( 'NONE',  ( 15.45084971874736723, 45.18125000068280173, -47.55282581475768211 ) ) ;
#12645=CARTESIAN_POINT ( 'NONE',  ( 50.00000000000000000, 21.00000000000000000, -6.123233995736766085E-15 ) ) ;
#12656=CARTESIAN_POINT ( 'NONE',  ( -8.660254037844387298, 20.00000000000000355, 5.000000000000000000 ) ) ;
#12661=CARTESIAN_POINT ( 'NONE',  ( -2.869705857872620669, 39.77257016122691624, 92.94441961119122197 ) ) ;
#12665=CARTESIAN_POINT ( 'NONE',  ( -40.34137639590981195, 20.05937500034139731, 29.30972558990012189 ) ) ;
#12667=CARTESIAN_POINT ( 'NONE',  ( -49.86468353124999453, 38.02187500034139589, 16.20201782572377169 ) ) ;
#12670=CARTESIAN_POINT ( 'NONE',  ( 15.45084971874737789, 30.60000000000000142, 47.55282581475767500 ) ) ;
#12671=CARTESIAN_POINT ( 'NONE',  ( 40.34137639590981905, 36.65937500034139873, 29.30972558990010768 ) ) ;
#12673=CARTESIAN_POINT ( 'NONE',  ( 50.00000000000000711, 46.90000000000000568, 16.24598481164530739 ) ) ;
#12681=AXIS2_PLACEMENT_3D ( 'NONE', #472, #10388, #6659 ) ;
#12686=CARTESIAN_POINT ( 'NONE',  ( 49.86468353124999453, 43.02187500034138878, -16.20201782572376459 ) ) ;
#12689=CARTESIAN_POINT ( 'NONE',  ( -15.45084971874737256, 29.38125000068279746, -47.55282581475767500 ) ) ;
#12691=CARTESIAN_POINT ( 'NONE',  ( 49.86468353124999453, 35.02187500034139589, -16.20201782572376459 ) ) ;
#12699=CARTESIAN_POINT ( 'NONE',  ( 9.631387414534489405E-15, 28.35937500034139802, 52.43083105670540789 ) ) ;
#12701=CARTESIAN_POINT ( 'NONE',  ( -40.34137639590981905, 47.72187500034139873, -29.30972558990011478 ) ) ;
#12709=CARTESIAN_POINT ( 'NONE',  ( -15.45084971874736368, 46.18125000068280173, 47.55282581475768211 ) ) ;
#12711=ORIENTED_EDGE ( 'NONE', *, *, #6034, .T. ) ;
#12721=CARTESIAN_POINT ( 'NONE',  ( 1.022488062601840571E-14, 49.28125000068280315, -50.00000000000000000 ) ) ;
#12724=CARTESIAN_POINT ( 'NONE',  ( 0.000000000000000000, 20.00000000000000355, 0.000000000000000000 ) ) ;
#12725=CARTESIAN_POINT ( 'NONE',  ( -49.99999999999999289, 43.68125000068279462, -16.24598481164531449 ) ) ;
#12727=CARTESIAN_POINT ( 'NONE',  ( 30.90169943749473802, 47.08125000068280031, -42.53254041760200721 ) ) ;
#12734=CARTESIAN_POINT ( 'NONE',  ( 15.45084971874737789, 42.38125000068279746, 47.55282581475767500 ) ) ;
#12738=CARTESIAN_POINT ( 'NONE',  ( 50.00000000000000000, 33.00000000000000000, -6.123233995736766085E-15 ) ) ;
#12743=VECTOR ( 'NONE', #11637, 1000.000000000000000 ) ;
#12744=CARTESIAN_POINT ( 'NONE',  ( -3.210462471511496205E-15, 21.35937500034139447, -52.43083105670540789 ) ) ;
#12746=CARTESIAN_POINT ( 'NONE',  ( -40.34137639590981905, 37.72187500034139873, -29.30972558990011478 ) ) ;
#12748=CARTESIAN_POINT ( 'NONE',  ( -49.99999999999999289, 30.10000000000000497, 16.24598481164533226 ) ) ;
#12749=CARTESIAN_POINT ( 'NONE',  ( 49.86468353125000164, 36.85937500034139447, -6.106662507704105588E-15 ) ) ;
#12751=CARTESIAN_POINT ( 'NONE',  ( -40.45084971874737789, 43.80000000000000426, -29.38926261462365730 ) ) ;
#12753=ORIENTED_EDGE ( 'NONE', *, *, #14017, .T. ) ;
#12756=ORIENTED_EDGE ( 'NONE', *, *, #15358, .F. ) ;
#12760=DIRECTION ( 'NONE',  ( 0.000000000000000000, 1.000000000000000000, 0.000000000000000000 ) ) ;
#12763=CARTESIAN_POINT ( 'NONE',  ( 30.81806926056964002, 44.62187500034140442, 42.41743335407647209 ) ) ;
#12764=CARTESIAN_POINT ( 'NONE',  ( -49.86468353125000164, 39.85937500034139447, 0.000000000000000000 ) ) ;
#12767=EDGE_CURVE ( 'NONE', #6301, #4835, #151, .T. ) ;
#12768=CARTESIAN_POINT ( 'NONE',  ( -40.45084971874737789, 25.58125000068279675, -29.38926261462365730 ) ) ;
#12770=CARTESIAN_POINT ( 'NONE',  ( 40.34137639590981905, 34.72187500034139873, 29.30972558990010768 ) ) ;
#12771=CARTESIAN_POINT ( 'NONE',  ( -15.45084971874736368, 28.40000000000000213, 47.55282581475768211 ) ) ;
#12773=ORIENTED_EDGE ( 'NONE', *, *, #8132, .T. ) ;
#12777=DIRECTION ( 'NONE',  ( -0.000000000000000000, 1.000000000000000000, -0.000000000000000000 ) ) ;
#12778=CARTESIAN_POINT ( 'NONE',  ( -49.86468353124999453, 33.95937500034139589, 16.20201782572377525 ) ) ;
#12780=CARTESIAN_POINT ( 'NONE',  ( 40.34137639590981195, 49.12187500034139731, -29.30972558990011834 ) ) ;
#12786=EDGE_LOOP ( 'NONE', ( #10490, #3070, #15439, #15917 ) ) ;
#12790=CARTESIAN_POINT ( 'NONE',  ( 15.45084971874736723, 35.18125000068280173, -47.55282581475768211 ) ) ;
#12794=CARTESIAN_POINT ( 'NONE',  ( -49.86468353124999453, 49.75937500034138594, -16.20201782572375393 ) ) ;
#12800=CARTESIAN_POINT ( 'NONE',  ( 50.00000000000000711, 38.68125000068280173, 16.24598481164530739 ) ) ;
#12801=CARTESIAN_POINT ( 'NONE',  ( 30.90169943749475223, 44.48125000068279888, 42.53254041760199300 ) ) ;
#12814=CARTESIAN_POINT ( 'NONE',  ( 7.919222016226693306, 32.55125428154685352, 50.00000000000003553 ) ) ;
#12820=CARTESIAN_POINT ( 'NONE',  ( 9.631387414534489405E-15, 22.35937500034139802, 52.43083105670540789 ) ) ;
#12822=CARTESIAN_POINT ( 'NONE',  ( -40.34137639590981195, 30.12187500034139731, 29.30972558990012189 ) ) ;
#12825=CARTESIAN_POINT ( 'NONE',  ( 15.45084971874736723, 29.40000000000000213, -47.55282581475768211 ) ) ;
#12826=CARTESIAN_POINT ( 'NONE',  ( 49.86468353124999453, 32.95937500034138168, -16.20201782572376459 ) ) ;
#12829=CARTESIAN_POINT ( 'NONE',  ( -30.90169943749474868, 41.70000000000000284, -42.53254041760200721 ) ) ;
#12842=CARTESIAN_POINT ( 'NONE',  ( 49.86468353125001585, 34.82187500034140015, 16.20201782572375038 ) ) ;
#12843=CARTESIAN_POINT ( 'NONE',  ( -40.34137639590981905, 41.65937500034139873, -29.30972558990011478 ) ) ;
#12844=CARTESIAN_POINT ( 'NONE',  ( -7.919222016226838967, 44.44874571845315359, 49.99999999999999289 ) ) ;
#12846=CARTESIAN_POINT ( 'NONE',  ( 49.99999999999999289, 28.88125000068279391, -16.24598481164532160 ) ) ;
#12847=CARTESIAN_POINT ( 'NONE',  ( 11.57959921299713457, 35.63367363361179230, 92.99972171590198400 ) ) ;
#12848=CARTESIAN_POINT ( 'NONE',  ( 49.86468353124999453, 29.02187500034139234, -16.20201782572376459 ) ) ;
#12849=EDGE_CURVE ( 'NONE', #15936, #11630, #10839, .T. ) ;
#12859=CARTESIAN_POINT ( 'NONE',  ( -30.81806926056963292, 31.55937500034139731, -42.41743335407647209 ) ) ;
#12862=CARTESIAN_POINT ( 'NONE',  ( -40.34137639590981195, 48.12187500034139731, 29.30972558990012189 ) ) ;
#12867=( BOUNDED_CURVE ( )  B_SPLINE_CURVE ( 2, ( #16233, #13647, #11002, #5774, #15905, #9843, #14895, #13487, #12323, #10919, #9592, #8503, #14719 ),
 .UNSPECIFIED., .F., .F. ) 
 B_SPLINE_CURVE_WITH_KNOTS ( ( 3, 2, 2, 2, 2, 2, 3 ),
 ( 0.6833333333333333481, 0.6866666666666666474, 0.6933333333333333570, 0.6999999999999999556, 0.7066666666666666652, 0.7133333333333333748, 0.7166666666666666741 ),
 .UNSPECIFIED. ) 
 CURVE ( )  GEOMETRIC_REPRESENTATION_ITEM ( )  RATIONAL_B_SPLINE_CURVE ( ( 0.9755282581475768211, 0.9755282581475768211, 1.000000000000000000, 0.9510565162951535312, 1.000000000000000000, 0.9510565162951535312, 1.000000000000000000, 0.9510565162951535312, 1.000000000000000000, 0.9510565162951535312, 1.000000000000000000, 0.9755282581475768211, 0.9755282581475768211 ) ) 
 REPRESENTATION_ITEM ( '' )  );
#12871=ORIENTED_EDGE ( 'NONE', *, *, #1637, .F. ) ;
#12873=( GEOMETRIC_REPRESENTATION_CONTEXT ( 3 ) GLOBAL_UNCERTAINTY_ASSIGNED_CONTEXT ( ( #15900 ) ) GLOBAL_UNIT_ASSIGNED_CONTEXT ( ( #12392, #9895, #2072 ) ) REPRESENTATION_CONTEXT ( 'NONE', 'WORKASPACE' ) );
#12875=CARTESIAN_POINT ( 'NONE',  ( -2.547328955960238000E-13, 34.28125000068279604, 49.99999999999999289 ) ) ;
#12878=CARTESIAN_POINT ( 'NONE',  ( 15.45084971874736723, 25.40000000000000213, -47.55282581475768211 ) ) ;
#12879=CARTESIAN_POINT ( 'NONE',  ( 15.45084971874736723, 33.18125000068279462, -47.55282581475768211 ) ) ;
#12880=CARTESIAN_POINT ( 'NONE',  ( -50.00000000000000000, 31.78125000068279959, 0.000000000000000000 ) ) ;
#12882=CARTESIAN_POINT ( 'NONE',  ( 49.86468353125000164, 22.92187500034139802, -6.106662507704105588E-15 ) ) ;
#12884=CARTESIAN_POINT ( 'NONE',  ( -30.90169943749473802, 40.08125000068279320, 42.53254041760200721 ) ) ;
#12890=VERTEX_POINT ( 'NONE', #11689 ) ;
#12892=VERTEX_POINT ( 'NONE', #10538 ) ;
#12893=CARTESIAN_POINT ( 'NONE',  ( 40.45084971874737789, 42.80000000000000426, 29.38926261462365375 ) ) ;
#12899=CARTESIAN_POINT ( 'NONE',  ( 8.446640517145639571E-15, 28.28125000068279959, 50.00000000000000000 ) ) ;
#12900=CARTESIAN_POINT ( 'NONE',  ( -6.186240466588083464, 38.88034870839190660, 92.94021688847078622 ) ) ;
#12906=CARTESIAN_POINT ( 'NONE',  ( -49.86468353124999453, 21.75937500034139305, -16.20201782572375393 ) ) ;
#12907=LINE ( 'NONE', #258, #11078 ) ;
#12908=CARTESIAN_POINT ( 'NONE',  ( 15.40903463028482356, 30.52187500034139589, 47.42413220539093999 ) ) ;
#12910=CLOSED_SHELL ( 'NONE', ( #16254, #6355, #3160, #11494, #15749, #3425, #13525, #11722, #15523, #10290, #12466, #11401, #406, #5731, #9297, #11989, #13412, #10090, #2134, #13267, #11951, #11190, #2234, #4391, #5490, #8749, #6773, #659, #10686, #7928, #16047, #2434, #3569, #1925, #7580, #15767, #4016, #503, #6987, #6430, #7780, #3723, #15701, #2009, #13646, #14032, #8663, #13165, #7437, #10981, #8252 ) ) ;
#12911=CARTESIAN_POINT ( 'NONE',  ( 30.90169943749475578, 30.70000000000000284, 42.53254041760200010 ) ) ;
#12912=CARTESIAN_POINT ( 'NONE',  ( -15.40903463028480580, 30.25937500034140015, 47.42413220539094709 ) ) ;
#12921=ORIENTED_EDGE ( 'NONE', *, *, #15235, .F. ) ;
#12922=DIRECTION ( 'NONE',  ( 0.000000000000000000, -0.9848077530122080203, 0.1736481776669307198 ) ) ;
#12925=CONICAL_SURFACE ( 'NONE', #2567, 100.0000000000000000, 0.1745329251994333364 ) ;
#12926=CARTESIAN_POINT ( 'NONE',  ( -40.45084971874737789, 37.79999999999999716, -29.38926261462365730 ) ) ;
#12930=CARTESIAN_POINT ( 'NONE',  ( -15.40903463028480580, 34.32187500034139305, 47.42413220539094709 ) ) ;
#12931=CARTESIAN_POINT ( 'NONE',  ( 9.631387414534489405E-15, 44.35937500034140157, 52.43083105670540789 ) ) ;
#12935=CARTESIAN_POINT ( 'NONE',  ( 49.99999999999999289, 20.88125000068279746, -16.24598481164532160 ) ) ;
#12937=CARTESIAN_POINT ( 'NONE',  ( -3.210462471511496205E-15, 29.42187500034139092, -52.43083105670540789 ) ) ;
#12948=CARTESIAN_POINT ( 'NONE',  ( 30.81806926056964002, 22.55937500034139020, 42.41743335407647209 ) ) ;
#12951=CARTESIAN_POINT ( 'NONE',  ( -3.210462471511496205E-15, 39.42187500034139447, -52.43083105670540789 ) ) ;
#12953=CARTESIAN_POINT ( 'NONE',  ( 49.86468353124999453, 45.02187500034138878, -16.20201782572376459 ) ) ;
#12954=DIRECTION ( 'NONE',  ( 0.000000000000000000, 1.000000000000000000, 0.000000000000000000 ) ) ;
#12965=CARTESIAN_POINT ( 'NONE',  ( 49.99999999999999289, 23.10000000000000497, -16.24598481164532160 ) ) ;
#12966=CARTESIAN_POINT ( 'NONE',  ( -15.40903463028481646, 45.45937500034139589, -47.42413220539093999 ) ) ;
#12969=CARTESIAN_POINT ( 'NONE',  ( 30.81806926056962936, 21.22187500034139518, -42.41743335407647209 ) ) ;
#12972=CARTESIAN_POINT ( 'NONE',  ( 9.657523855033129090E-15, 40.28125000068278894, 52.57311121191334990 ) ) ;
#12974=EDGE_CURVE ( 'NONE', #5249, #12890, #4572, .T. ) ;
#12975=CARTESIAN_POINT ( 'NONE',  ( 40.45084971874737789, 46.58125000068280031, 29.38926261462365375 ) ) ;
#12978=ORIENTED_EDGE ( 'NONE', *, *, #11943, .T. ) ;
#12981=CARTESIAN_POINT ( 'NONE',  ( 49.99999999999999289, 43.10000000000000142, -16.24598481164532160 ) ) ;
#12984=VERTEX_POINT ( 'NONE', #11334 ) ;
#12986=CARTESIAN_POINT ( 'NONE',  ( -17.36342088942478057, 24.75448731571099259, 94.04567196164467191 ) ) ;
#12990=CARTESIAN_POINT ( 'NONE',  ( 15.18950378164810822, 13.79078835917772672, 96.37912034925916771 ) ) ;
#12991=CARTESIAN_POINT ( 'NONE',  ( -46.73878613316165342, 20.00000000000001066, 17.37815620099909708 ) ) ;
#12992=CARTESIAN_POINT ( 'NONE',  ( -40.34137639590981905, 31.72187500034139873, -29.30972558990011478 ) ) ;
#12994=CONICAL_SURFACE ( 'NONE', #9020, 85.01963570546854498, 0.9599310885968793672 ) ;
#12995=CARTESIAN_POINT ( 'NONE',  ( -15.45084971874736368, 34.39999999999999858, 47.55282581475768211 ) ) ;
#12996=CARTESIAN_POINT ( 'NONE',  ( 49.86468353124999453, 30.95937500034139944, -16.20201782572376459 ) ) ;
#13008=CARTESIAN_POINT ( 'NONE',  ( -30.81806926056962226, 38.22187500034139873, 42.41743335407647919 ) ) ;
#13009=CARTESIAN_POINT ( 'NONE',  ( 49.86468353124999453, 32.95937500034138878, -16.20201782572376104 ) ) ;
#13013=CARTESIAN_POINT ( 'NONE',  ( -40.45084971874737079, 21.98125000068279888, 29.38926261462367151 ) ) ;
#13015=CARTESIAN_POINT ( 'NONE',  ( -30.81806926056963292, 25.62187500034139731, -42.41743335407647209 ) ) ;
#13022=CARTESIAN_POINT ( 'NONE',  ( 1.022488062601840571E-14, 49.28125000068280315, -50.00000000000000000 ) ) ;
#13026=CARTESIAN_POINT ( 'NONE',  ( -15.40903463028480580, 24.25937500034139660, 47.42413220539094709 ) ) ;
#13029=CARTESIAN_POINT ( 'NONE',  ( 15.40903463028482356, 42.52187500034139589, 47.42413220539093999 ) ) ;
#13032=CARTESIAN_POINT ( 'NONE',  ( -49.86468353125000164, 45.92187500034139447, 0.000000000000000000 ) ) ;
#13037=ORIENTED_EDGE ( 'NONE', *, *, #15336, .T. ) ;
#13039=ORIENTED_EDGE ( 'NONE', *, *, #13228, .F. ) ;
#13041=LINE ( 'NONE', #11785, #410 ) ;
#13043=CARTESIAN_POINT ( 'NONE',  ( 0.000000000000000000, 0.000000000000000000, 100.0000000000000000 ) ) ;
#13044=CARTESIAN_POINT ( 'NONE',  ( 15.45084971874737789, 26.60000000000000142, 47.55282581475767500 ) ) ;
#13045=CARTESIAN_POINT ( 'NONE',  ( -49.86468353125000164, 45.85937500034140157, 0.000000000000000000 ) ) ;
#13046=CARTESIAN_POINT ( 'NONE',  ( -30.90169943749473447, 26.08125000068279320, 42.53254041760200721 ) ) ;
#13049=LINE ( 'NONE', #12125, #1503 ) ;
#13052=CARTESIAN_POINT ( 'NONE',  ( 49.99999999999999289, 42.88125000068278325, -16.24598481164532160 ) ) ;
#13061=DIRECTION ( 'NONE',  ( -0.000000000000000000, 1.000000000000000000, -0.000000000000000000 ) ) ;
#13070=CARTESIAN_POINT ( 'NONE',  ( -7.919222016226752814, 37.33250428222964246, -50.00000000000000711 ) ) ;
#13071=CARTESIAN_POINT ( 'NONE',  ( -46.25745152662948811, 20.00000000000000355, 18.62156331808021648 ) ) ;
#13072=CARTESIAN_POINT ( 'NONE',  ( 40.34137639590981195, 31.12187500034139731, -29.30972558990011834 ) ) ;
#13075=CARTESIAN_POINT ( 'NONE',  ( -40.34137639590981195, 30.05937500034139731, 29.30972558990012189 ) ) ;
#13086=CARTESIAN_POINT ( 'NONE',  ( -15.40903463028481646, 33.52187500034140299, -47.42413220539093999 ) ) ;
#13087=CARTESIAN_POINT ( 'NONE',  ( -40.34137639590981195, 38.05937500034139731, 29.30972558990012189 ) ) ;
#13091=CARTESIAN_POINT ( 'NONE',  ( 30.81806926056962936, 49.15937500034138452, -42.41743335407647209 ) ) ;
#13094=CARTESIAN_POINT ( 'NONE',  ( 15.40903463028481113, 29.32187500034139660, -47.42413220539094709 ) ) ;
#13096=CARTESIAN_POINT ( 'NONE',  ( -49.99999999999999289, 27.68125000068279462, -16.24598481164531449 ) ) ;
#13104=CARTESIAN_POINT ( 'NONE',  ( -49.86468353124999453, 27.75937500034139660, -16.20201782572375393 ) ) ;
#13107=CARTESIAN_POINT ( 'NONE',  ( -40.34137639590981195, 40.12187500034139731, 29.30972558990012189 ) ) ;
#13108=VECTOR ( 'NONE', #13211, 1000.000000000000000 ) ;
#13109=CARTESIAN_POINT ( 'NONE',  ( 40.34137639590981905, 44.72187500034139163, 29.30972558990010768 ) ) ;
#13117=CARTESIAN_POINT ( 'NONE',  ( -49.99999999999999289, 43.88125000068279746, 16.24598481164533226 ) ) ;
#13119=CARTESIAN_POINT ( 'NONE',  ( -50.00000000000000000, 49.89062500034140157, 0.000000000000000000 ) ) ;
#13120=CARTESIAN_POINT ( 'NONE',  ( -40.45084971874737079, 26.20000000000000284, 29.38926261462367151 ) ) ;
#13121=CARTESIAN_POINT ( 'NONE',  ( 15.40903463028482356, 46.45937500034139589, 47.42413220539093999 ) ) ;
#13127=CARTESIAN_POINT ( 'NONE',  ( 40.45084971874737079, 36.98125000068279888, -29.38926261462366440 ) ) ;
#13130=CARTESIAN_POINT ( 'NONE',  ( 7.919222016226940219, 23.22999571913595673, -49.99999999999996447 ) ) ;
#13132=VERTEX_POINT ( 'NONE', #12899 ) ;
#13144=DIRECTION ( 'NONE',  ( -0.000000000000000000, 1.000000000000000000, -0.000000000000000000 ) ) ;
#13148=CARTESIAN_POINT ( 'NONE',  ( -45.11452830843730766, 20.00000000000000711, 21.24066852005664430 ) ) ;
#13151=CARTESIAN_POINT ( 'NONE',  ( -15.40903463028481646, 27.52187500034139944, -47.42413220539093999 ) ) ;
#13153=CARTESIAN_POINT ( 'NONE',  ( -49.86468353125000164, 29.85937500034139802, 0.000000000000000000 ) ) ;
#13156=VECTOR ( 'NONE', #8291, 1000.000000000000000 ) ;
#13158=ORIENTED_EDGE ( 'NONE', *, *, #8132, .F. ) ;
#13165=ADVANCED_FACE ( 'NONE', ( #6507 ), #14215, .T. ) ;
#13168=CARTESIAN_POINT ( 'NONE',  ( 49.86468353125001585, 36.82187500034140015, 16.20201782572375038 ) ) ;
#13169=CARTESIAN_POINT ( 'NONE',  ( 40.34137639590981905, 38.65937500034139873, 29.30972558990010768 ) ) ;
#13175=CARTESIAN_POINT ( 'NONE',  ( -3.219174618344376363E-15, 21.28125000068279959, -52.57311121191334990 ) ) ;
#13178=CARTESIAN_POINT ( 'NONE',  ( 40.34137639590981195, 25.12187500034139376, -29.30972558990011834 ) ) ;
#13184=VECTOR ( 'NONE', #12922, 1000.000000000000000 ) ;
#13190=CARTESIAN_POINT ( 'NONE',  ( -3.210462471511496205E-15, 25.35937500034139802, -52.43083105670540789 ) ) ;
#13192=CARTESIAN_POINT ( 'NONE',  ( -15.40903463028480580, 40.32187500034140015, 47.42413220539094709 ) ) ;
#13194=VECTOR ( 'NONE', #4931, 1000.000000000000000 ) ;
#13196=CARTESIAN_POINT ( 'NONE',  ( -49.86468353124999453, 47.82187500034140015, -16.20201782572375393 ) ) ;
#13198=EDGE_LOOP ( 'NONE', ( #7903, #3899, #8548, #1061 ) ) ;
#13206=CARTESIAN_POINT ( 'NONE',  ( -40.45084971874737079, 24.20000000000000284, 29.38926261462367151 ) ) ;
#13207=CARTESIAN_POINT ( 'NONE',  ( 49.86468353125000164, 46.85937500034139447, -6.106662507704105588E-15 ) ) ;
#13209=CARTESIAN_POINT ( 'NONE',  ( -2.547328955960238000E-13, 24.28125000068279604, 49.99999999999999289 ) ) ;
#13210=DIRECTION ( 'NONE',  ( -0.000000000000000000, 1.000000000000000000, -0.000000000000000000 ) ) ;
#13211=DIRECTION ( 'NONE',  ( -0.000000000000000000, 1.000000000000000000, -0.000000000000000000 ) ) ;
#13212=CARTESIAN_POINT ( 'NONE',  ( -40.45084971874737789, 33.58125000068280031, -29.38926261462365730 ) ) ;
#13228=EDGE_CURVE ( 'NONE', #4896, #6137, #11798, .T. ) ;
#13234=CARTESIAN_POINT ( 'NONE',  ( -15.45084971874736368, 38.18125000068280173, 47.55282581475768211 ) ) ;
#13235=CARTESIAN_POINT ( 'NONE',  ( 49.99999999999999289, 47.10000000000000142, -16.24598481164532160 ) ) ;
#13237=CARTESIAN_POINT ( 'NONE',  ( -15.40903463028481646, 23.52187500034139944, -47.42413220539093999 ) ) ;
#13238=CARTESIAN_POINT ( 'NONE',  ( 2.600676159226420495E-13, 21.50000000000000000, -49.99999999999999289 ) ) ;
#13240=CARTESIAN_POINT ( 'NONE',  ( -40.34137639590981905, 27.65937500034139873, -29.30972558990011478 ) ) ;
#13242=VERTEX_POINT ( 'NONE', #173 ) ;
#13249=CARTESIAN_POINT ( 'NONE',  ( -15.40903463028481646, 31.52187500034139944, -47.42413220539093999 ) ) ;
#13250=CARTESIAN_POINT ( 'NONE',  ( 40.34137639590981195, 39.05937500034140442, -29.30972558990011834 ) ) ;
#13254=CARTESIAN_POINT ( 'NONE',  ( 50.00000000000000711, 20.68125000068280173, 16.24598481164530739 ) ) ;
#13256=CARTESIAN_POINT ( 'NONE',  ( -30.81806926056963292, 23.62187500034139731, -42.41743335407647209 ) ) ;
#13267=ADVANCED_FACE ( 'NONE', ( #5278 ), #10329, .F. ) ;
#13268=CARTESIAN_POINT ( 'NONE',  ( -15.40903463028481646, 23.45937500034139944, -47.42413220539093999 ) ) ;
#13270=VECTOR ( 'NONE', #2403, 1000.000000000000000 ) ;
#13272=CARTESIAN_POINT ( 'NONE',  ( -3.219174618344376363E-15, 37.50000000000000000, -52.57311121191334990 ) ) ;
#13273=CARTESIAN_POINT ( 'NONE',  ( 15.40903463028481113, 49.32187500034139305, -47.42413220539094709 ) ) ;
#13275=VERTEX_POINT ( 'NONE', #6850 ) ;
#13277=ORIENTED_EDGE ( 'NONE', *, *, #8173, .T. ) ;
#13282=CARTESIAN_POINT ( 'NONE',  ( 30.90169943749475223, 36.48125000068279888, 42.53254041760199300 ) ) ;
#13283=CARTESIAN_POINT ( 'NONE',  ( -3.210462471511496205E-15, 45.35937500034139447, -52.43083105670540789 ) ) ;
#13284=CARTESIAN_POINT ( 'NONE',  ( 40.34137639590981905, 48.65937500034139873, 29.30972558990010768 ) ) ;
#13285=LINE ( 'NONE', #10394, #6635 ) ;
#13301=ORIENTED_EDGE ( 'NONE', *, *, #13600, .F. ) ;
#13304=CARTESIAN_POINT ( 'NONE',  ( 30.90169943749473802, 23.29999999999999716, -42.53254041760200721 ) ) ;
#13305=CARTESIAN_POINT ( 'NONE',  ( 0.000000000000000000, 0.000000000000000000, 0.000000000000000000 ) ) ;
#13311=CARTESIAN_POINT ( 'NONE',  ( -40.34137639590981195, 24.12187500034139731, 29.30972558990012189 ) ) ;
#13314=CARTESIAN_POINT ( 'NONE',  ( -49.86468353124999453, 23.75937500034140015, -16.20201782572375393 ) ) ;
#13322=EDGE_CURVE ( 'NONE', #9791, #14391, #572, .T. ) ;
#13325=CARTESIAN_POINT ( 'NONE',  ( -15.40903463028480580, 28.32187500034139660, 47.42413220539094709 ) ) ;
#13326=CARTESIAN_POINT ( 'NONE',  ( -40.34137639590981195, 34.05937500034139731, 29.30972558990012189 ) ) ;
#13330=CARTESIAN_POINT ( 'NONE',  ( 40.34137639590981905, 44.65937500034139163, 29.30972558990010768 ) ) ;
#13333=CARTESIAN_POINT ( 'NONE',  ( 9.657523855033129090E-15, 48.50000000000000000, 52.57311121191334990 ) ) ;
#13335=CARTESIAN_POINT ( 'NONE',  ( -49.99999999999999289, 27.88125000068280102, 16.24598481164533226 ) ) ;
#13336=ORIENTED_EDGE ( 'NONE', *, *, #4334, .T. ) ;
#13344=CARTESIAN_POINT ( 'NONE',  ( 49.86468353124999453, 20.95937500034138878, -16.20201782572376459 ) ) ;
#13347=CARTESIAN_POINT ( 'NONE',  ( -15.45084971874737256, 39.60000000000000142, -47.55282581475767500 ) ) ;
#13349=( BOUNDED_CURVE ( )  B_SPLINE_CURVE ( 2, ( #11474, #6169, #3677, #8812, #13876, #8733, #11400, #3832, #9726, #12801, #15202, #3916, #8897 ),
 .UNSPECIFIED., .F., .T. ) 
 B_SPLINE_CURVE_WITH_KNOTS ( ( 3, 2, 2, 2, 2, 2, 3 ),
 ( 0.1499999999999999944, 0.1533333333333333215, 0.1600000000000000033, 0.1666666666666666574, 0.1733333333333333393, 0.1799999999999999933, 0.1833333333333333481 ),
 .UNSPECIFIED. ) 
 CURVE ( )  GEOMETRIC_REPRESENTATION_ITEM ( )  RATIONAL_B_SPLINE_CURVE ( ( 0.9755282581475768211, 0.9755282581475768211, 1.000000000000000000, 0.9510565162951535312, 1.000000000000000000, 0.9510565162951535312, 1.000000000000000000, 0.9510565162951535312, 1.000000000000000000, 0.9510565162951535312, 1.000000000000000000, 0.9755282581475765991, 0.9755282581475767101 ) ) 
 REPRESENTATION_ITEM ( '' )  );
#13350=CARTESIAN_POINT ( 'NONE',  ( 30.81806926056962936, 39.22187500034139873, -42.41743335407647209 ) ) ;
#13351=CARTESIAN_POINT ( 'NONE',  ( 7.919222016226693306, 30.55125428154684286, 50.00000000000003553 ) ) ;
#13352=ORIENTED_EDGE ( 'NONE', *, *, #6451, .F. ) ;
#13358=CARTESIAN_POINT ( 'NONE',  ( -15.45084971874737256, 39.38125000068279746, -47.55282581475767500 ) ) ;
#13362=CARTESIAN_POINT ( 'NONE',  ( 9.631387414534489405E-15, 38.35937500034139447, 52.43083105670540789 ) ) ;
#13368=DIRECTION ( 'NONE',  ( 0.000000000000000000, 1.000000000000000000, 0.000000000000000000 ) ) ;
#13369=CARTESIAN_POINT ( 'NONE',  ( 50.00000000000000000, 41.00000000000000000, -6.123233995736766085E-15 ) ) ;
#13377=DIRECTION ( 'NONE',  ( -0.000000000000000000, 1.000000000000000000, -0.000000000000000000 ) ) ;
#13382=DIRECTION ( 'NONE',  ( 0.000000000000000000, 1.000000000000000000, 0.000000000000000000 ) ) ;
#13383=LINE ( 'NONE', #11159, #1018 ) ;
#13384=CARTESIAN_POINT ( 'NONE',  ( -7.919222016226934890, 32.44874571845316069, 49.99999999999996447 ) ) ;
#13386=CARTESIAN_POINT ( 'NONE',  ( -45.11452830843730766, 20.00000000000000711, 21.24066852005664430 ) ) ;
#13387=CARTESIAN_POINT ( 'NONE',  ( 9.631387414534489405E-15, 24.42187500034139447, 52.43083105670540789 ) ) ;
#13390=CARTESIAN_POINT ( 'NONE',  ( 30.81806926056962936, 23.15937500034139873, -42.41743335407647209 ) ) ;
#13399=CARTESIAN_POINT ( 'NONE',  ( 40.45084971874737079, 35.20000000000000284, -29.38926261462366440 ) ) ;
#13401=CARTESIAN_POINT ( 'NONE',  ( 30.81806926056964002, 32.62187500034140442, 42.41743335407647209 ) ) ;
#13402=CARTESIAN_POINT ( 'NONE',  ( -49.86468353125000164, 29.85937500034139802, 0.000000000000000000 ) ) ;
#13404=CARTESIAN_POINT ( 'NONE',  ( -8.660254037844387298, 28.00000000000000355, 5.000000000000000000 ) ) ;
#13405=CARTESIAN_POINT ( 'NONE',  ( -30.81806926056962226, 44.15937500034139163, 42.41743335407647919 ) ) ;
#13409=CARTESIAN_POINT ( 'NONE',  ( 49.86468353125001585, 22.82187500034138949, 16.20201782572375038 ) ) ;
#13412=ADVANCED_FACE ( 'NONE', ( #8237 ), #14618, .F. ) ;
#13414=ORIENTED_EDGE ( 'NONE', *, *, #5294, .F. ) ;
#13417=EDGE_LOOP ( 'NONE', ( #1292, #6317, #7644, #9972 ) ) ;
#13425=CARTESIAN_POINT ( 'NONE',  ( -49.86468353125000164, 49.92187500034140157, 0.000000000000000000 ) ) ;
#13431=CARTESIAN_POINT ( 'NONE',  ( -40.45084971874737789, 37.79999999999999716, -29.38926261462365730 ) ) ;
#13432=CARTESIAN_POINT ( 'NONE',  ( 9.631387414534489405E-15, 38.42187500034139447, 52.43083105670540789 ) ) ;
#13440=VERTEX_POINT ( 'NONE', #2924 ) ;
#13444=CARTESIAN_POINT ( 'NONE',  ( -30.90169943749473447, 22.08125000068279320, 42.53254041760200721 ) ) ;
#13445=CYLINDRICAL_SURFACE ( 'NONE', #10595, 50.00000000000000000 ) ;
#13446=CARTESIAN_POINT ( 'NONE',  ( 15.40903463028482356, 38.45937500034139589, 47.42413220539093999 ) ) ;
#13448=CARTESIAN_POINT ( 'NONE',  ( 49.86468353124999453, 46.95937500034139589, -16.20201782572376104 ) ) ;
#13454=CARTESIAN_POINT ( 'NONE',  ( -49.99999999999999289, 35.88125000068279746, 16.24598481164533226 ) ) ;
#13462=EDGE_LOOP ( 'NONE', ( #4025, #4506, #1438, #14692 ) ) ;
#13465=CARTESIAN_POINT ( 'NONE',  ( 15.45084971874737789, 28.60000000000000142, 47.55282581475767500 ) ) ;
#13473=CARTESIAN_POINT ( 'NONE',  ( -30.90169943749474513, 31.70000000000000639, -42.53254041760200721 ) ) ;
#13475=CARTESIAN_POINT ( 'NONE',  ( -45.54143403682493840, 20.00000000000001066, 20.30922080093765203 ) ) ;
#13476=CARTESIAN_POINT ( 'NONE',  ( -30.81806926056963292, 25.62187500034139731, -42.41743335407646498 ) ) ;
#13479=CARTESIAN_POINT ( 'NONE',  ( -15.40903463028480580, 24.25937500034139660, 47.42413220539094709 ) ) ;
#13487=CARTESIAN_POINT ( 'NONE',  ( 50.00000000000000711, 28.68125000068279462, 16.24598481164530739 ) ) ;
#13489=CARTESIAN_POINT ( 'NONE',  ( 15.40903463028481113, 29.32187500034139660, -47.42413220539094709 ) ) ;
#13490=CARTESIAN_POINT ( 'NONE',  ( -30.81806926056963292, 31.55937500034139376, -42.41743335407646498 ) ) ;
#13493=DIRECTION ( 'NONE',  ( 0.000000000000000000, 0.000000000000000000, 1.000000000000000000 ) ) ;
#13494=CARTESIAN_POINT ( 'NONE',  ( -15.40903463028481646, 47.45937500034139589, -47.42413220539093999 ) ) ;
#13497=CARTESIAN_POINT ( 'NONE',  ( -49.86468353124999453, 23.82187500034139305, -16.20201782572375393 ) ) ;
#13498=ORIENTED_EDGE ( 'NONE', *, *, #2914, .T. ) ;
#13504=CARTESIAN_POINT ( 'NONE',  ( 40.45084971874737079, 40.98125000068279888, -29.38926261462366440 ) ) ;
#13506=CARTESIAN_POINT ( 'NONE',  ( 40.34137639590981905, 46.72187500034139873, 29.30972558990010768 ) ) ;
#13510=CARTESIAN_POINT ( 'NONE',  ( -30.90169943749473802, 34.08125000068279320, 42.53254041760200721 ) ) ;
#13513=CARTESIAN_POINT ( 'NONE',  ( 15.40903463028481113, 41.32187500034140015, -47.42413220539094709 ) ) ;
#13518=EDGE_CURVE ( 'NONE', #9791, #13440, #13565, .T. ) ;
#13523=CARTESIAN_POINT ( 'NONE',  ( -40.45084971874737789, 39.58125000068280031, -29.38926261462365730 ) ) ;
#13525=ADVANCED_FACE ( 'NONE', ( #6160 ), #9742, .F. ) ;
#13526=CARTESIAN_POINT ( 'NONE',  ( 7.919222016226809657, 27.44874571845315003, -50.00000000000000000 ) ) ;
#13527=DIRECTION ( 'NONE',  ( 0.000000000000000000, 0.000000000000000000, 1.000000000000000000 ) ) ;
#13529=CARTESIAN_POINT ( 'NONE',  ( 40.34137639590981905, 38.65937500034139873, 29.30972558990010768 ) ) ;
#13531=CARTESIAN_POINT ( 'NONE',  ( 49.99999999999999289, 25.10000000000000142, -16.24598481164532160 ) ) ;
#13535=CARTESIAN_POINT ( 'NONE',  ( -3.111920190527341144E-15, 45.50000000000000000, -50.00000000000000000 ) ) ;
#13540=ORIENTED_EDGE ( 'NONE', *, *, #6349, .F. ) ;
#13545=EDGE_CURVE ( 'NONE', #10216, #13275, #434, .T. ) ;
#13546=ORIENTED_EDGE ( 'NONE', *, *, #12231, .T. ) ;
#13547=CARTESIAN_POINT ( 'NONE',  ( -49.99999999999999289, 47.68125000068280173, -16.24598481164531449 ) ) ;
#13550=FACE_OUTER_BOUND ( 'NONE', #2498, .T. ) ;
#13554=CARTESIAN_POINT ( 'NONE',  ( -40.45084971874737079, 45.98125000068279888, 29.38926261462367151 ) ) ;
#13557=CARTESIAN_POINT ( 'NONE',  ( -15.40903463028480580, 28.25937500034139660, 47.42413220539094709 ) ) ;
#13558=CARTESIAN_POINT ( 'NONE',  ( -49.99999999999999289, 29.89999999999999858, -16.24598481164531449 ) ) ;
#13559=ORIENTED_EDGE ( 'NONE', *, *, #12093, .T. ) ;
#13560=CARTESIAN_POINT ( 'NONE',  ( 30.90169943749473802, 45.29999999999999005, -42.53254041760200721 ) ) ;
#13562=VERTEX_POINT ( 'NONE', #8399 ) ;
#13565=B_SPLINE_CURVE_WITH_KNOTS ( 'NONE', 3,
 ( #7165, #7326, #14872, #3501, #7242, #903, #4582, #9900, #12397, #2324, #988, #1069, #2235, #5833, #9821, #8554, #4669, #12477, #13625, #2404, #12225, #6088, #5917, #4927, #5998, #10977, #7408, #4764 ),
 .UNSPECIFIED., .F., .F.,
 ( 4, 2, 2, 2, 2, 2, 2, 2, 2, 2, 2, 2, 2, 4 ),
 ( 0.09705106074666051963, 0.09878860373063949596, 0.1005261467146184723, 0.1040012326825764527, 0.1057387756665554429, 0.1074763186505344331, 0.1092138616345134233, 0.1109514046184924135, 0.1144264905864503939, 0.1161640335704293980, 0.1179015765544083882, 0.1213766625223663825, 0.1231142055063453866, 0.1248517484903243768 ),
 .UNSPECIFIED. ) ;
#13570=CARTESIAN_POINT ( 'NONE',  ( 30.81806926056962936, 29.22187500034139873, -42.41743335407647209 ) ) ;
#13571=CARTESIAN_POINT ( 'NONE',  ( -40.34137639590981905, 29.65937500034139518, -29.30972558990011478 ) ) ;
#13572=CARTESIAN_POINT ( 'NONE',  ( -49.99999999999999289, 36.10000000000000142, 16.24598481164533226 ) ) ;
#13575=CARTESIAN_POINT ( 'NONE',  ( -40.34137639590981195, 46.05937500034139731, 29.30972558990012189 ) ) ;
#13577=CARTESIAN_POINT ( 'NONE',  ( -30.81806926056962226, 24.22187500034139163, 42.41743335407647919 ) ) ;
#13585=CARTESIAN_POINT ( 'NONE',  ( -30.81806926056962226, 48.22187500034139163, 42.41743335407647919 ) ) ;
#13591=CARTESIAN_POINT ( 'NONE',  ( -40.45084971874737079, 35.98125000068279888, 29.38926261462367151 ) ) ;
#13592=CARTESIAN_POINT ( 'NONE',  ( 15.40903463028481113, 39.32187500034140015, -47.42413220539094709 ) ) ;
#13596=ORIENTED_EDGE ( 'NONE', *, *, #1414, .T. ) ;
#13600=EDGE_CURVE ( 'NONE', #13993, #2741, #15635, .T. ) ;
#13603=CARTESIAN_POINT ( 'NONE',  ( -2.547328955960238000E-13, 22.49999999999999645, 49.99999999999999289 ) ) ;
#13605=CARTESIAN_POINT ( 'NONE',  ( -15.40903463028480580, 40.25937500034139305, 47.42413220539094709 ) ) ;
#13606=CARTESIAN_POINT ( 'NONE',  ( -30.81806926056962226, 48.15937500034139873, 42.41743335407647209 ) ) ;
#13608=CARTESIAN_POINT ( 'NONE',  ( -49.86468353125000164, 49.92187500034140157, 0.000000000000000000 ) ) ;
#13612=CARTESIAN_POINT ( 'NONE',  ( -30.90169943749473447, 42.30000000000000426, 42.53254041760200721 ) ) ;
#13621=LINE ( 'NONE', #823, #12610 ) ;
#13623=CARTESIAN_POINT ( 'NONE',  ( -30.90169943749474513, 47.48125000068279888, -42.53254041760200721 ) ) ;
#13625=CARTESIAN_POINT ( 'NONE',  ( -8.844878598238441469, 7.388641928553207450, 98.30140974211549576 ) ) ;
#13632=CARTESIAN_POINT ( 'NONE',  ( -40.45084971874737079, 43.98125000068279888, 29.38926261462367151 ) ) ;
#13635=CARTESIAN_POINT ( 'NONE',  ( 49.86468353125001585, 20.75937500034140015, 16.20201782572375038 ) ) ;
#13636=CARTESIAN_POINT ( 'NONE',  ( -7.919222016226752814, 41.33250428222964246, -50.00000000000000711 ) ) ;
#13640=CARTESIAN_POINT ( 'NONE',  ( 49.99999999999999289, 45.10000000000000142, -16.24598481164532160 ) ) ;
#13642=CARTESIAN_POINT ( 'NONE',  ( 8.446640517145639571E-15, 48.49999999999999289, 50.00000000000000000 ) ) ;
#13646=ADVANCED_FACE ( 'NONE', ( #8978 ), #961, .F. ) ;
#13647=CARTESIAN_POINT ( 'NONE',  ( 7.919222016226809657, 29.22999571913594963, -50.00000000000000000 ) ) ;
#13651=CARTESIAN_POINT ( 'NONE',  ( 40.34137639590981905, 24.72187500034139873, 29.30972558990010768 ) ) ;
#13652=CARTESIAN_POINT ( 'NONE',  ( -3.210462471511496205E-15, 27.35937500034139447, -52.43083105670540789 ) ) ;
#13653=CARTESIAN_POINT ( 'NONE',  ( 0.000000000000000000, 22.50000000000000000, 102.0000000000000142 ) ) ;
#13654=CARTESIAN_POINT ( 'NONE',  ( -49.86468353124999453, 34.02187500034140299, 16.20201782572377169 ) ) ;
#13656=CARTESIAN_POINT ( 'NONE',  ( 30.81806926056964002, 42.55937500034139020, 42.41743335407647209 ) ) ;
#13658=CARTESIAN_POINT ( 'NONE',  ( -30.90169943749473802, 44.30000000000001137, 42.53254041760200721 ) ) ;
#13668=CARTESIAN_POINT ( 'NONE',  ( -15.40903463028480580, 48.32187500034140015, 47.42413220539094709 ) ) ;
#13673=CARTESIAN_POINT ( 'NONE',  ( 15.45084971874736723, 31.18125000068279817, -47.55282581475768211 ) ) ;
#13674=CARTESIAN_POINT ( 'NONE',  ( 49.86468353125000164, 34.92187500034140157, -6.106662507704105588E-15 ) ) ;
#13675=CARTESIAN_POINT ( 'NONE',  ( 0.000000000000000000, 45.07596123493892293, 92.05189185291139609 ) ) ;
#13683=CARTESIAN_POINT ( 'NONE',  ( 6.123233995736766085E-15, 50.00000000000000000, -50.00000000000000000 ) ) ;
#13685=CARTESIAN_POINT ( 'NONE',  ( 0.000000000000000000, 20.00000000000000355, 0.000000000000000000 ) ) ;
#13686=CARTESIAN_POINT ( 'NONE',  ( -30.81806926056962226, 40.15937500034139163, 42.41743335407647919 ) ) ;
#13687=CARTESIAN_POINT ( 'NONE',  ( -49.86468353124999453, 43.95937500034138878, 16.20201782572377169 ) ) ;
#13693=CARTESIAN_POINT ( 'NONE',  ( 17.50000000000000000, 22.50000000000000355, 102.0000000000000142 ) ) ;
#13694=CARTESIAN_POINT ( 'NONE',  ( 50.00000000000000711, 40.89999999999999858, 16.24598481164530739 ) ) ;
#13696=VERTEX_POINT ( 'NONE', #14438 ) ;
#13699=ORIENTED_EDGE ( 'NONE', *, *, #2766, .T. ) ;
#13706=CIRCLE ( 'NONE', #5514, 100.0000000000000000 ) ;
#13712=EDGE_CURVE ( 'NONE', #10597, #12892, #10473, .T. ) ;
#13714=DIRECTION ( 'NONE',  ( -0.000000000000000000, 1.000000000000000000, -0.000000000000000000 ) ) ;
#13716=CARTESIAN_POINT ( 'NONE',  ( 50.00000000000000000, 46.78125000068279604, -6.123233995736766085E-15 ) ) ;
#13718=AXIS2_PLACEMENT_3D ( 'NONE', #9558, #6909, #15946 ) ;
#13724=EDGE_CURVE ( 'NONE', #9639, #1788, #13049, .T. ) ;
#13730=CARTESIAN_POINT ( 'NONE',  ( 15.45084971874736723, 49.39999999999999858, -47.55282581475768211 ) ) ;
#13737=CARTESIAN_POINT ( 'NONE',  ( -30.81806926056962226, 20.22187500034139163, 42.41743335407647919 ) ) ;
#13738=CARTESIAN_POINT ( 'NONE',  ( 30.81806926056964002, 30.55937500034139731, 42.41743335407646498 ) ) ;
#13740=CARTESIAN_POINT ( 'NONE',  ( -15.40903463028480580, 32.32187500034139305, 47.42413220539094709 ) ) ;
#13741=DIRECTION ( 'NONE',  ( -0.000000000000000000, 1.000000000000000000, -0.000000000000000000 ) ) ;
#13742=CARTESIAN_POINT ( 'NONE',  ( 49.99999999999999289, 39.10000000000000853, -16.24598481164532160 ) ) ;
#13743=CARTESIAN_POINT ( 'NONE',  ( -15.40903463028481646, 41.45937500034140299, -47.42413220539093999 ) ) ;
#13745=CARTESIAN_POINT ( 'NONE',  ( 15.45084971874737789, 42.60000000000000142, 47.55282581475767500 ) ) ;
#13753=CIRCLE ( 'NONE', #3418, 50.00000000000000000 ) ;
#13754=CARTESIAN_POINT ( 'NONE',  ( -49.86468353125000164, 43.92187500034140157, 0.000000000000000000 ) ) ;
#13758=CARTESIAN_POINT ( 'NONE',  ( 49.99999999999999289, 24.88125000068279746, -16.24598481164532160 ) ) ;
#13759=CARTESIAN_POINT ( 'NONE',  ( 30.81806926056962936, 37.22187500034139873, -42.41743335407647209 ) ) ;
#13763=EDGE_LOOP ( 'NONE', ( #12316, #16359, #10485 ) ) ;
#13764=ORIENTED_EDGE ( 'NONE', *, *, #3788, .T. ) ;
#13770=CARTESIAN_POINT ( 'NONE',  ( -50.00000000000000000, 23.78125000068279959, 0.000000000000000000 ) ) ;
#13771=CARTESIAN_POINT ( 'NONE',  ( -30.81806926056962226, 34.15937500034139163, 42.41743335407647919 ) ) ;
#13772=CARTESIAN_POINT ( 'NONE',  ( -49.86468353124999453, 41.75937500034139305, -16.20201782572375393 ) ) ;
#13775=CARTESIAN_POINT ( 'NONE',  ( 0.000000000000000000, 28.00000000000000355, 0.000000000000000000 ) ) ;
#13783=( BOUNDED_CURVE ( )  B_SPLINE_CURVE ( 2, ( #11856, #4302, #9366, #10695, #458, #12014, #6961, #10622, #6043, #14657, #15999, #781, #5873 ),
 .UNSPECIFIED., .F., .T. ) 
 B_SPLINE_CURVE_WITH_KNOTS ( ( 3, 2, 2, 2, 2, 2, 3 ),
 ( 0.5166666666666667185, 0.5200000000000000178, 0.5266666666666666163, 0.5333333333333333259, 0.5400000000000000355, 0.5466666666666666341, 0.5500000000000000444 ),
 .UNSPECIFIED. ) 
 CURVE ( )  GEOMETRIC_REPRESENTATION_ITEM ( )  RATIONAL_B_SPLINE_CURVE ( ( 0.9755282581475768211, 0.9755282581475771542, 1.000000000000000000, 0.9510565162951535312, 1.000000000000000000, 0.9510565162951535312, 1.000000000000000000, 0.9510565162951535312, 1.000000000000000000, 0.9510565162951535312, 1.000000000000000000, 0.9755282581475763770, 0.9755282581475768211 ) ) 
 REPRESENTATION_ITEM ( '' )  );
#13795=( LENGTH_UNIT ( ) NAMED_UNIT ( * ) SI_UNIT ( .MILLI., .METRE. ) );
#13797=CARTESIAN_POINT ( 'NONE',  ( 30.90169943749475578, 48.48125000068279888, 42.53254041760200010 ) ) ;
#13798=CARTESIAN_POINT ( 'NONE',  ( 7.919222016226940219, 21.44874571845316069, -49.99999999999996447 ) ) ;
#13805=EDGE_LOOP ( 'NONE', ( #7401, #1895, #4814, #3319 ) ) ;
#13810=DIRECTION ( 'NONE',  ( 0.000000000000000000, 0.000000000000000000, 1.000000000000000000 ) ) ;
#13814=CARTESIAN_POINT ( 'NONE',  ( 30.81806926056962936, 23.22187500034139163, -42.41743335407647209 ) ) ;
#13815=CARTESIAN_POINT ( 'NONE',  ( -15.40903463028481646, 25.45937500034139589, -47.42413220539093999 ) ) ;
#13817=CARTESIAN_POINT ( 'NONE',  ( 9.631387414534489405E-15, 38.42187500034139447, 52.43083105670540789 ) ) ;
#13818=FACE_OUTER_BOUND ( 'NONE', #7802, .T. ) ;
#13819=CARTESIAN_POINT ( 'NONE',  ( -3.219174618344376363E-15, 35.50000000000000000, -52.57311121191334990 ) ) ;
#13820=CARTESIAN_POINT ( 'NONE',  ( -40.34137639590981905, 39.65937500034139873, -29.30972558990011478 ) ) ;
#13822=CARTESIAN_POINT ( 'NONE',  ( 15.45084971874736723, 47.40000000000000568, -47.55282581475768211 ) ) ;
#13829=CARTESIAN_POINT ( 'NONE',  ( 6.123233995736766085E-15, 20.00000000000000355, -50.00000000000000000 ) ) ;
#13832=CARTESIAN_POINT ( 'NONE',  ( 40.34137639590981195, 45.12187500034139731, -29.30972558990011834 ) ) ;
#13836=CARTESIAN_POINT ( 'NONE',  ( -30.90169943749474868, 27.48125000068279888, -42.53254041760200721 ) ) ;
#13837=CARTESIAN_POINT ( 'NONE',  ( -30.90169943749474513, 45.70000000000000284, -42.53254041760200721 ) ) ;
#13838=CARTESIAN_POINT ( 'NONE',  ( -15.40903463028480580, 32.32187500034139305, 47.42413220539094709 ) ) ;
#13842=ORIENTED_EDGE ( 'NONE', *, *, #5410, .F. ) ;
#13843=VERTEX_POINT ( 'NONE', #886 ) ;
#13849=CARTESIAN_POINT ( 'NONE',  ( 30.81806926056962936, 29.15937500034139518, -42.41743335407647209 ) ) ;
#13852=CARTESIAN_POINT ( 'NONE',  ( -15.40903463028480580, 44.32187500034140015, 47.42413220539094709 ) ) ;
#13858=AXIS2_PLACEMENT_3D ( 'NONE', #8384, #9561, #735 ) ;
#13868=CARTESIAN_POINT ( 'NONE',  ( -40.34137639590981905, 49.65937500034139873, -29.30972558990011478 ) ) ;
#13874=FILL_AREA_STYLE ('',( #5173 ) ) ;
#13875=CARTESIAN_POINT ( 'NONE',  ( -3.219174618344376363E-15, 45.28125000068279604, -52.57311121191334990 ) ) ;
#13876=CARTESIAN_POINT ( 'NONE',  ( 40.45084971874737079, 44.98125000068279888, -29.38926261462366440 ) ) ;
#13886=CARTESIAN_POINT ( 'NONE',  ( 7.919222016226940219, 33.44874571845316069, -49.99999999999996447 ) ) ;
#13890=LINE ( 'NONE', #6513, #11850 ) ;
#13891=CARTESIAN_POINT ( 'NONE',  ( 49.86468353125001585, 22.82187500034138949, 16.20201782572375038 ) ) ;
#13892=CARTESIAN_POINT ( 'NONE',  ( 9.631387414534489405E-15, 20.35937500034139092, 52.43083105670540789 ) ) ;
#13894=CARTESIAN_POINT ( 'NONE',  ( 30.81806926056964002, 34.62187500034139731, 42.41743335407646498 ) ) ;
#13897=CARTESIAN_POINT ( 'NONE',  ( 50.00000000000000711, 32.89999999999999147, 16.24598481164530739 ) ) ;
#13898=CARTESIAN_POINT ( 'NONE',  ( -49.86468353124999453, 37.75937500034140015, -16.20201782572375393 ) ) ;
#13900=CARTESIAN_POINT ( 'NONE',  ( 50.00000000000000711, 44.90000000000000568, 16.24598481164530739 ) ) ;
#13902=ORIENTED_EDGE ( 'NONE', *, *, #1732, .F. ) ;
#13905=ORIENTED_EDGE ( 'NONE', *, *, #2766, .F. ) ;
#13912=CARTESIAN_POINT ( 'NONE',  ( 9.631387414534489405E-15, 42.42187500034140157, 52.43083105670540789 ) ) ;
#13916=CARTESIAN_POINT ( 'NONE',  ( 30.90169943749474157, 29.08125000068280031, -42.53254041760200721 ) ) ;
#13918=CARTESIAN_POINT ( 'NONE',  ( -49.86468353124999453, 35.82187500034139305, -16.20201782572375393 ) ) ;
#13930=CARTESIAN_POINT ( 'NONE',  ( -49.99999999999999289, 23.68125000068279462, -16.24598481164531449 ) ) ;
#13931=CARTESIAN_POINT ( 'NONE',  ( -15.40903463028481646, 29.45937500034139589, -47.42413220539093999 ) ) ;
#13932=CARTESIAN_POINT ( 'NONE',  ( 40.34137639590981195, 43.12187500034139731, -29.30972558990011834 ) ) ;
#13941=CARTESIAN_POINT ( 'NONE',  ( -7.919222016226822092, 46.22999571913594963, 50.00000000000000000 ) ) ;
#13948=DIRECTION ( 'NONE',  ( 0.000000000000000000, 0.000000000000000000, 1.000000000000000000 ) ) ;
#13949=CARTESIAN_POINT ( 'NONE',  ( -40.34137639590981195, 48.05937500034139731, 29.30972558990012189 ) ) ;
#13958=CARTESIAN_POINT ( 'NONE',  ( 15.45084971874736723, 39.18125000068280173, -47.55282581475768211 ) ) ;
#13962=CARTESIAN_POINT ( 'NONE',  ( -40.34137639590981195, 22.05937500034139731, 29.30972558990012189 ) ) ;
#13969=DIRECTION ( 'NONE',  ( -0.000000000000000000, -0.000000000000000000, -1.000000000000000000 ) ) ;
#13974=CARTESIAN_POINT ( 'NONE',  ( -3.991010794631277836, 39.54842293358396432, 92.94258460798921817 ) ) ;
#13979=CARTESIAN_POINT ( 'NONE',  ( 49.86468353124999453, 22.95937500034139589, -16.20201782572376104 ) ) ;
#13981=CARTESIAN_POINT ( 'NONE',  ( 49.86468353124999453, 37.02187500034138878, -16.20201782572376104 ) ) ;
#13984=CARTESIAN_POINT ( 'NONE',  ( -3.219174618344376363E-15, 31.50000000000000000, -52.57311121191334990 ) ) ;
#13985=CARTESIAN_POINT ( 'NONE',  ( -49.86468353125000164, 41.85937500034139447, 0.000000000000000000 ) ) ;
#13987=CARTESIAN_POINT ( 'NONE',  ( -3.219174618344376363E-15, 45.49999999999999289, -52.57311121191334990 ) ) ;
#13993=VERTEX_POINT ( 'NONE', #4652 ) ;
#14000=CARTESIAN_POINT ( 'NONE',  ( 15.40903463028481113, 43.32187500034139305, -47.42413220539094709 ) ) ;
#14003=CARTESIAN_POINT ( 'NONE',  ( -30.90169943749473802, 28.08125000068280031, 42.53254041760200721 ) ) ;
#14005=CARTESIAN_POINT ( 'NONE',  ( 30.81806926056962936, 31.22187500034139873, -42.41743335407647209 ) ) ;
#14006=CARTESIAN_POINT ( 'NONE',  ( -30.90169943749473447, 28.29999999999999716, 42.53254041760200721 ) ) ;
#14009=EDGE_LOOP ( 'NONE', ( #10287, #9853, #7667, #12871 ) ) ;
#14014=CARTESIAN_POINT ( 'NONE',  ( -49.86468353125000164, 31.85937500034139447, 0.000000000000000000 ) ) ;
#14017=EDGE_CURVE ( 'NONE', #9639, #2321, #16360, .T. ) ;
#14018=CARTESIAN_POINT ( 'NONE',  ( -3.210462471511496205E-15, 45.42187500034138736, -52.43083105670540789 ) ) ;
#14020=LINE ( 'NONE', #2637, #15759 ) ;
#14025=EDGE_LOOP ( 'NONE', ( #4218, #16015, #7702, #14887, #10796 ) ) ;
#14026=( BOUNDED_CURVE ( )  B_SPLINE_CURVE ( 2, ( #15761, #14425, #3045, #12021, #5717, #6811, #8118, #16009, #15682, #10788, #8283, #13351, #12104 ),
 .UNSPECIFIED., .F., .F. ) 
 B_SPLINE_CURVE_WITH_KNOTS ( ( 3, 2, 2, 2, 2, 2, 3 ),
 ( 0.6166666666666666963, 0.6199999999999999956, 0.6266666666666667052, 0.6333333333333333037, 0.6400000000000000133, 0.6466666666666666119, 0.6500000000000000222 ),
 .UNSPECIFIED. ) 
 CURVE ( )  GEOMETRIC_REPRESENTATION_ITEM ( )  RATIONAL_B_SPLINE_CURVE ( ( 0.9755282581475768211, 0.9755282581475771542, 1.000000000000000000, 0.9510565162951535312, 1.000000000000000000, 0.9510565162951535312, 1.000000000000000000, 0.9510565162951535312, 1.000000000000000000, 0.9510565162951535312, 1.000000000000000000, 0.9755282581475763770, 0.9755282581475768211 ) ) 
 REPRESENTATION_ITEM ( '' )  );
#14032=ADVANCED_FACE ( 'NONE', ( #7334 ), #4288, .F. ) ;
#14037=CARTESIAN_POINT ( 'NONE',  ( -2.547328955960238000E-13, 32.28125000068278894, 49.99999999999999289 ) ) ;
#14042=CARTESIAN_POINT ( 'NONE',  ( 40.45084971874737079, 38.98125000068279888, -29.38926261462366440 ) ) ;
#14044=EDGE_CURVE ( 'NONE', #6639, #6101, #14120, .T. ) ;
#14047=VERTEX_POINT ( 'NONE', #15128 ) ;
#14055=ORIENTED_EDGE ( 'NONE', *, *, #13724, .F. ) ;
#14056=CARTESIAN_POINT ( 'NONE',  ( 40.45084971874737789, 32.80000000000000426, 29.38926261462365375 ) ) ;
#14061=CARTESIAN_POINT ( 'NONE',  ( 49.86468353125000164, 24.85937500034139802, -6.106662507704105588E-15 ) ) ;
#14063=CARTESIAN_POINT ( 'NONE',  ( 49.86468353125001585, 30.82187500034139660, 16.20201782572375038 ) ) ;
#14065=CARTESIAN_POINT ( 'NONE',  ( 9.657523855033129090E-15, 30.50000000000000000, 52.57311121191334990 ) ) ;
#14066=CARTESIAN_POINT ( 'NONE',  ( -49.86468353124999453, 29.95937500034139944, 16.20201782572377525 ) ) ;
#14068=CARTESIAN_POINT ( 'NONE',  ( -15.45084971874737256, 41.60000000000000142, -47.55282581475767500 ) ) ;
#14079=CARTESIAN_POINT ( 'NONE',  ( -49.86468353124999453, 40.02187500034140299, 16.20201782572377525 ) ) ;
#14080=CARTESIAN_POINT ( 'NONE',  ( -3.210462471511496205E-15, 41.35937500034138736, -52.43083105670540789 ) ) ;
#14083=CARTESIAN_POINT ( 'NONE',  ( -15.45084971874737256, 25.38125000068279746, -47.55282581475767500 ) ) ;
#14084=CARTESIAN_POINT ( 'NONE',  ( 16.92534237191551938, 26.98475202694456598, 93.72602301361716570 ) ) ;
#14085=CARTESIAN_POINT ( 'NONE',  ( 40.34137639590981905, 30.72187500034139518, 29.30972558990010768 ) ) ;
#14096=CARTESIAN_POINT ( 'NONE',  ( -15.40903463028480580, 32.25937500034140015, 47.42413220539094709 ) ) ;
#14098=CARTESIAN_POINT ( 'NONE',  ( 49.86468353125000164, 44.92187500034140157, -6.106662507704105588E-15 ) ) ;
#14102=CARTESIAN_POINT ( 'NONE',  ( 0.000000000000000000, 50.00000000000000000, 0.000000000000000000 ) ) ;
#14113=CARTESIAN_POINT ( 'NONE',  ( -30.90169943749474868, 25.69999999999999929, -42.53254041760200721 ) ) ;
#14119=CARTESIAN_POINT ( 'NONE',  ( -30.90169943749474868, 43.48125000068279178, -42.53254041760200721 ) ) ;
#14120=( BOUNDED_CURVE ( )  B_SPLINE_CURVE ( 2, ( #7658, #7599, #4854, #998, #9911, #7337, #12487, #3679, #8900, #6171, #1080, #11168, #7571 ),
 .UNSPECIFIED., .F., .F. ) 
 B_SPLINE_CURVE_WITH_KNOTS ( ( 3, 2, 2, 2, 2, 2, 3 ),
 ( 0.7833333333333333259, 0.7866666666666666252, 0.7933333333333333348, 0.8000000000000000444, 0.8066666666666666430, 0.8133333333333333526, 0.8166666666666666519 ),
 .UNSPECIFIED. ) 
 CURVE ( )  GEOMETRIC_REPRESENTATION_ITEM ( )  RATIONAL_B_SPLINE_CURVE ( ( 0.9755282581475768211, 0.9755282581475768211, 1.000000000000000000, 0.9510565162951535312, 1.000000000000000000, 0.9510565162951535312, 1.000000000000000000, 0.9510565162951535312, 1.000000000000000000, 0.9510565162951535312, 1.000000000000000000, 0.9755282581475768211, 0.9755282581475768211 ) ) 
 REPRESENTATION_ITEM ( '' )  );
#14132=ORIENTED_EDGE ( 'NONE', *, *, #6844, .T. ) ;
#14133=EDGE_CURVE ( 'NONE', #16188, #14909, #14292, .T. ) ;
#14140=CARTESIAN_POINT ( 'NONE',  ( -49.86468353124999453, 21.95937500034139234, 16.20201782572377169 ) ) ;
#14141=PLANE ( 'NONE',  #1230 ) ;
#14142=CARTESIAN_POINT ( 'NONE',  ( 40.34137639590981905, 30.72187500034139518, 29.30972558990010768 ) ) ;
#14145=CARTESIAN_POINT ( 'NONE',  ( -49.99999999999999289, 28.10000000000000497, 16.24598481164533226 ) ) ;
#14146=CARTESIAN_POINT ( 'NONE',  ( -15.40903463028480580, 34.25937500034139305, 47.42413220539094709 ) ) ;
#14157=CARTESIAN_POINT ( 'NONE',  ( 0.000000000000000000, 50.00000000000000000, 0.000000000000000000 ) ) ;
#14159=CONICAL_SURFACE ( 'NONE', #8581, 100.0000000000000000, 0.1745329251994333364 ) ;
#14160=LINE ( 'NONE', #12515, #4143 ) ;
#14161=CARTESIAN_POINT ( 'NONE',  ( -15.40903463028480580, 36.32187500034140015, 47.42413220539094709 ) ) ;
#14162=CARTESIAN_POINT ( 'NONE',  ( 15.40903463028481113, 39.25937500034140015, -47.42413220539094709 ) ) ;
#14165=CARTESIAN_POINT ( 'NONE',  ( -40.45084971874737079, 19.98125000068279888, 29.38926261462367151 ) ) ;
#14166=CARTESIAN_POINT ( 'NONE',  ( 16.59466974644969994, 28.08544099924165494, 93.58803292011415920 ) ) ;
#14167=CARTESIAN_POINT ( 'NONE',  ( 30.81806926056964002, 28.62187500034140086, 42.41743335407647209 ) ) ;
#14168=CARTESIAN_POINT ( 'NONE',  ( 8.446640517145639571E-15, 28.49999999999999645, 50.00000000000000000 ) ) ;
#14172=CARTESIAN_POINT ( 'NONE',  ( 15.45084971874736723, 49.18125000068279462, -47.55282581475768211 ) ) ;
#14178=CARTESIAN_POINT ( 'NONE',  ( -15.40903463028481646, 27.45937500034139944, -47.42413220539093999 ) ) ;
#14181=CARTESIAN_POINT ( 'NONE',  ( 49.86468353124999453, 45.02187500034138878, -16.20201782572376104 ) ) ;
#14184=CARTESIAN_POINT ( 'NONE',  ( 49.86468353125000164, 46.92187500034139447, -6.106662507704105588E-15 ) ) ;
#14194=CARTESIAN_POINT ( 'NONE',  ( 40.45084971874737789, 38.58125000068280031, 29.38926261462365375 ) ) ;
#14196=CARTESIAN_POINT ( 'NONE',  ( 40.45084971874737079, 23.20000000000000284, -29.38926261462366440 ) ) ;
#14197=CARTESIAN_POINT ( 'NONE',  ( -49.86468353124999453, 47.95937500034138878, 16.20201782572377525 ) ) ;
#14198=FACE_OUTER_BOUND ( 'NONE', #3072, .T. ) ;
#14200=CARTESIAN_POINT ( 'NONE',  ( -49.86468353125000164, 21.92187500034139802, 0.000000000000000000 ) ) ;
#14202=CARTESIAN_POINT ( 'NONE',  ( -30.90169943749474868, 37.48125000068279888, -42.53254041760200721 ) ) ;
#14204=CARTESIAN_POINT ( 'NONE',  ( 50.00000000000000000, 20.78125000068279959, -6.123233995736766085E-15 ) ) ;
#14209=CARTESIAN_POINT ( 'NONE',  ( 7.919222016226809657, 43.44874571845315359, -50.00000000000000000 ) ) ;
#14215=PLANE ( 'NONE',  #4417 ) ;
#14216=CARTESIAN_POINT ( 'NONE',  ( -10.68402110179033926, 36.37206659422378863, 92.97581280613414378 ) ) ;
#14220=CARTESIAN_POINT ( 'NONE',  ( -50.00000000000000000, 29.78125000068279959, 0.000000000000000000 ) ) ;
#14222=CARTESIAN_POINT ( 'NONE',  ( -48.20095974065431932, 20.00000000000001066, 12.77318064350212623 ) ) ;
#14223=CARTESIAN_POINT ( 'NONE',  ( -49.86468353124999453, 30.02187500034139234, 16.20201782572377169 ) ) ;
#14227=CARTESIAN_POINT ( 'NONE',  ( -15.45084971874736368, 28.40000000000000213, 47.55282581475768211 ) ) ;
#14228=CARTESIAN_POINT ( 'NONE',  ( 49.86468353125001585, 30.75937500034139305, 16.20201782572375038 ) ) ;
#14248=CARTESIAN_POINT ( 'NONE',  ( -40.34137639590981905, 33.72187500034139873, -29.30972558990011478 ) ) ;
#14249=CARTESIAN_POINT ( 'NONE',  ( 40.34137639590981195, 43.05937500034139731, -29.30972558990011834 ) ) ;
#14252=CARTESIAN_POINT ( 'NONE',  ( -50.00000000000000000, 19.78125000068279604, 0.000000000000000000 ) ) ;
#14254=CARTESIAN_POINT ( 'NONE',  ( -15.40903463028480580, 26.32187500034140015, 47.42413220539094709 ) ) ;
#14255=CIRCLE ( 'NONE', #7105, 50.00000000000000000 ) ;
#14260=CARTESIAN_POINT ( 'NONE',  ( 8.446640517145639571E-15, 48.28125000068279604, 50.00000000000000000 ) ) ;
#14264=CARTESIAN_POINT ( 'NONE',  ( 9.631387414534489405E-15, 24.35937500034139802, 52.43083105670540789 ) ) ;
#14265=DIRECTION ( 'NONE',  ( -0.000000000000000000, 1.000000000000000000, -0.000000000000000000 ) ) ;
#14266=CARTESIAN_POINT ( 'NONE',  ( 40.34137639590981905, 42.72187500034139873, 29.30972558990010768 ) ) ;
#14269=CARTESIAN_POINT ( 'NONE',  ( -30.81806926056962226, 46.22187500034139163, 42.41743335407647919 ) ) ;
#14275=ORIENTED_EDGE ( 'NONE', *, *, #11887, .T. ) ;
#14279=CARTESIAN_POINT ( 'NONE',  ( -15.45084971874737256, 43.38125000068279746, -47.55282581475767500 ) ) ;
#14282=CARTESIAN_POINT ( 'NONE',  ( -30.90169943749474868, 23.69999999999999929, -42.53254041760200721 ) ) ;
#14283=CARTESIAN_POINT ( 'NONE',  ( 30.81806926056964002, 42.55937500034139020, 42.41743335407647209 ) ) ;
#14289=CARTESIAN_POINT ( 'NONE',  ( -30.90169943749473802, 42.08125000068279320, 42.53254041760200721 ) ) ;
#14291=CARTESIAN_POINT ( 'NONE',  ( 15.45084971874737789, 22.38125000068280102, 47.55282581475767500 ) ) ;
#14292=LINE ( 'NONE', #74, #9214 ) ;
#14307=CARTESIAN_POINT ( 'NONE',  ( -2.547328955960238000E-13, 30.28125000068279604, 49.99999999999999289 ) ) ;
#14310=CARTESIAN_POINT ( 'NONE',  ( -46.44184698740843231, 20.00000000000000355, 18.15679736478566753 ) ) ;
#14311=CARTESIAN_POINT ( 'NONE',  ( -15.40903463028481646, 29.52187500034139589, -47.42413220539093999 ) ) ;
#14315=CARTESIAN_POINT ( 'NONE',  ( 15.40903463028482356, 32.45937500034138878, 47.42413220539093999 ) ) ;
#14323=( BOUNDED_CURVE ( )  B_SPLINE_CURVE ( 2, ( #2696, #12844, #4454, #4365, #9519, #8263, #10436, #10682, #14566, #9430, #14480, #3113, #7022 ),
 .UNSPECIFIED., .F., .F. ) 
 B_SPLINE_CURVE_WITH_KNOTS ( ( 3, 2, 2, 2, 2, 2, 3 ),
 ( 0.1833333333333333481, 0.1866666666666666752, 0.1933333333333333293, 0.2000000000000000111, 0.2066666666666666652, 0.2133333333333333470, 0.2166666666666666741 ),
 .UNSPECIFIED. ) 
 CURVE ( )  GEOMETRIC_REPRESENTATION_ITEM ( )  RATIONAL_B_SPLINE_CURVE ( ( 0.9755282581475767101, 0.9755282581475768211, 1.000000000000000000, 0.9510565162951535312, 1.000000000000000000, 0.9510565162951535312, 1.000000000000000000, 0.9510565162951535312, 1.000000000000000000, 0.9510565162951535312, 1.000000000000000000, 0.9755282581475768211, 0.9755282581475768211 ) ) 
 REPRESENTATION_ITEM ( '' )  );
#14328=CARTESIAN_POINT ( 'NONE',  ( 30.81806926056964002, 38.62187500034139731, 42.41743335407647209 ) ) ;
#14329=CARTESIAN_POINT ( 'NONE',  ( 30.81806926056964002, 36.55937500034139731, 42.41743335407646498 ) ) ;
#14332=CARTESIAN_POINT ( 'NONE',  ( 40.45084971874737789, 20.58125000068280031, 29.38926261462365375 ) ) ;
#14335=CARTESIAN_POINT ( 'NONE',  ( -40.34137639590981905, 29.72187500034139518, -29.30972558990011478 ) ) ;
#14346=CARTESIAN_POINT ( 'NONE',  ( -49.86468353124999453, 23.75937500034140015, -16.20201782572375393 ) ) ;
#14348=CARTESIAN_POINT ( 'NONE',  ( 30.81806926056962936, 39.22187500034139873, -42.41743335407646498 ) ) ;
#14351=CARTESIAN_POINT ( 'NONE',  ( -15.40903463028481646, 49.52187500034140299, -47.42413220539093999 ) ) ;
#14361=CARTESIAN_POINT ( 'NONE',  ( -3.219174618344376363E-15, 25.50000000000000355, -52.57311121191334990 ) ) ;
#14362=CARTESIAN_POINT ( 'NONE',  ( -15.40903463028481646, 41.45937500034140299, -47.42413220539093999 ) ) ;
#14363=CARTESIAN_POINT ( 'NONE',  ( -3.111920190527341144E-15, 25.28125000068279604, -50.00000000000000000 ) ) ;
#14367=CARTESIAN_POINT ( 'NONE',  ( 50.00000000000000711, 36.68125000068280173, 16.24598481164530739 ) ) ;
#14375=DIRECTION ( 'NONE',  ( 0.000000000000000000, 0.000000000000000000, 1.000000000000000000 ) ) ;
#14383=CARTESIAN_POINT ( 'NONE',  ( -30.90169943749474513, 37.48125000068279888, -42.53254041760200721 ) ) ;
#14384=CARTESIAN_POINT ( 'NONE',  ( 7.309249795462555710, 6.589106271932131165, 98.56897796993928296 ) ) ;
#14385=CARTESIAN_POINT ( 'NONE',  ( -48.33688377893763999, 20.00000000000000355, 12.24883938693908725 ) ) ;
#14386=CARTESIAN_POINT ( 'NONE',  ( -30.81806926056963292, 29.62187500034139376, -42.41743335407646498 ) ) ;
#14389=CARTESIAN_POINT ( 'NONE',  ( 15.40903463028481113, 35.25937500034139305, -47.42413220539094709 ) ) ;
#14391=VERTEX_POINT ( 'NONE', #640 ) ;
#14399=CARTESIAN_POINT ( 'NONE',  ( -15.40903463028481646, 37.52187500034139589, -47.42413220539093999 ) ) ;
#14400=CARTESIAN_POINT ( 'NONE',  ( 30.81806926056962936, 33.15937500034139873, -42.41743335407646498 ) ) ;
#14404=CARTESIAN_POINT ( 'NONE',  ( -30.90169943749474868, 23.48125000068279888, -42.53254041760200721 ) ) ;
#14406=CARTESIAN_POINT ( 'NONE',  ( 15.40903463028482356, 28.52187500034139589, 47.42413220539093999 ) ) ;
#14409=EDGE_LOOP ( 'NONE', ( #1272, #8697, #14758, #1896 ) ) ;
#14416=CARTESIAN_POINT ( 'NONE',  ( 2.600676159226420495E-13, 31.28125000068279604, -49.99999999999999289 ) ) ;
#14418=CARTESIAN_POINT ( 'NONE',  ( -3.210462471511496205E-15, 27.35937500034139802, -52.43083105670540789 ) ) ;
#14420=CARTESIAN_POINT ( 'NONE',  ( 49.86468353125000164, 40.92187500034139447, -6.106662507704105588E-15 ) ) ;
#14424=CARTESIAN_POINT ( 'NONE',  ( 49.86468353125001585, 44.82187500034138594, 16.20201782572375038 ) ) ;
#14425=CARTESIAN_POINT ( 'NONE',  ( 7.919222016226940219, 31.44874571845315714, -49.99999999999996447 ) ) ;
#14432=VECTOR ( 'NONE', #7480, 1000.000000000000000 ) ;
#14434=CARTESIAN_POINT ( 'NONE',  ( -40.45084971874737789, 23.80000000000000071, -29.38926261462365730 ) ) ;
#14435=CARTESIAN_POINT ( 'NONE',  ( -3.210462471511496205E-15, 43.35937500034138736, -52.43083105670540789 ) ) ;
#14436=CARTESIAN_POINT ( 'NONE',  ( 0.000000000000000000, 20.00000000000000355, 0.000000000000000000 ) ) ;
#14438=CARTESIAN_POINT ( 'NONE',  ( -3.111920190527341144E-15, 43.28125000068280315, -50.00000000000000000 ) ) ;
#14440=CARTESIAN_POINT ( 'NONE',  ( 9.657523855033129090E-15, 34.28125000068278894, 52.57311121191334990 ) ) ;
#14442=CARTESIAN_POINT ( 'NONE',  ( 2.600676159226420495E-13, 23.28125000068279604, -49.99999999999999289 ) ) ;
#14447=ORIENTED_EDGE ( 'NONE', *, *, #6349, .T. ) ;
#14453=DIRECTION ( 'NONE',  ( 0.000000000000000000, 0.000000000000000000, 1.000000000000000000 ) ) ;
#14457=CARTESIAN_POINT ( 'NONE',  ( -3.111920190527341144E-15, 29.28125000068279604, -50.00000000000000000 ) ) ;
#14458=CARTESIAN_POINT ( 'NONE',  ( 12.84309919097911923, 10.59908474996653460, 97.28791577635783483 ) ) ;
#14459=CARTESIAN_POINT ( 'NONE',  ( -47.18644234407105387, 20.00000000000000355, 16.12223069495573924 ) ) ;
#14460=CARTESIAN_POINT ( 'NONE',  ( 15.40903463028481113, 25.32187500034139660, -47.42413220539094709 ) ) ;
#14462=CARTESIAN_POINT ( 'NONE',  ( 9.631387414534489405E-15, 24.35937500034139802, 52.43083105670540789 ) ) ;
#14463=CARTESIAN_POINT ( 'NONE',  ( -1.240322475938754499E-13, 38.50000000000000711, 50.00000000000000000 ) ) ;
#14467=EDGE_CURVE ( 'NONE', #4062, #9157, #11237, .T. ) ;
#14469=( GEOMETRIC_REPRESENTATION_CONTEXT ( 3 ) GLOBAL_UNCERTAINTY_ASSIGNED_CONTEXT ( ( #100 ) ) GLOBAL_UNIT_ASSIGNED_CONTEXT ( ( #13795, #7486, #6245 ) ) REPRESENTATION_CONTEXT ( 'NONE', 'WORKASPACE' ) );
#14476=CARTESIAN_POINT ( 'NONE',  ( 40.34137639590981195, 35.12187500034139731, -29.30972558990011834 ) ) ;
#14477=CARTESIAN_POINT ( 'NONE',  ( -49.86468353124999453, 35.75937500034139305, -16.20201782572375393 ) ) ;
#14480=CARTESIAN_POINT ( 'NONE',  ( -15.45084971874737256, 43.60000000000000142, -47.55282581475767500 ) ) ;
#14484=CARTESIAN_POINT ( 'NONE',  ( 15.45084971874736723, 21.18125000068279817, -47.55282581475768211 ) ) ;
#14487=CARTESIAN_POINT ( 'NONE',  ( 30.90169943749474157, 49.29999999999999716, -42.53254041760200721 ) ) ;
#14496=ORIENTED_EDGE ( 'NONE', *, *, #14044, .T. ) ;
#14498=CARTESIAN_POINT ( 'NONE',  ( 7.919222016226940219, 31.22999571913595673, -49.99999999999996447 ) ) ;
#14500=CARTESIAN_POINT ( 'NONE',  ( -3.210462471511496205E-15, 23.35937500034139802, -52.43083105670540789 ) ) ;
#14502=VECTOR ( 'NONE', #158, 1000.000000000000000 ) ;
#14504=CARTESIAN_POINT ( 'NONE',  ( 15.45084971874736723, 35.39999999999999858, -47.55282581475768211 ) ) ;
#14507=( BOUNDED_CURVE ( )  B_SPLINE_CURVE ( 2, ( #1817, #6910, #11964, #10884, #8542, #16121, #4569, #9632, #10963, #7227, #12287, #11142, #3566 ),
 .UNSPECIFIED., .F., .F. ) 
 B_SPLINE_CURVE_WITH_KNOTS ( ( 3, 2, 2, 2, 2, 2, 3 ),
 ( 0.4166666666666666852, 0.4199999999999999845, 0.4266666666666666941, 0.4333333333333333481, 0.4400000000000000022, 0.4466666666666666563, 0.4500000000000000111 ),
 .UNSPECIFIED. ) 
 CURVE ( )  GEOMETRIC_REPRESENTATION_ITEM ( )  RATIONAL_B_SPLINE_CURVE ( ( 0.9755282581475768211, 0.9755282581475770431, 1.000000000000000000, 0.9510565162951535312, 1.000000000000000000, 0.9510565162951535312, 1.000000000000000000, 0.9510565162951535312, 1.000000000000000000, 0.9510565162951535312, 1.000000000000000000, 0.9755282581475765991, 0.9755282581475768211 ) ) 
 REPRESENTATION_ITEM ( '' )  );
#14508=CARTESIAN_POINT ( 'NONE',  ( -49.86468353124999453, 45.82187500034140015, -16.20201782572375393 ) ) ;
#14517=DIRECTION ( 'NONE',  ( 0.000000000000000000, 0.000000000000000000, 1.000000000000000000 ) ) ;
#14518=CARTESIAN_POINT ( 'NONE',  ( 0.000000000000000000, 50.00000000000000000, 0.000000000000000000 ) ) ;
#14520=CARTESIAN_POINT ( 'NONE',  ( 49.86468353125001585, 46.75937500034140015, 16.20201782572375038 ) ) ;
#14521=CARTESIAN_POINT ( 'NONE',  ( 15.40903463028481113, 47.25937500034140015, -47.42413220539094709 ) ) ;
#14528=CARTESIAN_POINT ( 'NONE',  ( -2.547328955960238000E-13, 20.28125000068279959, 49.99999999999999289 ) ) ;
#14546=CARTESIAN_POINT ( 'NONE',  ( 1.157856716130699404, 5.028685516365632324, 99.10823101669018342 ) ) ;
#14547=CARTESIAN_POINT ( 'NONE',  ( -47.74744883082067304, 20.00000000000000355, 14.37691108325808109 ) ) ;
#14548=CARTESIAN_POINT ( 'NONE',  ( 40.34137639590981905, 22.72187500034139518, 29.30972558990010768 ) ) ;
#14551=CARTESIAN_POINT ( 'NONE',  ( -49.86468353124999453, 23.95937500034138878, 16.20201782572377525 ) ) ;
#14552=EDGE_CURVE ( 'NONE', #11668, #842, #14555, .T. ) ;
#14553=CARTESIAN_POINT ( 'NONE',  ( -7.919222016226816763, 29.55125428154684286, -49.99999999999999289 ) ) ;
#14555=( BOUNDED_CURVE ( )  B_SPLINE_CURVE ( 2, ( #9886, #8878, #10132, #13612, #5984, #16447, #2311, #8543, #16358, #4998, #15182, #7550, #7396 ),
 .UNSPECIFIED., .F., .F. ) 
 B_SPLINE_CURVE_WITH_KNOTS ( ( 3, 2, 2, 2, 2, 2, 3 ),
 ( 0.2500000000000000000, 0.2533333333333333548, 0.2600000000000000089, 0.2666666666666666630, 0.2733333333333333171, 0.2800000000000000266, 0.2833333333333333814 ),
 .UNSPECIFIED. ) 
 CURVE ( )  GEOMETRIC_REPRESENTATION_ITEM ( )  RATIONAL_B_SPLINE_CURVE ( ( 0.9755282581475765991, 0.9755282581475765991, 1.000000000000000000, 0.9510565162951535312, 1.000000000000000000, 0.9510565162951535312, 1.000000000000000000, 0.9510565162951535312, 1.000000000000000000, 0.9510565162951535312, 1.000000000000000000, 0.9755282581475765991, 0.9755282581475768211 ) ) 
 REPRESENTATION_ITEM ( '' )  );
#14564=CARTESIAN_POINT ( 'NONE',  ( 30.81806926056962936, 31.22187500034139873, -42.41743335407647209 ) ) ;
#14565=CARTESIAN_POINT ( 'NONE',  ( 49.86468353124999453, 38.95937500034139589, -16.20201782572376104 ) ) ;
#14566=CARTESIAN_POINT ( 'NONE',  ( -40.45084971874737789, 43.80000000000000426, -29.38926261462365730 ) ) ;
#14569=CARTESIAN_POINT ( 'NONE',  ( -40.34137639590981905, 43.65937500034139163, -29.30972558990011478 ) ) ;
#14571=CARTESIAN_POINT ( 'NONE',  ( 49.86468353124999453, 21.02187500034139589, -16.20201782572376459 ) ) ;
#14580=CARTESIAN_POINT ( 'NONE',  ( -30.81806926056963292, 47.62187500034139731, -42.41743335407647209 ) ) ;
#14584=CARTESIAN_POINT ( 'NONE',  ( -40.45084971874737079, 36.20000000000000284, 29.38926261462367151 ) ) ;
#14585=CARTESIAN_POINT ( 'NONE',  ( 49.86468353125000164, 38.92187500034139447, -6.106662507704105588E-15 ) ) ;
#14594=DIRECTION ( 'NONE',  ( -0.000000000000000000, 1.000000000000000000, -0.000000000000000000 ) ) ;
#14596=LINE ( 'NONE', #5645, #4255 ) ;
#14599=CARTESIAN_POINT ( 'NONE',  ( 30.81806926056962936, 35.15937500034139873, -42.41743335407647209 ) ) ;
#14600=CARTESIAN_POINT ( 'NONE',  ( -30.81806926056962226, 46.15937500034139873, 42.41743335407647209 ) ) ;
#14603=DIRECTION ( 'NONE',  ( -0.000000000000000000, 1.000000000000000000, -0.000000000000000000 ) ) ;
#14608=ORIENTED_EDGE ( 'NONE', *, *, #73, .F. ) ;
#14618=CYLINDRICAL_SURFACE ( 'NONE', #942, 50.00000000000000000 ) ;
#14620=DIRECTION ( 'NONE',  ( -0.000000000000000000, -1.000000000000000000, -0.000000000000000000 ) ) ;
#14623=CARTESIAN_POINT ( 'NONE',  ( -15.45084971874737256, 47.60000000000000142, -47.55282581475767500 ) ) ;
#14624=CARTESIAN_POINT ( 'NONE',  ( 6.123233995736766085E-15, 20.00000000000000355, -50.00000000000000000 ) ) ;
#14626=CARTESIAN_POINT ( 'NONE',  ( 15.40903463028482356, 20.52187500034139589, 47.42413220539093999 ) ) ;
#14630=CARTESIAN_POINT ( 'NONE',  ( 49.86468353125000164, 28.85937500034139802, -6.106662507704105588E-15 ) ) ;
#14634=EDGE_CURVE ( 'NONE', #14047, #16188, #16263, .T. ) ;
#14637=CYLINDRICAL_SURFACE ( 'NONE', #8141, 50.00000000000000000 ) ;
#14641=CARTESIAN_POINT ( 'NONE',  ( 49.86468353125001585, 30.82187500034139660, 16.20201782572375038 ) ) ;
#14642=CARTESIAN_POINT ( 'NONE',  ( 49.86468353125000164, 28.85937500034139802, -6.106662507704105588E-15 ) ) ;
#14643=CARTESIAN_POINT ( 'NONE',  ( 30.90169943749473802, 27.08125000068280031, -42.53254041760200721 ) ) ;
#14646=CARTESIAN_POINT ( 'NONE',  ( -40.34137639590981195, 42.05937500034139731, 29.30972558990012189 ) ) ;
#14648=CARTESIAN_POINT ( 'NONE',  ( 40.34137639590981905, 20.72187500034139873, 29.30972558990010768 ) ) ;
#14657=CARTESIAN_POINT ( 'NONE',  ( -30.90169943749474513, 33.48125000068279888, -42.53254041760200721 ) ) ;
#14659=CARTESIAN_POINT ( 'NONE',  ( -15.40903463028481646, 47.52187500034139589, -47.42413220539093999 ) ) ;
#14662=CARTESIAN_POINT ( 'NONE',  ( -40.45084971874737079, 38.20000000000000284, 29.38926261462367151 ) ) ;
#14663=CARTESIAN_POINT ( 'NONE',  ( 30.81806926056962936, 41.22187500034139873, -42.41743335407647209 ) ) ;
#14669=VERTEX_POINT ( 'NONE', #1471 ) ;
#14673=CARTESIAN_POINT ( 'NONE',  ( -50.00000000000000000, 39.78125000068279604, 0.000000000000000000 ) ) ;
#14678=CARTESIAN_POINT ( 'NONE',  ( -3.210462471511496205E-15, 35.35937500034140157, -52.43083105670540789 ) ) ;
#14679=CARTESIAN_POINT ( 'NONE',  ( 9.631387414534489405E-15, 48.35937500034139447, 52.43083105670540789 ) ) ;
#14684=CARTESIAN_POINT ( 'NONE',  ( 6.123233995736766085E-15, 20.00000000000000355, -50.00000000000000000 ) ) ;
#14685=CARTESIAN_POINT ( 'NONE',  ( 15.45084971874737789, 40.60000000000000142, 47.55282581475767500 ) ) ;
#14692=ORIENTED_EDGE ( 'NONE', *, *, #9148, .F. ) ;
#14698=FACE_OUTER_BOUND ( 'NONE', #5487, .T. ) ;
#14701=LINE ( 'NONE', #6999, #6761 ) ;
#14704=CARTESIAN_POINT ( 'NONE',  ( -45.87472660798568569, 20.00000000000000355, 19.54543171153602188 ) ) ;
#14708=CARTESIAN_POINT ( 'NONE',  ( 15.40903463028481113, 25.25937500034139660, -47.42413220539094709 ) ) ;
#14710=ORIENTED_EDGE ( 'NONE', *, *, #3090, .T. ) ;
#14713=CARTESIAN_POINT ( 'NONE',  ( -3.111920190527341144E-15, 45.50000000000000000, -50.00000000000000000 ) ) ;
#14719=CARTESIAN_POINT ( 'NONE',  ( 8.446640517145639571E-15, 28.28125000068279959, 50.00000000000000000 ) ) ;
#14722=CARTESIAN_POINT ( 'NONE',  ( 40.34137639590981195, 31.12187500034139731, -29.30972558990011834 ) ) ;
#14723=CARTESIAN_POINT ( 'NONE',  ( 30.81806926056964002, 26.55937500034139376, 42.41743335407646498 ) ) ;
#14728=CARTESIAN_POINT ( 'NONE',  ( -40.34137639590981195, 44.05937500034139731, 29.30972558990012189 ) ) ;
#14731=CARTESIAN_POINT ( 'NONE',  ( -49.99999999999999289, 49.89999999999999147, -16.24598481164531449 ) ) ;
#14732=ORIENTED_EDGE ( 'NONE', *, *, #1637, .T. ) ;
#14740=CARTESIAN_POINT ( 'NONE',  ( -2.547328955960238000E-13, 34.50000000000000000, 49.99999999999999289 ) ) ;
#14742=CARTESIAN_POINT ( 'NONE',  ( 40.34137639590981195, 21.05937500034139376, -29.30972558990011834 ) ) ;
#14745=( BOUNDED_CURVE ( )  B_SPLINE_CURVE ( 2, ( #14713, #9837, #2003, #13560, #16150, #13640, #9757, #6102, #8496, #841, #9917, #3516, #12491 ),
 .UNSPECIFIED., .F., .F. ) 
 B_SPLINE_CURVE_WITH_KNOTS ( ( 3, 2, 2, 2, 2, 2, 3 ),
 ( 0.1499999999999999944, 0.1533333333333333215, 0.1600000000000000033, 0.1666666666666666574, 0.1733333333333333393, 0.1799999999999999933, 0.1833333333333333481 ),
 .UNSPECIFIED. ) 
 CURVE ( )  GEOMETRIC_REPRESENTATION_ITEM ( )  RATIONAL_B_SPLINE_CURVE ( ( 0.9755282581475768211, 0.9755282581475768211, 1.000000000000000000, 0.9510565162951535312, 1.000000000000000000, 0.9510565162951535312, 1.000000000000000000, 0.9510565162951535312, 1.000000000000000000, 0.9510565162951535312, 1.000000000000000000, 0.9755282581475765991, 0.9755282581475767101 ) ) 
 REPRESENTATION_ITEM ( '' )  );
#14747=CARTESIAN_POINT ( 'NONE',  ( 40.45084971874737079, 34.98125000068279888, -29.38926261462366440 ) ) ;
#14748=CARTESIAN_POINT ( 'NONE',  ( -49.99999999999999289, 38.10000000000000142, 16.24598481164533226 ) ) ;
#14749=CARTESIAN_POINT ( 'NONE',  ( -49.86468353124999453, 37.82187500034139305, -16.20201782572375393 ) ) ;
#14754=EDGE_LOOP ( 'NONE', ( #8194, #2376, #5742 ) ) ;
#14758=ORIENTED_EDGE ( 'NONE', *, *, #5123, .F. ) ;
#14763=CARTESIAN_POINT ( 'NONE',  ( -7.919222016226688865, 21.33250428222963890, -50.00000000000003553 ) ) ;
#14764=FACE_OUTER_BOUND ( 'NONE', #8989, .T. ) ;
#14766=CARTESIAN_POINT ( 'NONE',  ( -30.81806926056963292, 35.55937500034139020, -42.41743335407647209 ) ) ;
#14767=CARTESIAN_POINT ( 'NONE',  ( 1.084250397222511456E-14, 50.00000000000000000, 85.01963570546854498 ) ) ;
#14769=AXIS2_PLACEMENT_3D ( 'NONE', #7180, #5935, #10999 ) ;
#14788=DIRECTION ( 'NONE',  ( -0.000000000000000000, 1.000000000000000000, -0.000000000000000000 ) ) ;
#14790=PLANE ( 'NONE',  #14951 ) ;
#14794=CARTESIAN_POINT ( 'NONE',  ( 15.40903463028482356, 22.52187500034139589, 47.42413220539093999 ) ) ;
#14797=CARTESIAN_POINT ( 'NONE',  ( -30.81806926056962226, 26.15937500034139163, 42.41743335407647919 ) ) ;
#14799=CARTESIAN_POINT ( 'NONE',  ( -7.919222016226934890, 30.44874571845316069, 49.99999999999996447 ) ) ;
#14812=CARTESIAN_POINT ( 'NONE',  ( -49.86468353124999453, 32.02187500034139589, 16.20201782572377525 ) ) ;
#14813=CARTESIAN_POINT ( 'NONE',  ( 15.40903463028481113, 31.25937500034140015, -47.42413220539094709 ) ) ;
#14814=CARTESIAN_POINT ( 'NONE',  ( -30.90169943749473447, 36.29999999999999716, 42.53254041760200721 ) ) ;
#14817=CARTESIAN_POINT ( 'NONE',  ( -49.86468353124999453, 45.95937500034138878, 16.20201782572377525 ) ) ;
#14819=CARTESIAN_POINT ( 'NONE',  ( -49.86468353125000164, 19.92187500034139447, 0.000000000000000000 ) ) ;
#14830=CARTESIAN_POINT ( 'NONE',  ( 9.631387414534489405E-15, 48.42187500034140157, 52.43083105670540789 ) ) ;
#14834=CARTESIAN_POINT ( 'NONE',  ( -49.99999999999999289, 31.68125000068279462, -16.24598481164531449 ) ) ;
#14836=CARTESIAN_POINT ( 'NONE',  ( -3.210462471511496205E-15, 43.42187500034140157, -52.43083105670540789 ) ) ;
#14845=ORIENTED_EDGE ( 'NONE', *, *, #1295, .F. ) ;
#14846=CARTESIAN_POINT ( 'NONE',  ( -15.45084971874736368, 40.18125000068280173, 47.55282581475768211 ) ) ;
#14852=CARTESIAN_POINT ( 'NONE',  ( -15.40903463028480580, 38.25937500034140015, 47.42413220539094709 ) ) ;
#14853=CARTESIAN_POINT ( 'NONE',  ( 49.86468353125001585, 48.75937500034140015, 16.20201782572375038 ) ) ;
#14858=DIRECTION ( 'NONE',  ( 0.000000000000000000, 0.000000000000000000, 1.000000000000000000 ) ) ;
#14864=EDGE_CURVE ( 'NONE', #13242, #13843, #14026, .T. ) ;
#14867=DIRECTION ( 'NONE',  ( 0.000000000000000000, 0.000000000000000000, 1.000000000000000000 ) ) ;
#14868=SURFACE_STYLE_USAGE ( .BOTH. , #6084 ) ;
#14870=CARTESIAN_POINT ( 'NONE',  ( -40.45084971874737079, 47.98125000068279888, 29.38926261462367151 ) ) ;
#14872=CARTESIAN_POINT ( 'NONE',  ( -17.47218334215669344, 21.35978834315422503, 94.63430745020650647 ) ) ;
#14876=CARTESIAN_POINT ( 'NONE',  ( -40.45084971874737789, 47.80000000000000426, -29.38926261462365730 ) ) ;
#14878=CARTESIAN_POINT ( 'NONE',  ( -46.00435827497687313, 20.00000000000000355, 19.23833313609354434 ) ) ;
#14879=CARTESIAN_POINT ( 'NONE',  ( -15.45084971874736368, 44.18125000068280173, 47.55282581475768211 ) ) ;
#14882=CARTESIAN_POINT ( 'NONE',  ( -40.34137639590981905, 21.65937500034139518, -29.30972558990011478 ) ) ;
#14883=CARTESIAN_POINT ( 'NONE',  ( -40.45084971874737789, 41.58125000068280031, -29.38926261462365730 ) ) ;
#14886=EDGE_CURVE ( 'NONE', #12470, #8883, #2043, .T. ) ;
#14887=ORIENTED_EDGE ( 'NONE', *, *, #564, .F. ) ;
#14890=CARTESIAN_POINT ( 'NONE',  ( 1.022488062601840571E-14, 49.50000000000000711, -50.00000000000000000 ) ) ;
#14895=CARTESIAN_POINT ( 'NONE',  ( 50.00000000000000000, 28.78125000068279959, -6.123233995736766085E-15 ) ) ;
#14897=CARTESIAN_POINT ( 'NONE',  ( 9.631387414534489405E-15, 24.42187500034139447, 52.43083105670540789 ) ) ;
#14898=CARTESIAN_POINT ( 'NONE',  ( 9.631387414534489405E-15, 30.35937500034139092, 52.43083105670540789 ) ) ;
#14899=CARTESIAN_POINT ( 'NONE',  ( -30.90169943749474513, 35.69999999999999574, -42.53254041760200721 ) ) ;
#14900=CARTESIAN_POINT ( 'NONE',  ( -30.81806926056962226, 34.22187500034139163, 42.41743335407647209 ) ) ;
#14902=CARTESIAN_POINT ( 'NONE',  ( 49.86468353125000164, 46.85937500034139447, -6.106662507704105588E-15 ) ) ;
#14904=CARTESIAN_POINT ( 'NONE',  ( 9.657523855033129090E-15, 44.50000000000000711, 52.57311121191334990 ) ) ;
#14909=VERTEX_POINT ( 'NONE', #13675 ) ;
#14911=CARTESIAN_POINT ( 'NONE',  ( -49.86468353124999453, 47.82187500034140015, -16.20201782572375393 ) ) ;
#14913=CYLINDRICAL_SURFACE ( 'NONE', #6258, 50.00000000000000000 ) ;
#14915=CARTESIAN_POINT ( 'NONE',  ( -50.00000000000000000, 35.78125000068280315, 0.000000000000000000 ) ) ;
#14916=CARTESIAN_POINT ( 'NONE',  ( 30.81806926056964002, 38.62187500034139731, 42.41743335407647209 ) ) ;
#14928=CARTESIAN_POINT ( 'NONE',  ( -49.99999999999999289, 49.68125000068279462, -16.24598481164531449 ) ) ;
#14930=CARTESIAN_POINT ( 'NONE',  ( -49.86468353125000164, 39.85937500034139447, 0.000000000000000000 ) ) ;
#14931=CARTESIAN_POINT ( 'NONE',  ( -30.81806926056962226, 42.15937500034139163, 42.41743335407647209 ) ) ;
#14932=CARTESIAN_POINT ( 'NONE',  ( 40.45084971874737079, 25.19999999999999929, -29.38926261462366440 ) ) ;
#14937=CARTESIAN_POINT ( 'NONE',  ( -48.35726954556750457, 20.00000000000000355, 12.16803787670978387 ) ) ;
#14939=CARTESIAN_POINT ( 'NONE',  ( -1.240322475938754499E-13, 40.50000000000000000, 50.00000000000000000 ) ) ;
#14946=ORIENTED_EDGE ( 'NONE', *, *, #15358, .T. ) ;
#14947=( BOUNDED_CURVE ( )  B_SPLINE_CURVE ( 2, ( #425, #3092, #9168, #8170, #4193, #7835, #8078, #1597, #10744, #5530, #10591, #4271, #13238 ),
 .UNSPECIFIED., .F., .T. ) 
 B_SPLINE_CURVE_WITH_KNOTS ( ( 3, 2, 2, 2, 2, 2, 3 ),
 ( 0.9166666666666667407, 0.9200000000000000400, 0.9266666666666666385, 0.9333333333333333481, 0.9399999999999999467, 0.9466666666666666563, 0.9500000000000000666 ),
 .UNSPECIFIED. ) 
 CURVE ( )  GEOMETRIC_REPRESENTATION_ITEM ( )  RATIONAL_B_SPLINE_CURVE ( ( 0.9755282581475768211, 0.9755282581475771542, 1.000000000000000000, 0.9510565162951535312, 1.000000000000000000, 0.9510565162951535312, 1.000000000000000000, 0.9510565162951535312, 1.000000000000000000, 0.9510565162951535312, 1.000000000000000000, 0.9755282581475763770, 0.9755282581475768211 ) ) 
 REPRESENTATION_ITEM ( '' )  );
#14949=CARTESIAN_POINT ( 'NONE',  ( -15.45084971874736368, 40.40000000000000568, 47.55282581475768211 ) ) ;
#14951=AXIS2_PLACEMENT_3D ( 'NONE', #829, #749, #16138 ) ;
#14958=DIRECTION ( 'NONE',  ( -0.000000000000000000, 1.000000000000000000, -0.000000000000000000 ) ) ;
#14961=CARTESIAN_POINT ( 'NONE',  ( -45.67643563157982101, 19.99999999999998934, 20.00444126042745197 ) ) ;
#14962=CARTESIAN_POINT ( 'NONE',  ( 49.99999999999999289, 46.88125000068279036, -16.24598481164532160 ) ) ;
#14977=AXIS2_PLACEMENT_3D ( 'NONE', #1984, #11593, #15411 ) ;
#14979=CARTESIAN_POINT ( 'NONE',  ( 9.631387414534489405E-15, 20.42187500034139802, 52.43083105670540789 ) ) ;
#14980=CARTESIAN_POINT ( 'NONE',  ( -15.40903463028480580, 28.25937500034139660, 47.42413220539094709 ) ) ;
#14982=CARTESIAN_POINT ( 'NONE',  ( 40.34137639590981905, 32.72187500034139873, 29.30972558990010768 ) ) ;
#14984=CARTESIAN_POINT ( 'NONE',  ( 15.40903463028482356, 36.45937500034139589, 47.42413220539093999 ) ) ;
#14986=CARTESIAN_POINT ( 'NONE',  ( -3.219174618344376363E-15, 47.49999999999999289, -52.57311121191334990 ) ) ;
#14987=EDGE_CURVE ( 'NONE', #4733, #15952, #2032, .T. ) ;
#14988=EDGE_LOOP ( 'NONE', ( #2342, #5639, #5680, #1821, #250, #3198 ) ) ;
#14994=CARTESIAN_POINT ( 'NONE',  ( 15.45084971874737789, 40.38125000068280457, 47.55282581475767500 ) ) ;
#14995=CARTESIAN_POINT ( 'NONE',  ( 49.86468353124999453, 41.02187500034139589, -16.20201782572376459 ) ) ;
#14999=CARTESIAN_POINT ( 'NONE',  ( 40.45084971874737079, 28.98125000068279888, -29.38926261462366440 ) ) ;
#15001=CARTESIAN_POINT ( 'NONE',  ( 30.81806926056964002, 32.62187500034140442, 42.41743335407647209 ) ) ;
#15006=AXIS2_PLACEMENT_3D ( 'NONE', #3285, #16175, #4805 ) ;
#15007=VERTEX_POINT ( 'NONE', #6382 ) ;
#15015=CARTESIAN_POINT ( 'NONE',  ( -49.86468353125000164, 29.85937500034139802, 0.000000000000000000 ) ) ;
#15016=CARTESIAN_POINT ( 'NONE',  ( 15.40903463028482356, 40.45937500034139589, 47.42413220539093999 ) ) ;
#15021=AXIS2_PLACEMENT_3D ( 'NONE', #11067, #14788, #9981 ) ;
#15045=FACE_OUTER_BOUND ( 'NONE', #13763, .T. ) ;
#15046=CARTESIAN_POINT ( 'NONE',  ( -50.00000000000000000, 49.78125000068280315, 0.000000000000000000 ) ) ;
#15047=CARTESIAN_POINT ( 'NONE',  ( 15.45084971874736723, 21.40000000000000213, -47.55282581475768211 ) ) ;
#15050=CARTESIAN_POINT ( 'NONE',  ( -49.86468353125000164, 21.85937500034139802, 0.000000000000000000 ) ) ;
#15053=VECTOR ( 'NONE', #15688, 1000.000000000000000 ) ;
#15066=CARTESIAN_POINT ( 'NONE',  ( -15.40903463028481646, 23.52187500034139944, -47.42413220539093999 ) ) ;
#15067=CARTESIAN_POINT ( 'NONE',  ( 30.81806926056964002, 20.55937500034139376, 42.41743335407646498 ) ) ;
#15069=CARTESIAN_POINT ( 'NONE',  ( -3.210462471511496205E-15, 33.42187500034139447, -52.43083105670540789 ) ) ;
#15071=CARTESIAN_POINT ( 'NONE',  ( -30.90169943749473802, 40.30000000000000426, 42.53254041760200721 ) ) ;
#15072=CARTESIAN_POINT ( 'NONE',  ( -49.86468353124999453, 39.75937500034139305, -16.20201782572375393 ) ) ;
#15074=CARTESIAN_POINT ( 'NONE',  ( 30.90169943749475578, 46.69999999999999574, 42.53254041760200010 ) ) ;
#15078=EDGE_LOOP ( 'NONE', ( #1920, #11723, #12385, #8021 ) ) ;
#15085=CARTESIAN_POINT ( 'NONE',  ( 49.86468353125000164, 42.92187500034140157, -6.106662507704105588E-15 ) ) ;
#15088=CARTESIAN_POINT ( 'NONE',  ( -40.45084971874737789, 29.58125000068279675, -29.38926261462365730 ) ) ;
#15089=CARTESIAN_POINT ( 'NONE',  ( 30.81806926056964002, 36.62187500034139731, 42.41743335407647209 ) ) ;
#15101=CARTESIAN_POINT ( 'NONE',  ( 15.40903463028481113, 29.25937500034139660, -47.42413220539094709 ) ) ;
#15103=CARTESIAN_POINT ( 'NONE',  ( 30.81806926056964002, 44.62187500034139731, 42.41743335407646498 ) ) ;
#15110=ORIENTED_EDGE ( 'NONE', *, *, #5307, .F. ) ;
#15116=VERTEX_POINT ( 'NONE', #2538 ) ;
#15125=CARTESIAN_POINT ( 'NONE',  ( -30.90169943749474868, 49.48125000068279178, -42.53254041760200721 ) ) ;
#15128=CARTESIAN_POINT ( 'NONE',  ( 0.000000000000000000, 50.00000000000000000, -85.01963570546854498 ) ) ;
#15129=CARTESIAN_POINT ( 'NONE',  ( -2.317185599438165467E-15, 40.00000000000004974, 92.94692077166139654 ) ) ;
#15137=CARTESIAN_POINT ( 'NONE',  ( -4.545615046168190787, 39.40905366563087853, 92.94163982466287166 ) ) ;
#15141=CARTESIAN_POINT ( 'NONE',  ( 30.81806926056962936, 25.22187500034139873, -42.41743335407647209 ) ) ;
#15142=CARTESIAN_POINT ( 'NONE',  ( 15.40903463028481113, 21.25937500034139660, -47.42413220539094709 ) ) ;
#15144=CARTESIAN_POINT ( 'NONE',  ( 9.631387414534489405E-15, 32.42187500034139447, 52.43083105670540789 ) ) ;
#15148=CARTESIAN_POINT ( 'NONE',  ( -40.45084971874737079, 34.20000000000000284, 29.38926261462367151 ) ) ;
#15149=CARTESIAN_POINT ( 'NONE',  ( 15.40903463028482356, 38.45937500034139589, 47.42413220539093999 ) ) ;
#15152=CARTESIAN_POINT ( 'NONE',  ( 49.99999999999999289, 45.10000000000000853, -16.24598481164532160 ) ) ;
#15159=CARTESIAN_POINT ( 'NONE',  ( 2.600676159226420495E-13, 33.49999999999999289, -49.99999999999999289 ) ) ;
#15162=CARTESIAN_POINT ( 'NONE',  ( 15.40903463028482356, 40.52187500034139589, 47.42413220539093999 ) ) ;
#15165=CARTESIAN_POINT ( 'NONE',  ( -3.219174618344376363E-15, 29.28125000068279604, -52.57311121191334990 ) ) ;
#15168=CARTESIAN_POINT ( 'NONE',  ( -30.81806926056963292, 31.62187500034139731, -42.41743335407647209 ) ) ;
#15169=CARTESIAN_POINT ( 'NONE',  ( 40.45084971874737079, 39.19999999999999574, -29.38926261462366440 ) ) ;
#15176=CARTESIAN_POINT ( 'NONE',  ( 0.000000000000000000, 28.00000000000000355, -10.00000000000000000 ) ) ;
#15177=CARTESIAN_POINT ( 'NONE',  ( -49.86468353124999453, 29.95937500034139944, 16.20201782572377525 ) ) ;
#15179=CARTESIAN_POINT ( 'NONE',  ( 15.40903463028481113, 47.32187500034140015, -47.42413220539094709 ) ) ;
#15180=DIRECTION ( 'NONE',  ( 0.000000000000000000, 0.000000000000000000, -1.000000000000000000 ) ) ;
#15182=CARTESIAN_POINT ( 'NONE',  ( -15.45084971874737256, 41.60000000000000142, -47.55282581475767500 ) ) ;
#15191=VERTEX_POINT ( 'NONE', #10833 ) ;
#15192=CARTESIAN_POINT ( 'NONE',  ( -1.240322475938754499E-13, 40.28125000068280315, 50.00000000000000000 ) ) ;
#15201=CARTESIAN_POINT ( 'NONE',  ( 30.90169943749475578, 44.48125000068279888, 42.53254041760200010 ) ) ;
#15202=CARTESIAN_POINT ( 'NONE',  ( 15.45084971874737789, 44.38125000068279746, 47.55282581475767500 ) ) ;
#15210=ORIENTED_EDGE ( 'NONE', *, *, #11870, .F. ) ;
#15219=CARTESIAN_POINT ( 'NONE',  ( 49.86468353124999453, 24.95937500034139234, -16.20201782572376104 ) ) ;
#15221=CARTESIAN_POINT ( 'NONE',  ( 15.40903463028481113, 37.32187500034140015, -47.42413220539094709 ) ) ;
#15223=CARTESIAN_POINT ( 'NONE',  ( 15.45084971874736723, 33.39999999999999858, -47.55282581475768211 ) ) ;
#15224=CARTESIAN_POINT ( 'NONE',  ( -49.86468353125000164, 35.85937500034140157, 0.000000000000000000 ) ) ;
#15227=CARTESIAN_POINT ( 'NONE',  ( -50.00000000000000000, 44.00000000000000711, 0.000000000000000000 ) ) ;
#15235=EDGE_CURVE ( 'NONE', #13843, #384, #15724, .T. ) ;
#15244=CARTESIAN_POINT ( 'NONE',  ( -49.86468353124999453, 41.82187500034140015, -16.20201782572375393 ) ) ;
#15247=CARTESIAN_POINT ( 'NONE',  ( 15.45084971874737789, 30.38125000068280102, 47.55282581475767500 ) ) ;
#15248=CARTESIAN_POINT ( 'NONE',  ( -30.90169943749474513, 35.48125000068279888, -42.53254041760200721 ) ) ;
#15250=CARTESIAN_POINT ( 'NONE',  ( 30.81806926056962936, 33.22187500034139163, -42.41743335407647209 ) ) ;
#15252=EDGE_LOOP ( 'NONE', ( #13352, #15441, #1273, #5784, #8331, #1185, #8931 ) ) ;
#15258=CARTESIAN_POINT ( 'NONE',  ( 0.000000000000000000, 20.00000000000000355, 0.000000000000000000 ) ) ;
#15259=CARTESIAN_POINT ( 'NONE',  ( -49.86468353124999453, 29.75937500034139305, -16.20201782572375393 ) ) ;
#15261=CARTESIAN_POINT ( 'NONE',  ( 40.34137639590981905, 48.72187500034139873, 29.30972558990010768 ) ) ;
#15270=CARTESIAN_POINT ( 'NONE',  ( -40.45084971874737789, 45.58125000068280031, -29.38926261462365730 ) ) ;
#15277=DIRECTION ( 'NONE',  ( -0.000000000000000000, 1.000000000000000000, -0.000000000000000000 ) ) ;
#15284=CARTESIAN_POINT ( 'NONE',  ( 50.00000000000000000, 24.78125000068279959, -6.123233995736766085E-15 ) ) ;
#15289=CARTESIAN_POINT ( 'NONE',  ( -40.45084971874737789, 41.58125000068280031, -29.38926261462365730 ) ) ;
#15290=( BOUNDED_CURVE ( )  B_SPLINE_CURVE ( 2, ( #12424, #9767, #7272, #14643, #12328, #8578, #6112, #3526, #11100, #9847, #7434, #5779, #3271 ),
 .UNSPECIFIED., .F., .T. ) 
 B_SPLINE_CURVE_WITH_KNOTS ( ( 3, 2, 2, 2, 2, 2, 3 ),
 ( 0.7500000000000000000, 0.7533333333333332993, 0.7600000000000000089, 0.7666666666666667185, 0.7733333333333333171, 0.7800000000000000266, 0.7833333333333333259 ),
 .UNSPECIFIED. ) 
 CURVE ( )  GEOMETRIC_REPRESENTATION_ITEM ( )  RATIONAL_B_SPLINE_CURVE ( ( 0.9755282581475768211, 0.9755282581475768211, 1.000000000000000000, 0.9510565162951535312, 1.000000000000000000, 0.9510565162951535312, 1.000000000000000000, 0.9510565162951535312, 1.000000000000000000, 0.9510565162951535312, 1.000000000000000000, 0.9755282581475768211, 0.9755282581475768211 ) ) 
 REPRESENTATION_ITEM ( '' )  );
#15291=CARTESIAN_POINT ( 'NONE',  ( 30.90169943749475223, 20.69999999999999574, 42.53254041760199300 ) ) ;
#15292=CARTESIAN_POINT ( 'NONE',  ( 50.00000000000000000, 46.78125000068279604, -6.123233995736766085E-15 ) ) ;
#15294=ORIENTED_EDGE ( 'NONE', *, *, #4180, .T. ) ;
#15300=CYLINDRICAL_SURFACE ( 'NONE', #11288, 17.50000000000000000 ) ;
#15310=CARTESIAN_POINT ( 'NONE',  ( -30.81806926056962226, 26.15937500034139163, 42.41743335407647209 ) ) ;
#15311=VECTOR ( 'NONE', #198, 1000.000000000000114 ) ;
#15313=CARTESIAN_POINT ( 'NONE',  ( 15.40903463028481113, 31.32187500034139305, -47.42413220539094709 ) ) ;
#15316=CARTESIAN_POINT ( 'NONE',  ( -30.90169943749473802, 32.30000000000000426, 42.53254041760200721 ) ) ;
#15317=CARTESIAN_POINT ( 'NONE',  ( -49.86468353124999453, 37.95937500034140299, 16.20201782572377525 ) ) ;
#15319=CARTESIAN_POINT ( 'NONE',  ( -49.99999999999999289, 41.90000000000001279, -16.24598481164531449 ) ) ;
#15320=VERTEX_POINT ( 'NONE', #4607 ) ;
#15331=CARTESIAN_POINT ( 'NONE',  ( -15.40903463028481646, 41.52187500034139589, -47.42413220539093999 ) ) ;
#15332=CARTESIAN_POINT ( 'NONE',  ( 30.81806926056964002, 42.55937500034139020, 42.41743335407646498 ) ) ;
#15335=CARTESIAN_POINT ( 'NONE',  ( 15.45084971874737789, 28.38125000068279746, 47.55282581475767500 ) ) ;
#15336=EDGE_CURVE ( 'NONE', #4175, #13132, #12867, .T. ) ;
#15338=CARTESIAN_POINT ( 'NONE',  ( -3.111920190527341144E-15, 35.28125000068280315, -50.00000000000000000 ) ) ;
#15339=CARTESIAN_POINT ( 'NONE',  ( 40.34137639590981905, 36.72187500034139163, 29.30972558990010768 ) ) ;
#15349=CARTESIAN_POINT ( 'NONE',  ( -40.34137639590981905, 33.65937500034139873, -29.30972558990011478 ) ) ;
#15350=LINE ( 'NONE', #5151, #10614 ) ;
#15351=CARTESIAN_POINT ( 'NONE',  ( -15.40903463028481646, 47.52187500034139589, -47.42413220539093999 ) ) ;
#15358=EDGE_CURVE ( 'NONE', #5867, #4422, #2669, .T. ) ;
#15364=CARTESIAN_POINT ( 'NONE',  ( -3.111920190527341144E-15, 35.28125000068280315, -50.00000000000000000 ) ) ;
#15365=CARTESIAN_POINT ( 'NONE',  ( 7.919222016226875382, 39.22999571913595673, -49.99999999999997158 ) ) ;
#15368=CARTESIAN_POINT ( 'NONE',  ( -15.40903463028480580, 48.25937500034140015, 47.42413220539094709 ) ) ;
#15373=CARTESIAN_POINT ( 'NONE',  ( 9.657523855033129090E-15, 38.28125000068279604, 52.57311121191334990 ) ) ;
#15383=CARTESIAN_POINT ( 'NONE',  ( 50.00000000000000711, 42.68125000068280173, 16.24598481164530739 ) ) ;
#15386=ORIENTED_EDGE ( 'NONE', *, *, #14987, .F. ) ;
#15387=CARTESIAN_POINT ( 'NONE',  ( 0.000000000000000000, 20.00000000000000355, 0.000000000000000000 ) ) ;
#15388=CARTESIAN_POINT ( 'NONE',  ( -16.94841605670512052, 27.00700085982962051, 93.71793596878799804 ) ) ;
#15391=( BOUNDED_CURVE ( )  B_SPLINE_CURVE ( 2, ( #1643, #9225, #9305, #9134, #2901, #13117, #15524, #1566, #308, #6740, #14279, #15443, #5407 ),
 .UNSPECIFIED., .F., .F. ) 
 B_SPLINE_CURVE_WITH_KNOTS ( ( 3, 2, 2, 2, 2, 2, 3 ),
 ( 0.1833333333333333481, 0.1866666666666666752, 0.1933333333333333293, 0.2000000000000000111, 0.2066666666666666652, 0.2133333333333333470, 0.2166666666666666741 ),
 .UNSPECIFIED. ) 
 CURVE ( )  GEOMETRIC_REPRESENTATION_ITEM ( )  RATIONAL_B_SPLINE_CURVE ( ( 0.9755282581475767101, 0.9755282581475768211, 1.000000000000000000, 0.9510565162951535312, 1.000000000000000000, 0.9510565162951535312, 1.000000000000000000, 0.9510565162951535312, 1.000000000000000000, 0.9510565162951535312, 1.000000000000000000, 0.9755282581475768211, 0.9755282581475768211 ) ) 
 REPRESENTATION_ITEM ( '' )  );
#15392=CARTESIAN_POINT ( 'NONE',  ( -1.240322475938754499E-13, 38.28125000068280315, 50.00000000000000000 ) ) ;
#15394=CARTESIAN_POINT ( 'NONE',  ( -30.81806926056962226, 22.15937500034139163, 42.41743335407647209 ) ) ;
#15397=CARTESIAN_POINT ( 'NONE',  ( -49.86468353125000164, 31.92187500034139447, 0.000000000000000000 ) ) ;
#15399=CARTESIAN_POINT ( 'NONE',  ( -40.45084971874737079, 28.20000000000000284, 29.38926261462367151 ) ) ;
#15401=CARTESIAN_POINT ( 'NONE',  ( 40.34137639590981195, 33.05937500034139731, -29.30972558990011834 ) ) ;
#15411=DIRECTION ( 'NONE',  ( 0.000000000000000000, 0.000000000000000000, 1.000000000000000000 ) ) ;
#15413=CARTESIAN_POINT ( 'NONE',  ( 40.34137639590981905, 34.72187500034139873, 29.30972558990010768 ) ) ;
#15414=CARTESIAN_POINT ( 'NONE',  ( -49.86468353124999453, 39.95937500034139589, 16.20201782572377169 ) ) ;
#15417=CARTESIAN_POINT ( 'NONE',  ( -49.99999999999999289, 23.68125000068279462, -16.24598481164531449 ) ) ;
#15418=CARTESIAN_POINT ( 'NONE',  ( 12.00283417906081773, 35.24790003054248899, 93.01444432686068353 ) ) ;
#15419=CARTESIAN_POINT ( 'NONE',  ( -49.86468353124999453, 26.02187500034139944, 16.20201782572377525 ) ) ;
#15426=CARTESIAN_POINT ( 'NONE',  ( -50.00000000000000000, 24.00000000000000000, 0.000000000000000000 ) ) ;
#15428=CARTESIAN_POINT ( 'NONE',  ( 49.86468353125001585, 26.75937500034139660, 16.20201782572375038 ) ) ;
#15431=CARTESIAN_POINT ( 'NONE',  ( 15.40903463028482356, 44.52187500034139589, 47.42413220539093999 ) ) ;
#15434=FACE_OUTER_BOUND ( 'NONE', #10264, .T. ) ;
#15439=ORIENTED_EDGE ( 'NONE', *, *, #1549, .F. ) ;
#15440=LINE ( 'NONE', #2721, #11848 ) ;
#15441=ORIENTED_EDGE ( 'NONE', *, *, #6942, .T. ) ;
#15443=CARTESIAN_POINT ( 'NONE',  ( -7.919222016226816763, 43.33250428222963535, -49.99999999999999289 ) ) ;
#15447=CARTESIAN_POINT ( 'NONE',  ( -49.99999999999999289, 27.89999999999999858, -16.24598481164531449 ) ) ;
#15448=CARTESIAN_POINT ( 'NONE',  ( 49.86468353125000164, 48.85937500034139447, -6.106662507704105588E-15 ) ) ;
#15449=CARTESIAN_POINT ( 'NONE',  ( -15.45084971874737256, 25.38125000068279746, -47.55282581475767500 ) ) ;
#15451=CARTESIAN_POINT ( 'NONE',  ( -3.210462471511496205E-15, 23.42187500034139802, -52.43083105670540789 ) ) ;
#15454=CARTESIAN_POINT ( 'NONE',  ( -50.00000000000000000, 41.78125000068280315, 0.000000000000000000 ) ) ;
#15472=CARTESIAN_POINT ( 'NONE',  ( 5.716386541834933332, 5.919903133645938453, 98.79670695971100258 ) ) ;
#15473=CARTESIAN_POINT ( 'NONE',  ( -46.85365039762112360, 20.00000000000000355, 17.06523097087215390 ) ) ;
#15474=CARTESIAN_POINT ( 'NONE',  ( 40.34137639590981195, 27.12187500034139731, -29.30972558990011834 ) ) ;
#15476=CARTESIAN_POINT ( 'NONE',  ( 50.00000000000000711, 28.89999999999999858, 16.24598481164530739 ) ) ;
#15477=CARTESIAN_POINT ( 'NONE',  ( -49.86468353124999453, 33.75937500034140015, -16.20201782572375393 ) ) ;
#15480=CARTESIAN_POINT ( 'NONE',  ( 30.90169943749473802, 39.30000000000000426, -42.53254041760200721 ) ) ;
#15486=( BOUNDED_CURVE ( )  B_SPLINE_CURVE ( 2, ( #6836, #9480, #6672, #15626, #4251, #9317, #14204, #4075, #8147, #5585, #639, #11721, #14528 ),
 .UNSPECIFIED., .F., .F. ) 
 B_SPLINE_CURVE_WITH_KNOTS ( ( 3, 2, 2, 2, 2, 2, 3 ),
 ( 0.9500000000000000666, 0.9533333333333333659, 0.9599999999999999645, 0.9666666666666666741, 0.9733333333333333837, 0.9799999999999999822, 0.9833333333333333925 ),
 .UNSPECIFIED. ) 
 CURVE ( )  GEOMETRIC_REPRESENTATION_ITEM ( )  RATIONAL_B_SPLINE_CURVE ( ( 0.9755282581475768211, 0.9755282581475771542, 1.000000000000000000, 0.9510565162951535312, 1.000000000000000000, 0.9510565162951535312, 1.000000000000000000, 0.9510565162951535312, 1.000000000000000000, 0.9510565162951535312, 1.000000000000000000, 0.9755282581475763770, 0.9755282581475768211 ) ) 
 REPRESENTATION_ITEM ( '' )  );
#15490=CARTESIAN_POINT ( 'NONE',  ( 40.34137639590981905, 36.72187500034139163, 29.30972558990010768 ) ) ;
#15491=CARTESIAN_POINT ( 'NONE',  ( -3.210462471511496205E-15, 43.35937500034139447, -52.43083105670540789 ) ) ;
#15495=CARTESIAN_POINT ( 'NONE',  ( -40.34137639590981905, 49.65937500034139873, -29.30972558990011478 ) ) ;
#15497=CARTESIAN_POINT ( 'NONE',  ( -30.81806926056963292, 29.62187500034139376, -42.41743335407647209 ) ) ;
#15505=CARTESIAN_POINT ( 'NONE',  ( 15.45084971874736723, 31.18125000068279817, -47.55282581475768211 ) ) ;
#15507=CARTESIAN_POINT ( 'NONE',  ( 30.81806926056962936, 25.15937500034139518, -42.41743335407647209 ) ) ;
#15508=CARTESIAN_POINT ( 'NONE',  ( 0.000000000000000000, 20.00000000000000355, 0.000000000000000000 ) ) ;
#15510=CARTESIAN_POINT ( 'NONE',  ( 49.86468353125001585, 42.82187500034139305, 16.20201782572375038 ) ) ;
#15513=CARTESIAN_POINT ( 'NONE',  ( 49.86468353124999453, 47.02187500034139589, -16.20201782572376459 ) ) ;
#15517=VERTEX_POINT ( 'NONE', #1753 ) ;
#15523=ADVANCED_FACE ( 'NONE', ( #1829 ), #9251, .F. ) ;
#15524=CARTESIAN_POINT ( 'NONE',  ( -50.00000000000000000, 43.78125000068280315, 0.000000000000000000 ) ) ;
#15527=CARTESIAN_POINT ( 'NONE',  ( 40.45084971874737789, 26.80000000000000071, 29.38926261462365375 ) ) ;
#15528=CARTESIAN_POINT ( 'NONE',  ( 15.40903463028481113, 47.25937500034140015, -47.42413220539094709 ) ) ;
#15535=CARTESIAN_POINT ( 'NONE',  ( 50.00000000000000000, 42.78125000068280315, -6.123233995736766085E-15 ) ) ;
#15554=DIRECTION ( 'NONE',  ( 0.000000000000000000, 0.000000000000000000, 1.000000000000000000 ) ) ;
#15559=CARTESIAN_POINT ( 'NONE',  ( 9.341593500131070371, 7.690831593539996902, 98.20175713279056140 ) ) ;
#15561=CARTESIAN_POINT ( 'NONE',  ( 15.40903463028482356, 28.52187500034139589, 47.42413220539093999 ) ) ;
#15565=CARTESIAN_POINT ( 'NONE',  ( -49.86468353124999453, 29.75937500034139305, -16.20201782572375393 ) ) ;
#15570=CARTESIAN_POINT ( 'NONE',  ( 7.919222016226875382, 39.44874571845315359, -49.99999999999997158 ) ) ;
#15582=CARTESIAN_POINT ( 'NONE',  ( 49.86468353125001585, 32.82187500034139305, 16.20201782572375038 ) ) ;
#15583=CARTESIAN_POINT ( 'NONE',  ( 30.81806926056962936, 35.15937500034139873, -42.41743335407646498 ) ) ;
#15586=CARTESIAN_POINT ( 'NONE',  ( 49.86468353125001585, 48.75937500034140015, 16.20201782572375038 ) ) ;
#15588=CARTESIAN_POINT ( 'NONE',  ( -49.86468353124999453, 25.82187500034139305, -16.20201782572375393 ) ) ;
#15593=CARTESIAN_POINT ( 'NONE',  ( -30.90169943749473447, 28.08125000068280031, 42.53254041760200721 ) ) ;
#15594=ORIENTED_EDGE ( 'NONE', *, *, #14886, .T. ) ;
#15602=CARTESIAN_POINT ( 'NONE',  ( -49.86468353124999453, 25.75937500034140015, -16.20201782572375393 ) ) ;
#15604=CARTESIAN_POINT ( 'NONE',  ( -15.40903463028481646, 39.52187500034139589, -47.42413220539093999 ) ) ;
#15607=CARTESIAN_POINT ( 'NONE',  ( 15.40903463028482356, 44.52187500034139589, 47.42413220539093999 ) ) ;
#15612=CARTESIAN_POINT ( 'NONE',  ( -3.111920190527341144E-15, 45.28125000068279604, -50.00000000000000000 ) ) ;
#15614=CARTESIAN_POINT ( 'NONE',  ( -1.240322475938754499E-13, 36.50000000000000711, 50.00000000000000000 ) ) ;
#15616=CARTESIAN_POINT ( 'NONE',  ( 40.45084971874737789, 22.80000000000000071, 29.38926261462365375 ) ) ;
#15617=CARTESIAN_POINT ( 'NONE',  ( 30.81806926056962936, 45.15937500034139873, -42.41743335407647209 ) ) ;
#15618=CARTESIAN_POINT ( 'NONE',  ( 1.293669679204937499E-13, 37.28125000068280315, -50.00000000000000000 ) ) ;
#15623=CARTESIAN_POINT ( 'NONE',  ( 0.000000000000000000, 28.00000000000000355, 0.000000000000000000 ) ) ;
#15624=CARTESIAN_POINT ( 'NONE',  ( -15.45084971874737256, 39.38125000068279746, -47.55282581475767500 ) ) ;
#15626=CARTESIAN_POINT ( 'NONE',  ( 30.90169943749473802, 21.08125000068279675, -42.53254041760200721 ) ) ;
#15628=ORIENTED_EDGE ( 'NONE', *, *, #3788, .F. ) ;
#15632=DIRECTION ( 'NONE',  ( -0.000000000000000000, 1.000000000000000000, -0.000000000000000000 ) ) ;
#15634=CARTESIAN_POINT ( 'NONE',  ( 0.000000000000000000, 0.000000000000000000, 0.000000000000000000 ) ) ;
#15635=( BOUNDED_CURVE ( )  B_SPLINE_CURVE ( 2, ( #63, #5090, #12879, #11394, #7482, #16459, #11467, #1316, #7563, #6240, #5169, #10065, #14037 ),
 .UNSPECIFIED., .F., .F. ) 
 B_SPLINE_CURVE_WITH_KNOTS ( ( 3, 2, 2, 2, 2, 2, 3 ),
 ( 0.5500000000000000444, 0.5533333333333333437, 0.5600000000000000533, 0.5666666666666666519, 0.5733333333333333615, 0.5799999999999999600, 0.5833333333333333703 ),
 .UNSPECIFIED. ) 
 CURVE ( )  GEOMETRIC_REPRESENTATION_ITEM ( )  RATIONAL_B_SPLINE_CURVE ( ( 0.9755282581475768211, 0.9755282581475771542, 1.000000000000000000, 0.9510565162951535312, 1.000000000000000000, 0.9510565162951535312, 1.000000000000000000, 0.9510565162951535312, 1.000000000000000000, 0.9510565162951535312, 1.000000000000000000, 0.9755282581475763770, 0.9755282581475768211 ) ) 
 REPRESENTATION_ITEM ( '' )  );
#15642=CARTESIAN_POINT ( 'NONE',  ( -40.45084971874737789, 37.58125000068280031, -29.38926261462365730 ) ) ;
#15643=CYLINDRICAL_SURFACE ( 'NONE', #9659, 10.00000000000000000 ) ;
#15645=CARTESIAN_POINT ( 'NONE',  ( 40.34137639590981905, 28.72187500034139873, 29.30972558990010768 ) ) ;
#15649=CARTESIAN_POINT ( 'NONE',  ( 30.81806926056964002, 34.55937500034139731, 42.41743335407647209 ) ) ;
#15651=ORIENTED_EDGE ( 'NONE', *, *, #13724, .T. ) ;
#15657=VECTOR ( 'NONE', #11789, 1000.000000000000000 ) ;
#15663=CARTESIAN_POINT ( 'NONE',  ( 40.34137639590981905, 38.72187500034139873, 29.30972558990010768 ) ) ;
#15664=CARTESIAN_POINT ( 'NONE',  ( -40.34137639590981905, 33.65937500034139873, -29.30972558990011478 ) ) ;
#15668=CARTESIAN_POINT ( 'NONE',  ( -15.45084971874737256, 21.38125000068279746, -47.55282581475767500 ) ) ;
#15670=CARTESIAN_POINT ( 'NONE',  ( 49.86468353125000164, 28.92187500034139802, -6.106662507704105588E-15 ) ) ;
#15678=CARTESIAN_POINT ( 'NONE',  ( -30.81806926056962226, 26.15937500034139163, 42.41743335407647919 ) ) ;
#15679=CARTESIAN_POINT ( 'NONE',  ( 49.86468353124999453, 41.02187500034139589, -16.20201782572376104 ) ) ;
#15682=CARTESIAN_POINT ( 'NONE',  ( 40.45084971874737789, 30.80000000000000071, 29.38926261462365375 ) ) ;
#15688=DIRECTION ( 'NONE',  ( -0.000000000000000000, -1.000000000000000000, -0.000000000000000000 ) ) ;
#15689=CARTESIAN_POINT ( 'NONE',  ( 30.90169943749473802, 39.08125000068280031, -42.53254041760200721 ) ) ;
#15690=DIRECTION ( 'NONE',  ( 0.000000000000000000, 0.000000000000000000, -1.000000000000000000 ) ) ;
#15691=CARTESIAN_POINT ( 'NONE',  ( -15.45084971874736368, 26.40000000000000213, 47.55282581475768211 ) ) ;
#15692=CARTESIAN_POINT ( 'NONE',  ( -49.86468353124999453, 43.95937500034138878, 16.20201782572377525 ) ) ;
#15694=CARTESIAN_POINT ( 'NONE',  ( 0.000000000000000000, 50.00000000000000000, 0.000000000000000000 ) ) ;
#15698=CARTESIAN_POINT ( 'NONE',  ( -40.45084971874737789, 35.58125000068279320, -29.38926261462365730 ) ) ;
#15700=CARTESIAN_POINT ( 'NONE',  ( 30.90169943749473802, 23.08125000068279675, -42.53254041760200721 ) ) ;
#15701=ADVANCED_FACE ( 'NONE', ( #9496 ), #14790, .T. ) ;
#15717=CARTESIAN_POINT ( 'NONE',  ( -47.24032962522632317, 20.00000000000000355, 15.96451374291463310 ) ) ;
#15718=CARTESIAN_POINT ( 'NONE',  ( -30.81806926056963292, 21.62187500034139376, -42.41743335407646498 ) ) ;
#15721=CARTESIAN_POINT ( 'NONE',  ( -3.210462471511496205E-15, 35.35937500034140157, -52.43083105670540789 ) ) ;
#15724=( BOUNDED_CURVE ( )  B_SPLINE_CURVE ( 2, ( #5679, #14799, #3433, #12155, #5930, #8494, #7175, #13558, #4439, #3514, #5848, #14553, #9586 ),
 .UNSPECIFIED., .F., .F. ) 
 B_SPLINE_CURVE_WITH_KNOTS ( ( 3, 2, 2, 2, 2, 2, 3 ),
 ( 0.6500000000000000222, 0.6533333333333333215, 0.6600000000000000311, 0.6666666666666666297, 0.6733333333333333393, 0.6800000000000000488, 0.6833333333333333481 ),
 .UNSPECIFIED. ) 
 CURVE ( )  GEOMETRIC_REPRESENTATION_ITEM ( )  RATIONAL_B_SPLINE_CURVE ( ( 0.9755282581475768211, 0.9755282581475771542, 1.000000000000000000, 0.9510565162951535312, 1.000000000000000000, 0.9510565162951535312, 1.000000000000000000, 0.9510565162951535312, 1.000000000000000000, 0.9510565162951535312, 1.000000000000000000, 0.9755282581475768211, 0.9755282581475768211 ) ) 
 REPRESENTATION_ITEM ( '' )  );
#15727=VERTEX_POINT ( 'NONE', #15887 ) ;
#15732=CARTESIAN_POINT ( 'NONE',  ( 49.86468353125001585, 38.82187500034140015, 16.20201782572375038 ) ) ;
#15733=CARTESIAN_POINT ( 'NONE',  ( 49.86468353124999453, 36.95937500034139589, -16.20201782572376104 ) ) ;
#15738=EDGE_CURVE ( 'NONE', #2027, #15007, #14701, .T. ) ;
#15739=CARTESIAN_POINT ( 'NONE',  ( -50.00000000000000000, 21.78125000068279959, 0.000000000000000000 ) ) ;
#15741=CARTESIAN_POINT ( 'NONE',  ( 9.631387414534489405E-15, 30.42187500034139447, 52.43083105670540789 ) ) ;
#15749=ADVANCED_FACE ( 'NONE', ( #1988 ), #654, .F. ) ;
#15753=CARTESIAN_POINT ( 'NONE',  ( 40.34137639590981905, 24.65937500034139873, 29.30972558990010768 ) ) ;
#15755=EDGE_CURVE ( 'NONE', #12890, #6301, #610, .T. ) ;
#15757=CARTESIAN_POINT ( 'NONE',  ( 50.00000000000000711, 34.89999999999998437, 16.24598481164530739 ) ) ;
#15759=VECTOR ( 'NONE', #7712, 1000.000000000000227 ) ;
#15760=CARTESIAN_POINT ( 'NONE',  ( -49.86468353124999453, 49.82187500034140015, -16.20201782572375393 ) ) ;
#15761=CARTESIAN_POINT ( 'NONE',  ( 2.600676159226420495E-13, 31.49999999999999289, -49.99999999999999289 ) ) ;
#15762=ORIENTED_EDGE ( 'NONE', *, *, #12093, .F. ) ;
#15767=ADVANCED_FACE ( 'NONE', ( #13550 ), #14159, .T. ) ;
#15772=CARTESIAN_POINT ( 'NONE',  ( 40.45084971874737079, 36.98125000068279888, -29.38926261462366440 ) ) ;
#15773=CARTESIAN_POINT ( 'NONE',  ( -40.34137639590981905, 43.65937500034139163, -29.30972558990011478 ) ) ;
#15800=CARTESIAN_POINT ( 'NONE',  ( 16.61632465174088580, 16.89218409470073468, 95.58913275680403387 ) ) ;
#15801=CARTESIAN_POINT ( 'NONE',  ( -47.98103867763168040, 19.99999999999999645, 13.57697939761855643 ) ) ;
#15802=CARTESIAN_POINT ( 'NONE',  ( -40.34137639590981195, 20.12187500034139731, 29.30972558990012189 ) ) ;
#15805=CARTESIAN_POINT ( 'NONE',  ( -30.81806926056963292, 25.55937500034139376, -42.41743335407647209 ) ) ;
#15807=EDGE_LOOP ( 'NONE', ( #4879, #5737, #5659, #15762 ) ) ;
#15812=AXIS2_PLACEMENT_3D ( 'NONE', #2158, #11073, #8560 ) ;
#15818=CARTESIAN_POINT ( 'NONE',  ( -40.34137639590981905, 29.72187500034139518, -29.30972558990011478 ) ) ;
#15819=CARTESIAN_POINT ( 'NONE',  ( -30.81806926056962226, 34.15937500034139163, 42.41743335407647209 ) ) ;
#15826=CARTESIAN_POINT ( 'NONE',  ( -40.34137639590981195, 48.05937500034139731, 29.30972558990012189 ) ) ;
#15830=CARTESIAN_POINT ( 'NONE',  ( 40.45084971874737789, 48.80000000000000426, 29.38926261462365375 ) ) ;
#15832=EDGE_LOOP ( 'NONE', ( #10555, #7102 ) ) ;
#15841=CARTESIAN_POINT ( 'NONE',  ( 40.45084971874737789, 44.58125000068280031, 29.38926261462365375 ) ) ;
#15843=CARTESIAN_POINT ( 'NONE',  ( 15.45084971874737789, 30.38125000068280102, 47.55282581475767500 ) ) ;
#15845=CARTESIAN_POINT ( 'NONE',  ( 40.34137639590981195, 47.12187500034140442, -29.30972558990011834 ) ) ;
#15849=SHAPE_DEFINITION_REPRESENTATION ( #547, #9477 ) ;
#15850=CARTESIAN_POINT ( 'NONE',  ( -40.45084971874737079, 40.20000000000000284, 29.38926261462367151 ) ) ;
#15852=CARTESIAN_POINT ( 'NONE',  ( 49.86468353124999453, 41.02187500034139589, -16.20201782572376459 ) ) ;
#15854=VERTEX_POINT ( 'NONE', #905 ) ;
#15860=CARTESIAN_POINT ( 'NONE',  ( 1.293669679204937499E-13, 39.28125000068280315, -50.00000000000000000 ) ) ;
#15865=CARTESIAN_POINT ( 'NONE',  ( -30.81806926056963292, 43.55937500034139731, -42.41743335407647209 ) ) ;
#15867=CARTESIAN_POINT ( 'NONE',  ( 15.45084971874737789, 24.60000000000000142, 47.55282581475767500 ) ) ;
#15869=CARTESIAN_POINT ( 'NONE',  ( 6.123233995736766085E-15, 20.00000000000000355, -50.00000000000000000 ) ) ;
#15887=CARTESIAN_POINT ( 'NONE',  ( -45.11452830843730766, 20.00000000000000711, 21.24066852005664430 ) ) ;
#15889=CARTESIAN_POINT ( 'NONE',  ( 8.446640517145639571E-15, 48.49999999999999289, 50.00000000000000000 ) ) ;
#15893=CARTESIAN_POINT ( 'NONE',  ( -40.34137639590981905, 21.72187500034139518, -29.30972558990011478 ) ) ;
#15896=CARTESIAN_POINT ( 'NONE',  ( -30.81806926056963292, 23.55937500034139376, -42.41743335407647209 ) ) ;
#15899=EDGE_LOOP ( 'NONE', ( #3568, #13699 ) ) ;
#15900=UNCERTAINTY_MEASURE_WITH_UNIT (LENGTH_MEASURE( 1.000000000000000082E-05 ), #12392, 'distance_accuracy_value', 'NONE');
#15905=CARTESIAN_POINT ( 'NONE',  ( 40.45084971874737079, 28.98125000068279888, -29.38926261462366440 ) ) ;
#15907=CARTESIAN_POINT ( 'NONE',  ( 15.40903463028482356, 26.52187500034139589, 47.42413220539093999 ) ) ;
#15908=CARTESIAN_POINT ( 'NONE',  ( 15.40903463028481113, 33.25937500034140015, -47.42413220539094709 ) ) ;
#15909=CARTESIAN_POINT ( 'NONE',  ( -15.45084971874736368, 36.39999999999999858, 47.55282581475768211 ) ) ;
#15911=DIRECTION ( 'NONE',  ( -0.000000000000000000, -1.000000000000000000, -0.000000000000000000 ) ) ;
#15912=CARTESIAN_POINT ( 'NONE',  ( 40.34137639590981905, 42.65937500034139873, 29.30972558990010768 ) ) ;
#15915=CARTESIAN_POINT ( 'NONE',  ( -15.40903463028481646, 21.52187500034139589, -47.42413220539093999 ) ) ;
#15917=ORIENTED_EDGE ( 'NONE', *, *, #2914, .F. ) ;
#15925=CARTESIAN_POINT ( 'NONE',  ( -49.86468353125000164, 45.92187500034139447, 0.000000000000000000 ) ) ;
#15929=CARTESIAN_POINT ( 'NONE',  ( 40.45084971874737079, 37.20000000000000284, -29.38926261462366440 ) ) ;
#15930=CARTESIAN_POINT ( 'NONE',  ( 49.86468353125000164, 42.92187500034140157, -6.106662507704105588E-15 ) ) ;
#15936=VERTEX_POINT ( 'NONE', #12721 ) ;
#15940=CARTESIAN_POINT ( 'NONE',  ( -15.45084971874737256, 21.60000000000000142, -47.55282581475767500 ) ) ;
#15941=CARTESIAN_POINT ( 'NONE',  ( 30.81806926056962936, 39.15937500034139873, -42.41743335407647209 ) ) ;
#15942=CARTESIAN_POINT ( 'NONE',  ( -40.34137639590981195, 48.05937500034139731, 29.30972558990012189 ) ) ;
#15946=DIRECTION ( 'NONE',  ( 0.000000000000000000, 0.000000000000000000, 1.000000000000000000 ) ) ;
#15948=CARTESIAN_POINT ( 'NONE',  ( 7.919222016226875382, 41.44874571845315359, -49.99999999999997158 ) ) ;
#15952=VERTEX_POINT ( 'NONE', #8980 ) ;
#15954=VERTEX_POINT ( 'NONE', #16380 ) ;
#15957=CARTESIAN_POINT ( 'NONE',  ( -7.919222016226752814, 39.55125428154683931, -50.00000000000000711 ) ) ;
#15958=CARTESIAN_POINT ( 'NONE',  ( 50.00000000000000000, 29.00000000000000000, -6.123233995736766085E-15 ) ) ;
#15964=DIRECTION ( 'NONE',  ( 0.000000000000000000, 0.000000000000000000, 1.000000000000000000 ) ) ;
#15966=CARTESIAN_POINT ( 'NONE',  ( -2.547328955960238000E-13, 20.28125000068279959, 49.99999999999999289 ) ) ;
#15969=CARTESIAN_POINT ( 'NONE',  ( -15.40903463028481646, 21.52187500034139589, -47.42413220539093999 ) ) ;
#15973=CARTESIAN_POINT ( 'NONE',  ( 49.86468353124999453, 28.95937500034139944, -16.20201782572376459 ) ) ;
#15975=ORIENTED_EDGE ( 'NONE', *, *, #5840, .F. ) ;
#15982=CARTESIAN_POINT ( 'NONE',  ( 6.123233995736766085E-15, 20.00000000000000355, -50.00000000000000000 ) ) ;
#15983=CARTESIAN_POINT ( 'NONE',  ( -15.40903463028481646, 29.52187500034139589, -47.42413220539093999 ) ) ;
#15984=CARTESIAN_POINT ( 'NONE',  ( 40.34137639590981905, 28.65937500034139873, 29.30972558990010768 ) ) ;
#15989=CARTESIAN_POINT ( 'NONE',  ( 49.86468353124999453, 46.95937500034139589, -16.20201782572376459 ) ) ;
#15992=CARTESIAN_POINT ( 'NONE',  ( -30.81806926056962226, 20.22187500034139163, 42.41743335407647919 ) ) ;
#15998=VECTOR ( 'NONE', #12191, 1000.000000000000000 ) ;
#15999=CARTESIAN_POINT ( 'NONE',  ( -15.45084971874737256, 33.38125000068280457, -47.55282581475767500 ) ) ;
#16002=CARTESIAN_POINT ( 'NONE',  ( -40.34137639590981905, 45.72187500034139873, -29.30972558990011478 ) ) ;
#16006=CARTESIAN_POINT ( 'NONE',  ( 30.90169943749474157, 37.08125000068279320, -42.53254041760200721 ) ) ;
#16007=CARTESIAN_POINT ( 'NONE',  ( -15.45084971874736368, 38.40000000000000568, 47.55282581475768211 ) ) ;
#16008=CARTESIAN_POINT ( 'NONE',  ( -30.81806926056962226, 38.22187500034139873, 42.41743335407647919 ) ) ;
#16009=CARTESIAN_POINT ( 'NONE',  ( 50.00000000000000711, 30.89999999999999858, 16.24598481164530739 ) ) ;
#16015=ORIENTED_EDGE ( 'NONE', *, *, #6562, .T. ) ;
#16019=CARTESIAN_POINT ( 'NONE',  ( 40.45084971874737079, 27.20000000000000284, -29.38926261462366440 ) ) ;
#16021=CARTESIAN_POINT ( 'NONE',  ( 9.631387414534489405E-15, 40.35937500034139447, 52.43083105670540789 ) ) ;
#16022=CARTESIAN_POINT ( 'NONE',  ( -40.34137639590981905, 49.65937500034139873, -29.30972558990011478 ) ) ;
#16023=CARTESIAN_POINT ( 'NONE',  ( 40.45084971874737789, 24.80000000000000426, 29.38926261462365375 ) ) ;
#16027=CARTESIAN_POINT ( 'NONE',  ( 30.90169943749475223, 40.69999999999999574, 42.53254041760199300 ) ) ;
#16032=EDGE_CURVE ( 'NONE', #2741, #6400, #4377, .T. ) ;
#16034=ORIENTED_EDGE ( 'NONE', *, *, #12294, .T. ) ;
#16038=CARTESIAN_POINT ( 'NONE',  ( 50.00000000000000711, 28.89999999999999858, 16.24598481164530739 ) ) ;
#16045=CARTESIAN_POINT ( 'NONE',  ( 2.600676159226420495E-13, 31.49999999999999289, -49.99999999999999289 ) ) ;
#16047=ADVANCED_FACE ( 'NONE', ( #14198 ), #2980, .F. ) ;
#16048=CARTESIAN_POINT ( 'NONE',  ( -45.25922935877468944, 20.00000000000001776, 20.93126818148126489 ) ) ;
#16049=CARTESIAN_POINT ( 'NONE',  ( -30.81806926056962226, 20.22187500034139518, 42.41743335407647209 ) ) ;
#16053=CARTESIAN_POINT ( 'NONE',  ( 49.86468353125001585, 26.75937500034139660, 16.20201782572375038 ) ) ;
#16054=CARTESIAN_POINT ( 'NONE',  ( -49.99999999999999289, 41.68125000068280173, -16.24598481164531449 ) ) ;
#16066=CARTESIAN_POINT ( 'NONE',  ( 9.631387414534489405E-15, 28.42187500034139092, 52.43083105670540789 ) ) ;
#16067=CARTESIAN_POINT ( 'NONE',  ( -40.34137639590981905, 27.65937500034139873, -29.30972558990011478 ) ) ;
#16070=FACE_OUTER_BOUND ( 'NONE', #15078, .T. ) ;
#16072=CARTESIAN_POINT ( 'NONE',  ( -49.86468353124999453, 47.95937500034138878, 16.20201782572377525 ) ) ;
#16076=CARTESIAN_POINT ( 'NONE',  ( 30.81806926056962936, 21.22187500034139518, -42.41743335407647209 ) ) ;
#16089=CARTESIAN_POINT ( 'NONE',  ( -40.34137639590981195, 48.12187500034139731, 29.30972558990012189 ) ) ;
#16094=CARTESIAN_POINT ( 'NONE',  ( -49.99999999999999289, 35.88125000068279746, 16.24598481164533226 ) ) ;
#16096=CARTESIAN_POINT ( 'NONE',  ( -49.86468353125000164, 39.92187500034139447, 0.000000000000000000 ) ) ;
#16109=CARTESIAN_POINT ( 'NONE',  ( 40.45084971874737789, 36.58125000068280031, 29.38926261462365375 ) ) ;
#16111=CARTESIAN_POINT ( 'NONE',  ( -40.34137639590981905, 37.65937500034139873, -29.30972558990011478 ) ) ;
#16113=CARTESIAN_POINT ( 'NONE',  ( 49.86468353124999453, 48.95937500034140299, -16.20201782572376104 ) ) ;
#16114=EDGE_CURVE ( 'NONE', #15191, #40, #16262, .T. ) ;
#16116=AXIS2_PLACEMENT_3D ( 'NONE', #11728, #2996, #8157 ) ;
#16121=CARTESIAN_POINT ( 'NONE',  ( 49.99999999999999289, 37.10000000000000142, -16.24598481164532160 ) ) ;
#16127=VERTEX_POINT ( 'NONE', #15618 ) ;
#16132=CYLINDRICAL_SURFACE ( 'NONE', #7620, 50.00000000000000000 ) ;
#16133=CARTESIAN_POINT ( 'NONE',  ( 30.90169943749475223, 28.70000000000000284, 42.53254041760199300 ) ) ;
#16134=ORIENTED_EDGE ( 'NONE', *, *, #14044, .F. ) ;
#16135=CARTESIAN_POINT ( 'NONE',  ( -15.45084971874737256, 47.38125000068279746, -47.55282581475767500 ) ) ;
#16138=DIRECTION ( 'NONE',  ( 1.000000000000000000, 0.000000000000000000, -0.000000000000000000 ) ) ;
#16143=CARTESIAN_POINT ( 'NONE',  ( 9.657523855033129090E-15, 46.28125000068279604, 52.57311121191334990 ) ) ;
#16146=CARTESIAN_POINT ( 'NONE',  ( 40.34137639590981905, 28.65937500034139873, 29.30972558990010768 ) ) ;
#16150=CARTESIAN_POINT ( 'NONE',  ( 40.45084971874737079, 45.20000000000000284, -29.38926261462366440 ) ) ;
#16158=CARTESIAN_POINT ( 'NONE',  ( 15.40903463028481113, 31.32187500034139305, -47.42413220539094709 ) ) ;
#16159=CARTESIAN_POINT ( 'NONE',  ( 40.34137639590981905, 32.65937500034139873, 29.30972558990010768 ) ) ;
#16160=CARTESIAN_POINT ( 'NONE',  ( -50.00000000000000000, 36.00000000000000711, 0.000000000000000000 ) ) ;
#16161=CARTESIAN_POINT ( 'NONE',  ( -49.86468353125000164, 33.92187500034139447, 0.000000000000000000 ) ) ;
#16164=CARTESIAN_POINT ( 'NONE',  ( 49.86468353124999453, 42.95937500034139589, -16.20201782572376459 ) ) ;
#16167=CARTESIAN_POINT ( 'NONE',  ( 30.90169943749475578, 44.69999999999999574, 42.53254041760200010 ) ) ;
#16175=DIRECTION ( 'NONE',  ( -0.000000000000000000, 1.000000000000000000, -0.000000000000000000 ) ) ;
#16177=EDGE_CURVE ( 'NONE', #15517, #4175, #12281, .T. ) ;
#16178=CARTESIAN_POINT ( 'NONE',  ( 49.86468353125001585, 48.82187500034139305, 16.20201782572375038 ) ) ;
#16181=CARTESIAN_POINT ( 'NONE',  ( 50.00000000000000000, 32.78125000068279604, -6.123233995736766085E-15 ) ) ;
#16183=CARTESIAN_POINT ( 'NONE',  ( 15.40903463028482356, 40.52187500034139589, 47.42413220539093999 ) ) ;
#16188=VERTEX_POINT ( 'NONE', #14767 ) ;
#16189=ORIENTED_EDGE ( 'NONE', *, *, #1424, .T. ) ;
#16193=CARTESIAN_POINT ( 'NONE',  ( 50.00000000000000000, 27.00000000000000355, -6.123233995736766085E-15 ) ) ;
#16194=DIRECTION ( 'NONE',  ( 0.000000000000000000, 0.000000000000000000, 1.000000000000000000 ) ) ;
#16196=CARTESIAN_POINT ( 'NONE',  ( 30.81806926056964002, 38.55937500034140442, 42.41743335407647209 ) ) ;
#16197=CARTESIAN_POINT ( 'NONE',  ( -15.40903463028481646, 43.45937500034139589, -47.42413220539093999 ) ) ;
#16200=CARTESIAN_POINT ( 'NONE',  ( 49.99999999999999289, 41.10000000000000142, -16.24598481164532160 ) ) ;
#16218=CARTESIAN_POINT ( 'NONE',  ( 40.45084971874737789, 46.80000000000000426, 29.38926261462365375 ) ) ;
#16219=CARTESIAN_POINT ( 'NONE',  ( 15.45084971874737789, 44.38125000068279746, 47.55282581475767500 ) ) ;
#16222=CARTESIAN_POINT ( 'NONE',  ( 15.40903463028482356, 20.45937500034139589, 47.42413220539093999 ) ) ;
#16224=( BOUNDED_CURVE ( )  B_SPLINE_CURVE ( 2, ( #803, #2381, #11040, #13444, #9712, #6141, #2298, #6063, #7464, #12531, #5891, #14763, #12200 ),
 .UNSPECIFIED., .F., .T. ) 
 B_SPLINE_CURVE_WITH_KNOTS ( ( 3, 2, 2, 2, 2, 2, 3 ),
 ( 0.9166666666666667407, 0.9200000000000000400, 0.9266666666666666385, 0.9333333333333333481, 0.9399999999999999467, 0.9466666666666666563, 0.9500000000000000666 ),
 .UNSPECIFIED. ) 
 CURVE ( )  GEOMETRIC_REPRESENTATION_ITEM ( )  RATIONAL_B_SPLINE_CURVE ( ( 0.9755282581475768211, 0.9755282581475771542, 1.000000000000000000, 0.9510565162951535312, 1.000000000000000000, 0.9510565162951535312, 1.000000000000000000, 0.9510565162951535312, 1.000000000000000000, 0.9510565162951535312, 1.000000000000000000, 0.9755282581475763770, 0.9755282581475768211 ) ) 
 REPRESENTATION_ITEM ( '' )  );
#16229=CARTESIAN_POINT ( 'NONE',  ( 15.45084971874737789, 48.60000000000000142, 47.55282581475767500 ) ) ;
#16233=CARTESIAN_POINT ( 'NONE',  ( -3.111920190527341144E-15, 29.28125000068279604, -50.00000000000000000 ) ) ;
#16235=CARTESIAN_POINT ( 'NONE',  ( 30.81806926056964002, 20.62187500034139020, 42.41743335407647209 ) ) ;
#16236=CARTESIAN_POINT ( 'NONE',  ( -3.210462471511496205E-15, 31.35937500034138736, -52.43083105670540789 ) ) ;
#16238=CARTESIAN_POINT ( 'NONE',  ( -15.40903463028481646, 35.52187500034139589, -47.42413220539093999 ) ) ;
#16240=CARTESIAN_POINT ( 'NONE',  ( 15.40903463028481113, 41.25937500034139305, -47.42413220539094709 ) ) ;
#16242=CARTESIAN_POINT ( 'NONE',  ( -30.90169943749474868, 43.70000000000000284, -42.53254041760200721 ) ) ;
#16243=EDGE_LOOP ( 'NONE', ( #2317, #12066, #7721, #4061 ) ) ;
#16244=EDGE_CURVE ( 'NONE', #12025, #15727, #4480, .T. ) ;
#16248=CARTESIAN_POINT ( 'NONE',  ( -7.919222016226934890, 34.44874571845316069, 49.99999999999996447 ) ) ;
#16249=CARTESIAN_POINT ( 'NONE',  ( 49.99999999999999289, 40.88125000068279746, -16.24598481164532160 ) ) ;
#16250=CARTESIAN_POINT ( 'NONE',  ( -49.86468353124999453, 42.02187500034139589, 16.20201782572377525 ) ) ;
#16253=CARTESIAN_POINT ( 'NONE',  ( -49.99999999999999289, 27.68125000068279462, -16.24598481164531449 ) ) ;
#16254=ADVANCED_FACE ( 'NONE', ( #4347 ), #15643, .T. ) ;
#16255=CARTESIAN_POINT ( 'NONE',  ( -40.34137639590981905, 33.72187500034139873, -29.30972558990011478 ) ) ;
#16259=EDGE_CURVE ( 'NONE', #13440, #3318, #11188, .T. ) ;
#16262=( BOUNDED_CURVE ( )  B_SPLINE_CURVE ( 2, ( #10565, #4321, #3991, #13046, #10471, #11714, #1648, #2731, #8050, #6745, #15449, #11640, #14363 ),
 .UNSPECIFIED., .F., .F. ) 
 B_SPLINE_CURVE_WITH_KNOTS ( ( 3, 2, 2, 2, 2, 2, 3 ),
 ( 0.7833333333333333259, 0.7866666666666666252, 0.7933333333333333348, 0.8000000000000000444, 0.8066666666666666430, 0.8133333333333333526, 0.8166666666666666519 ),
 .UNSPECIFIED. ) 
 CURVE ( )  GEOMETRIC_REPRESENTATION_ITEM ( )  RATIONAL_B_SPLINE_CURVE ( ( 0.9755282581475768211, 0.9755282581475768211, 1.000000000000000000, 0.9510565162951535312, 1.000000000000000000, 0.9510565162951535312, 1.000000000000000000, 0.9510565162951535312, 1.000000000000000000, 0.9510565162951535312, 1.000000000000000000, 0.9755282581475768211, 0.9755282581475768211 ) ) 
 REPRESENTATION_ITEM ( '' )  );
#16263=CIRCLE ( 'NONE', #9365, 85.01963570546854498 ) ;
#16268=PLANE ( 'NONE',  #6548 ) ;
#16270=CARTESIAN_POINT ( 'NONE',  ( -40.34137639590981195, 36.05937500034139731, 29.30972558990012189 ) ) ;
#16271=CARTESIAN_POINT ( 'NONE',  ( 49.86468353125001585, 40.75937500034138594, 16.20201782572375038 ) ) ;
#16289=CARTESIAN_POINT ( 'NONE',  ( 0.000000000000000000, 20.00000000000000355, 50.00000000000000000 ) ) ;
#16290=CARTESIAN_POINT ( 'NONE',  ( 0.000000000000000000, 20.00000000000000355, 50.00000000000000000 ) ) ;
#16292=CARTESIAN_POINT ( 'NONE',  ( 2.600676159226421000E-13, 23.28125000068279604, -49.99999999999999289 ) ) ;
#16294=CARTESIAN_POINT ( 'NONE',  ( -3.111920190527341144E-15, 25.28125000068279604, -50.00000000000000000 ) ) ;
#16297=CARTESIAN_POINT ( 'NONE',  ( 30.90169943749474157, 49.08125000068280031, -42.53254041760200721 ) ) ;
#16298=CARTESIAN_POINT ( 'NONE',  ( 40.45084971874737789, 20.80000000000000426, 29.38926261462365375 ) ) ;
#16300=CARTESIAN_POINT ( 'NONE',  ( 15.40903463028482356, 22.45937500034139589, 47.42413220539093999 ) ) ;
#16306=CARTESIAN_POINT ( 'NONE',  ( 7.919222016226854954, 42.33250428222964246, 49.99999999999998579 ) ) ;
#16312=DIRECTION ( 'NONE',  ( -0.000000000000000000, 1.000000000000000000, -0.000000000000000000 ) ) ;
#16316=CARTESIAN_POINT ( 'NONE',  ( -30.81806926056963292, 23.62187500034139731, -42.41743335407647209 ) ) ;
#16317=CARTESIAN_POINT ( 'NONE',  ( 15.40903463028481113, 29.25937500034139660, -47.42413220539094709 ) ) ;
#16319=CARTESIAN_POINT ( 'NONE',  ( 49.86468353124999453, 35.02187500034139589, -16.20201782572376104 ) ) ;
#16321=CARTESIAN_POINT ( 'NONE',  ( -30.90169943749474868, 37.70000000000000995, -42.53254041760200721 ) ) ;
#16322=CARTESIAN_POINT ( 'NONE',  ( -49.86468353125000164, 37.85937500034139447, 0.000000000000000000 ) ) ;
#16324=CARTESIAN_POINT ( 'NONE',  ( 15.45084971874737789, 46.60000000000000142, 47.55282581475767500 ) ) ;
#16330=CARTESIAN_POINT ( 'NONE',  ( -49.99999999999999289, 34.10000000000000853, 16.24598481164533226 ) ) ;
#16333=CARTESIAN_POINT ( 'NONE',  ( 40.34137639590981195, 41.12187500034139731, -29.30972558990011834 ) ) ;
#16337=CARTESIAN_POINT ( 'NONE',  ( 40.45084971874737789, 24.58125000068280031, 29.38926261462365375 ) ) ;
#16338=CARTESIAN_POINT ( 'NONE',  ( -3.210462471511496205E-15, 35.42187500034140157, -52.43083105670540789 ) ) ;
#16350=DIRECTION ( 'NONE',  ( 0.000000000000000000, 1.000000000000000000, 0.000000000000000000 ) ) ;
#16352=CARTESIAN_POINT ( 'NONE',  ( 30.81806926056962936, 33.15937500034139873, -42.41743335407647209 ) ) ;
#16354=CARTESIAN_POINT ( 'NONE',  ( 30.81806926056964002, 48.62187500034139731, 42.41743335407646498 ) ) ;
#16358=CARTESIAN_POINT ( 'NONE',  ( -40.45084971874737789, 41.80000000000000426, -29.38926261462365730 ) ) ;
#16359=ORIENTED_EDGE ( 'NONE', *, *, #15755, .F. ) ;
#16360=( BOUNDED_CURVE ( )  B_SPLINE_CURVE ( 2, ( #13608, #973, #4747, #6069, #9882, #10296, #1381, #3970, #12780, #6563, #7711, #11293, #15261, #16354, #6224, #10210, #9120, #11529, #12862, #4994, #5152, #219, #12701, #2465, #15351, #3890, #15179, #1467, #5076, #1128, #10129, #48, #6391, #1215, #10049, #11453, #3729, #6472, #11621, #7547, #2551, #8962, #8789, #7872, #5322, #14018, #3809, #10374, #9043, #14181, #14098, #128, #2712, #15103, #15431, #2634, #13852, #8874, #4051, #12616, #7791, #5241, #7634, #2798, #6312, #11378, #16442, #1300, #13932, #2888, #7956, #15510, #14266, #11772, #13029, #11696, #9211, #11940, #4138, #4225, #1630, #463, #3043, #4306, #5565, #6648, #2966, #10626, #9371, #15679, #14420, #6726, #8113, #8032, #297, #374, #13192, #5394, #13107, #10546, #5476, #1797, #6889, #541, #15604, #12951, #9293, #14348, #1554, #10453, #1712, #6808, #11860, #7360, #11421, #13817, #2510, #10171, #4954, #12667, #4872, #14, #12746, #5116, #2429, #3527, #15221, #8673, #2599, #13981, #1265, #6113, #2262, #11183, #4792, #2353, #10014, #3851, #12502, #7435, #1016, #9848, #6356, #7675, #16238, #6270, #7506, #12577, #6187, #16319, #8579, #3772, #11342, #13894, #16409, #8916, #1175, #14900, #8754, #13654, #16161, #1343, #5041, #11101, #12425, #15069, #3698, #1095, #11261, #9928, #7589, #10095, #14982, #3611, #8831, #15144, #13740, #424, #9167, #2758, #15397, #9006, #12992, #1675, #7753, #7833, #15313, #1423, #13072, #3934, #4095, #14063, #14142, #7917, #12908, #2679, #6516, #6774, #12822, #14223, #11574, #10589, #4190, #14386, #14311, #1596, #2931, #10250, #5528, #11662, #181, #4017, #15645, #5285, #15561, #4270, #11818, #9256, #10336, #2849, #7998, #1518, #6608, #9086, #13151, #6690, #259, #91, #15474, #5195, #3007, #5364, #10420, #11738, #9335, #8077, #6434, #341, #11493, #5439, #10502, #10906, #7171, #13476, #12232, #3091, #14460, #2082, #4516, #9655, #835, #12060, #3336, #11983, #11907, #13387, #4432, #9413, #13311, #7004, #6859, #9749, #4678, #8407, #13237, #8168, #1835, #505, #9502, #663, #5925, #3175, #14548, #6931, #14794, #1910, #10667, #8322, #580, #5602, #5760, #10829, #15893, #15718, #15969, #1995, #4590, #7091, #10985, #12151, #4349, #9581, #5674, #10743, #14626, #3428, #753, #16049, #15802, #3252, #5841 ),
 .UNSPECIFIED., .F., .F. ) 
 B_SPLINE_CURVE_WITH_KNOTS ( ( 3, 2, 2, 2, 2, 2, 2, 2, 2, 2, 2, 2, 2, 2, 2, 2, 2, 2, 2, 2, 2, 2, 2, 2, 2, 2, 2, 2, 2, 2, 2, 2, 2, 2, 2, 2, 2, 2, 2, 2, 2, 2, 2, 2, 2, 2, 2, 2, 2, 2, 2, 2, 2, 2, 2, 2, 2, 2, 2, 2, 2, 2, 2, 2, 2, 2, 2, 2, 2, 2, 2, 2, 2, 2, 2, 2, 2, 2, 2, 2, 2, 2, 2, 2, 2, 2, 2, 2, 2, 2, 2, 2, 2, 2, 2, 2, 2, 2, 2, 2, 2, 2, 2, 2, 2, 2, 2, 2, 2, 2, 2, 2, 2, 2, 2, 2, 2, 2, 2, 2, 2, 2, 2, 2, 2, 2, 2, 2, 2, 2, 2, 2, 2, 2, 2, 2, 2, 2, 2, 2, 2, 2, 2, 2, 2, 2, 2, 2, 2, 2, 3 ),
 ( 0.000000000000000000, 0.006666666666666667095, 0.01333333333333333419, 0.02000000000000000042, 0.02666666666666666838, 0.03333333333333333287, 0.04000000000000000083, 0.04666666666666666879, 0.05333333333333333676, 0.05999999999999999778, 0.06666666666666666574, 0.07333333333333333370, 0.08000000000000000167, 0.08666666666666666963, 0.09333333333333333759, 0.1000000000000000056, 0.1066666666666666735, 0.1133333333333333276, 0.1199999999999999956, 0.1266666666666666774, 0.1333333333333333315, 0.1400000000000000133, 0.1466666666666666674, 0.1533333333333333215, 0.1600000000000000033, 0.1666666666666666574, 0.1733333333333333393, 0.1799999999999999933, 0.1866666666666666752, 0.1933333333333333293, 0.2000000000000000111, 0.2066666666666666652, 0.2133333333333333470, 0.2200000000000000011, 0.2266666666666666552, 0.2333333333333333370, 0.2399999999999999911, 0.2466666666666666730, 0.2533333333333333548, 0.2600000000000000089, 0.2666666666666666630, 0.2733333333333333171, 0.2800000000000000266, 0.2866666666666666807, 0.2933333333333333348, 0.2999999999999999889, 0.3066666666666666430, 0.3133333333333333526, 0.3200000000000000067, 0.3266666666666666607, 0.3333333333333333148, 0.3400000000000000244, 0.3466666666666666785, 0.3533333333333333326, 0.3599999999999999867, 0.3666666666666666408, 0.3733333333333333504, 0.3800000000000000044, 0.3866666666666666585, 0.3933333333333333126, 0.4000000000000000222, 0.4066666666666666763, 0.4133333333333333304, 0.4199999999999999845, 0.4266666666666666941, 0.4333333333333333481, 0.4400000000000000022, 0.4466666666666666563, 0.4533333333333333104, 0.4600000000000000200, 0.4666666666666666741, 0.4733333333333333282, 0.4799999999999999822, 0.4866666666666666918, 0.4933333333333333459, 0.5000000000000000000, 0.5066666666666667096, 0.5133333333333333082, 0.5200000000000000178, 0.5266666666666666163, 0.5333333333333333259, 0.5400000000000000355, 0.5466666666666666341, 0.5533333333333333437, 0.5600000000000000533, 0.5666666666666666519, 0.5733333333333333615, 0.5799999999999999600, 0.5866666666666666696, 0.5933333333333333792, 0.5999999999999999778, 0.6066666666666666874, 0.6133333333333332860, 0.6199999999999999956, 0.6266666666666667052, 0.6333333333333333037, 0.6400000000000000133, 0.6466666666666666119, 0.6533333333333333215, 0.6600000000000000311, 0.6666666666666666297, 0.6733333333333333393, 0.6800000000000000488, 0.6866666666666666474, 0.6933333333333333570, 0.6999999999999999556, 0.7066666666666666652, 0.7133333333333333748, 0.7199999999999999734, 0.7266666666666666829, 0.7333333333333332815, 0.7399999999999999911, 0.7466666666666667007, 0.7533333333333332993, 0.7600000000000000089, 0.7666666666666667185, 0.7733333333333333171, 0.7800000000000000266, 0.7866666666666666252, 0.7933333333333333348, 0.8000000000000000444, 0.8066666666666666430, 0.8133333333333333526, 0.8199999999999999512, 0.8266666666666666607, 0.8333333333333333703, 0.8399999999999999689, 0.8466666666666666785, 0.8533333333333333881, 0.8599999999999999867, 0.8666666666666666963, 0.8733333333333332948, 0.8800000000000000044, 0.8866666666666667140, 0.8933333333333333126, 0.9000000000000000222, 0.9066666666666666208, 0.9133333333333333304, 0.9200000000000000400, 0.9266666666666666385, 0.9333333333333333481, 0.9399999999999999467, 0.9466666666666666563, 0.9533333333333333659, 0.9599999999999999645, 0.9666666666666666741, 0.9733333333333333837, 0.9799999999999999822, 0.9866666666666666918, 0.9933333333333332904, 0.9973788038104776099 ),
 .UNSPECIFIED. ) 
 CURVE ( )  GEOMETRIC_REPRESENTATION_ITEM ( )  RATIONAL_B_SPLINE_CURVE ( ( 1.000000000000000000, 0.9510565162951535312, 1.000000000000000000, 0.9510565162951535312, 1.000000000000000000, 0.9510565162951535312, 1.000000000000000000, 0.9510565162951535312, 1.000000000000000000, 0.9510565162951535312, 1.000000000000000000, 0.9510565162951535312, 1.000000000000000000, 0.9510565162951535312, 1.000000000000000000, 0.9510565162951535312, 1.000000000000000000, 0.9510565162951535312, 1.000000000000000000, 0.9510565162951535312, 1.000000000000000000, 0.9510565162951535312, 1.000000000000000000, 0.9510565162951535312, 1.000000000000000000, 0.9510565162951535312, 1.000000000000000000, 0.9510565162951535312, 1.000000000000000000, 0.9510565162951535312, 1.000000000000000000, 0.9510565162951535312, 1.000000000000000000, 0.9510565162951535312, 1.000000000000000000, 0.9510565162951535312, 1.000000000000000000, 0.9510565162951535312, 1.000000000000000000, 0.9510565162951535312, 1.000000000000000000, 0.9510565162951535312, 1.000000000000000000, 0.9510565162951535312, 1.000000000000000000, 0.9510565162951535312, 1.000000000000000000, 0.9510565162951535312, 1.000000000000000000, 0.9510565162951535312, 1.000000000000000000, 0.9510565162951535312, 1.000000000000000000, 0.9510565162951535312, 1.000000000000000000, 0.9510565162951535312, 1.000000000000000000, 0.9510565162951535312, 1.000000000000000000, 0.9510565162951535312, 1.000000000000000000, 0.9510565162951535312, 1.000000000000000000, 0.9510565162951535312, 1.000000000000000000, 0.9510565162951535312, 1.000000000000000000, 0.9510565162951535312, 1.000000000000000000, 0.9510565162951535312, 1.000000000000000000, 0.9510565162951535312, 1.000000000000000000, 0.9510565162951535312, 1.000000000000000000, 0.9510565162951535312, 1.000000000000000000, 0.9510565162951535312, 1.000000000000000000, 0.9510565162951535312, 1.000000000000000000, 0.9510565162951535312, 1.000000000000000000, 0.9510565162951535312, 1.000000000000000000, 0.9510565162951535312, 1.000000000000000000, 0.9510565162951535312, 1.000000000000000000, 0.9510565162951535312, 1.000000000000000000, 0.9510565162951535312, 1.000000000000000000, 0.9510565162951535312, 1.000000000000000000, 0.9510565162951535312, 1.000000000000000000, 0.9510565162951535312, 1.000000000000000000, 0.9510565162951535312, 1.000000000000000000, 0.9510565162951535312, 1.000000000000000000, 0.9510565162951535312, 1.000000000000000000, 0.9510565162951535312, 1.000000000000000000, 0.9510565162951535312, 1.000000000000000000, 0.9510565162951535312, 1.000000000000000000, 0.9510565162951535312, 1.000000000000000000, 0.9510565162951535312, 1.000000000000000000, 0.9510565162951535312, 1.000000000000000000, 0.9510565162951535312, 1.000000000000000000, 0.9510565162951535312, 1.000000000000000000, 0.9510565162951535312, 1.000000000000000000, 0.9510565162951535312, 1.000000000000000000, 0.9510565162951535312, 1.000000000000000000, 0.9510565162951535312, 1.000000000000000000, 0.9510565162951535312, 1.000000000000000000, 0.9510565162951535312, 1.000000000000000000, 0.9510565162951535312, 1.000000000000000000, 0.9510565162951535312, 1.000000000000000000, 0.9510565162951535312, 1.000000000000000000, 0.9510565162951535312, 1.000000000000000000, 0.9510565162951535312, 1.000000000000000000, 0.9510565162951535312, 1.000000000000000000, 0.9510565162951535312, 1.000000000000000000, 0.9510565162951535312, 1.000000000000000000, 0.9510565162951535312, 1.000000000000000000, 0.9510565162951535312, 1.000000000000000000, 0.9510565162951535312, 1.000000000000000000, 0.9510565162951535312, 1.000000000000000000, 0.9510565162951535312, 1.000000000000000000, 0.9510565162951535312, 1.000000000000000000, 0.9510565162951535312, 1.000000000000000000, 0.9510565162951535312, 1.000000000000000000, 0.9510565162951535312, 1.000000000000000000, 0.9510565162951535312, 1.000000000000000000, 0.9510565162951535312, 1.000000000000000000, 0.9510565162951535312, 1.000000000000000000, 0.9510565162951535312, 1.000000000000000000, 0.9510565162951535312, 1.000000000000000000, 0.9510565162951535312, 1.000000000000000000, 0.9510565162951535312, 1.000000000000000000, 0.9510565162951535312, 1.000000000000000000, 0.9510565162951535312, 1.000000000000000000, 0.9510565162951535312, 1.000000000000000000, 0.9510565162951535312, 1.000000000000000000, 0.9510565162951535312, 1.000000000000000000, 0.9510565162951535312, 1.000000000000000000, 0.9510565162951535312, 1.000000000000000000, 0.9510565162951535312, 1.000000000000000000, 0.9510565162951535312, 1.000000000000000000, 0.9510565162951535312, 1.000000000000000000, 0.9510565162951535312, 1.000000000000000000, 0.9510565162951535312, 1.000000000000000000, 0.9510565162951535312, 1.000000000000000000, 0.9510565162951535312, 1.000000000000000000, 0.9510565162951535312, 1.000000000000000000, 0.9510565162951535312, 1.000000000000000000, 0.9510565162951535312, 1.000000000000000000, 0.9510565162951535312, 1.000000000000000000, 0.9510565162951535312, 1.000000000000000000, 0.9510565162951535312, 1.000000000000000000, 0.9510565162951535312, 1.000000000000000000, 0.9510565162951535312, 1.000000000000000000, 0.9510565162951535312, 1.000000000000000000, 0.9510565162951535312, 1.000000000000000000, 0.9510565162951535312, 1.000000000000000000, 0.9510565162951535312, 1.000000000000000000, 0.9510565162951535312, 1.000000000000000000, 0.9510565162951535312, 1.000000000000000000, 0.9510565162951535312, 1.000000000000000000, 0.9510565162951535312, 1.000000000000000000, 0.9510565162951535312, 1.000000000000000000, 0.9510565162951535312, 1.000000000000000000, 0.9510565162951535312, 1.000000000000000000, 0.9510565162951535312, 1.000000000000000000, 0.9510565162951535312, 1.000000000000000000, 0.9510565162951535312, 1.000000000000000000, 0.9510565162951535312, 1.000000000000000000, 0.9510565162951535312, 1.000000000000000000, 0.9510565162951535312, 1.000000000000000000, 0.9510565162951535312, 1.000000000000000000, 0.9510565162951535312, 1.000000000000000000, 0.9510565162951535312, 1.000000000000000000, 0.9510565162951535312, 1.000000000000000000, 0.9510565162951535312, 1.000000000000000000, 0.9510565162951535312, 1.000000000000000000, 0.9510565162951535312, 1.000000000000000000, 0.9510565162951535312, 1.000000000000000000, 0.9510565162951535312, 1.000000000000000000, 0.9510565162951535312, 1.000000000000000000, 0.9510565162951535312, 1.000000000000000000, 0.9510565162951535312, 1.000000000000000000, 0.9510565162951535312, 1.000000000000000000, 0.9510565162951535312, 1.000000000000000000, 0.9510565162951535312, 1.000000000000000000, 0.9510565162951535312, 1.000000000000000000, 0.9510565162951535312, 1.000000000000000000, 0.9510565162951535312, 1.000000000000000000, 0.9510565162951535312, 1.000000000000000000, 0.9510565162951535312, 1.000000000000000000, 0.9703000872435175728, 0.9766452105560685659 ) ) 
 REPRESENTATION_ITEM ( '' )  );
#16361=EDGE_CURVE ( 'NONE', #16417, #15116, #3202, .T. ) ;
#16377=CYLINDRICAL_SURFACE ( 'NONE', #5844, 50.00000000000000000 ) ;
#16380=CARTESIAN_POINT ( 'NONE',  ( -1.175978673139307859E-14, 45.07596123493892293, -92.05189185291139609 ) ) ;
#16383=EDGE_CURVE ( 'NONE', #6101, #102, #5923, .T. ) ;
#16385=CARTESIAN_POINT ( 'NONE',  ( 15.45084971874737789, 48.38125000068280457, 47.55282581475767500 ) ) ;
#16386=CARTESIAN_POINT ( 'NONE',  ( 15.45084971874737789, 20.60000000000000142, 47.55282581475767500 ) ) ;
#16389=CARTESIAN_POINT ( 'NONE',  ( 9.631387414534489405E-15, 20.35937500034139092, 52.43083105670540789 ) ) ;
#16390=CARTESIAN_POINT ( 'NONE',  ( -49.99999999999999289, 41.88125000068279746, 16.24598481164533226 ) ) ;
#16401=CARTESIAN_POINT ( 'NONE',  ( -0.5757193964092639504, 40.00000000000000000, 92.94692077166138233 ) ) ;
#16405=CARTESIAN_POINT ( 'NONE',  ( 15.40903463028482356, 22.52187500034139589, 47.42413220539093999 ) ) ;
#16406=CARTESIAN_POINT ( 'NONE',  ( -49.86468353124999453, 23.95937500034138878, 16.20201782572377169 ) ) ;
#16409=CARTESIAN_POINT ( 'NONE',  ( 15.40903463028482356, 34.52187500034140299, 47.42413220539093999 ) ) ;
#16411=CARTESIAN_POINT ( 'NONE',  ( 15.45084971874737789, 32.60000000000000142, 47.55282581475767500 ) ) ;
#16412=CARTESIAN_POINT ( 'NONE',  ( 30.81806926056962936, 41.15937500034139873, -42.41743335407647209 ) ) ;
#16414=CARTESIAN_POINT ( 'NONE',  ( -30.90169943749473802, 48.30000000000000426, 42.53254041760200721 ) ) ;
#16417=VERTEX_POINT ( 'NONE', #4588 ) ;
#16421=CARTESIAN_POINT ( 'NONE',  ( -7.919222016226688865, 33.55125428154685352, -50.00000000000003553 ) ) ;
#16424=CARTESIAN_POINT ( 'NONE',  ( -40.34137639590981195, 42.12187500034139731, 29.30972558990012189 ) ) ;
#16429=CARTESIAN_POINT ( 'NONE',  ( -49.99999999999999289, 29.68125000068279817, -16.24598481164531449 ) ) ;
#16431=CARTESIAN_POINT ( 'NONE',  ( -30.81806926056962226, 34.22187500034139873, 42.41743335407647919 ) ) ;
#16434=CARTESIAN_POINT ( 'NONE',  ( -40.45084971874737079, 28.20000000000000284, 29.38926261462367151 ) ) ;
#16440=CARTESIAN_POINT ( 'NONE',  ( 49.86468353125000164, 28.85937500034139802, -6.106662507704105588E-15 ) ) ;
#16441=DIRECTION ( 'NONE',  ( -0.000000000000000000, 1.000000000000000000, -0.000000000000000000 ) ) ;
#16442=CARTESIAN_POINT ( 'NONE',  ( 15.40903463028481113, 43.32187500034139305, -47.42413220539094709 ) ) ;
#16447=CARTESIAN_POINT ( 'NONE',  ( -49.99999999999999289, 42.09999999999999432, 16.24598481164533226 ) ) ;
#16457=LINE ( 'NONE', #10224, #12743 ) ;
#16458=CARTESIAN_POINT ( 'NONE',  ( 0.000000000000000000, 20.00000000000000355, 0.000000000000000000 ) ) ;
#16459=CARTESIAN_POINT ( 'NONE',  ( 49.99999999999999289, 32.88125000068280457, -16.24598481164532160 ) ) ;
ENDSEC;
END-ISO-10303-21;
